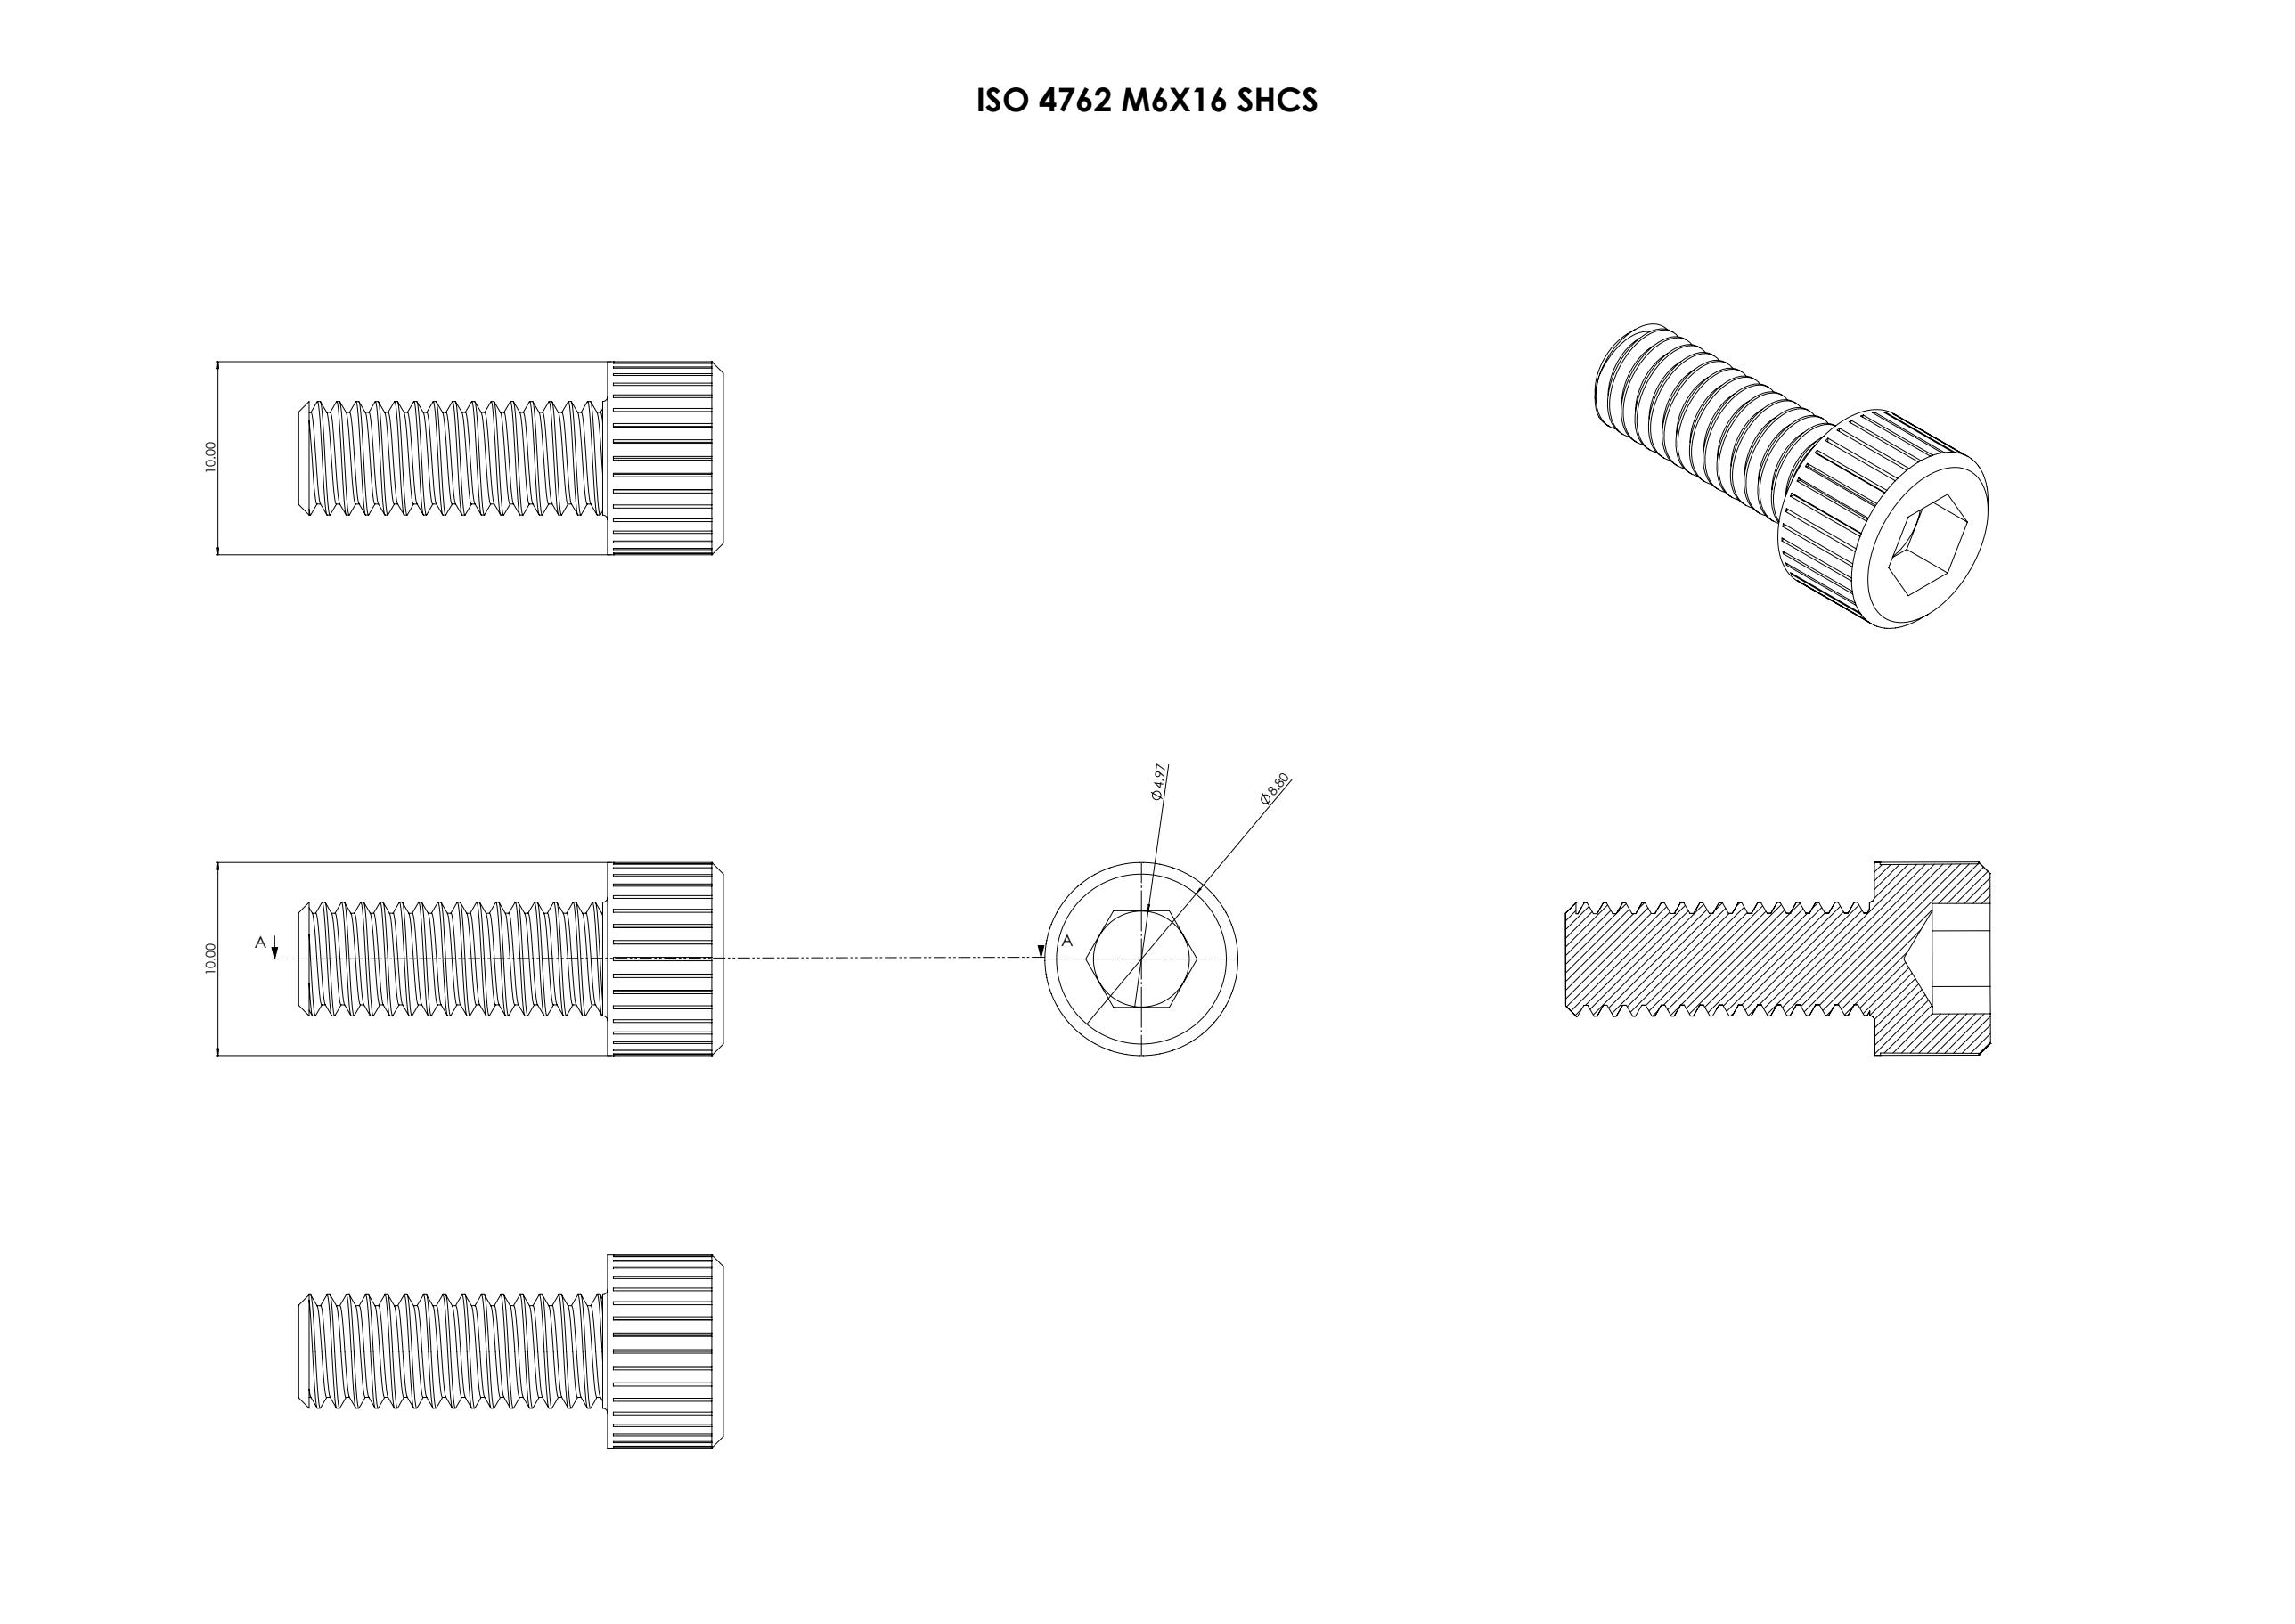
ISO-10303-21;
HEADER;
/* Generated by software containing ST-Developer
 * from STEP Tools, Inc. (www.steptools.com) 
 */

FILE_DESCRIPTION(
/* description */ (''),
/* implementation_level */ '2;1');

FILE_NAME(
/* name */ '09_ISO_4762_M6x16_SHCS.step',
/* time_stamp */ '2026-10-11T08:27:52-07:00',
/* author */ (''),
/* organization */ (''),
/* preprocessor_version */ 'ST-DEVELOPER v20.2',
/* originating_system */ 'Autodesk Translation Framework v15.15.0.0',
/* authorisation */ '');

FILE_SCHEMA (('AUTOMOTIVE_DESIGN { 1 0 10303 214 3 1 1 }'));
ENDSEC;

DATA;
#10=MECHANICAL_DESIGN_GEOMETRIC_PRESENTATION_REPRESENTATION('',(#927),#94301);
#550=B_SPLINE_CURVE_WITH_KNOTS('',3,(#87482,#87483,#87484,#87485,#87486,
#87487,#87488,#87489,#87490,#87491),.UNSPECIFIED.,.F.,.F.,(4,3,3,4),(-4.09293042013066,
-3.98462531944883,-2.98846898958662,-2.06863817490914),.UNSPECIFIED.);
#551=B_SPLINE_CURVE_WITH_KNOTS('',3,(#87494,#87495,#87496,#87497,#87498,
#87499,#87500),.UNSPECIFIED.,.F.,.F.,(4,3,4),(0.,0.996156329862199,1.11730040836818),
 .UNSPECIFIED.);
#552=B_SPLINE_CURVE_WITH_KNOTS('',3,(#87505,#87506,#87507,#87508,#87509,
#87510,#87511,#87512,#87513,#87514,#87515,#87516,#87517,#87518,#87519,#87520,
#87521,#87522,#87523,#87524,#87525,#87526),.UNSPECIFIED.,.F.,.F.,(4,3,3,
3,3,3,3,4),(-10.3761157273103,-9.96156329862207,-8.96540696875986,-7.96925063889766,
-6.97309430903545,-5.97693797917324,-4.98078164931104,-4.09293042013066),
 .UNSPECIFIED.);
#553=B_SPLINE_CURVE_WITH_KNOTS('',3,(#87527,#87528,#87529,#87530,#87531,
#87532,#87533,#87534,#87535,#87536,#87537,#87538,#87539,#87540,#87541,#87542,
#87543,#87544,#87545,#87546,#87547,#87548),.UNSPECIFIED.,.F.,.F.,(4,3,3,
3,3,3,3,4),(1.11730040836818,1.99231265972441,2.98846898958662,3.98462531944883,
4.98078164931103,5.97693797917324,6.97309430903544,7.40048571554775),
 .UNSPECIFIED.);
#554=B_SPLINE_CURVE_WITH_KNOTS('',3,(#87553,#87554,#87555,#87556,#87557,
#87558,#87559,#87560,#87561,#87562,#87563,#87564,#87565,#87566,#87567,#87568,
#87569,#87570,#87571,#87572,#87573,#87574),.UNSPECIFIED.,.F.,.F.,(4,3,3,
3,3,3,3,4),(-16.6593010344898,-15.9385012777953,-14.9423449479331,-13.9461886180709,
-12.9500322882087,-11.9538759583465,-10.9577196284843,-10.3761157273103),
 .UNSPECIFIED.);
#555=B_SPLINE_CURVE_WITH_KNOTS('',3,(#87575,#87576,#87577,#87578,#87579,
#87580,#87581,#87582,#87583,#87584,#87585,#87586,#87587,#87588,#87589,#87590,
#87591,#87592,#87593,#87594,#87595,#87596),.UNSPECIFIED.,.F.,.F.,(4,3,3,
3,3,3,3,4),(7.40048571554775,7.96925063889765,8.96540696875986,9.96156329862207,
10.9577196284843,11.9538759583465,12.9500322882087,13.6836710227273),
 .UNSPECIFIED.);
#556=B_SPLINE_CURVE_WITH_KNOTS('',3,(#87601,#87602,#87603,#87604,#87605,
#87606,#87607,#87608,#87609,#87610,#87611,#87612,#87613,#87614,#87615,#87616,
#87617,#87618,#87619,#87620,#87621,#87622,#87623,#87624,#87625),
 .UNSPECIFIED.,.F.,.F.,(4,3,3,3,3,3,3,3,4),(-22.9424863416694,-22.9115955868308,
-21.9154392569686,-20.9192829271063,-19.9231265972441,-18.9269702673819,
-17.9308139375197,-16.9346576076575,-16.6593010344898),.UNSPECIFIED.);
#557=B_SPLINE_CURVE_WITH_KNOTS('',3,(#87626,#87627,#87628,#87629,#87630,
#87631,#87632,#87633,#87634,#87635,#87636,#87637,#87638,#87639,#87640,#87641,
#87642,#87643,#87644,#87645,#87646,#87647,#87648,#87649,#87650),
 .UNSPECIFIED.,.F.,.F.,(4,3,3,3,3,3,3,3,4),(13.6836710227273,13.9461886180709,
14.9423449479331,15.9385012777953,16.9346576076575,17.9308139375197,18.9269702673819,
19.9231265972441,19.9668563299069),.UNSPECIFIED.);
#558=B_SPLINE_CURVE_WITH_KNOTS('',3,(#87655,#87656,#87657,#87658,#87659,
#87660,#87661,#87662,#87663,#87664,#87665,#87666,#87667,#87668,#87669,#87670,
#87671,#87672,#87673,#87674,#87675,#87676),.UNSPECIFIED.,.F.,.F.,(4,3,3,
3,3,3,3,4),(-29.225671648849,-28.888533566004,-27.8923772361418,-26.8962209062796,
-25.9000645764174,-24.9039082465552,-23.907751916693,-22.9424863416694),
 .UNSPECIFIED.);
#559=B_SPLINE_CURVE_WITH_KNOTS('',3,(#87677,#87678,#87679,#87680,#87681,
#87682,#87683,#87684,#87685,#87686,#87687,#87688,#87689,#87690,#87691,#87692,
#87693,#87694,#87695,#87696,#87697,#87698),.UNSPECIFIED.,.F.,.F.,(4,3,3,
3,3,3,3,4),(19.9668563299069,20.9192829271063,21.9154392569685,22.9115955868307,
23.907751916693,24.9039082465552,25.9000645764174,26.2500416370865),
 .UNSPECIFIED.);
#560=B_SPLINE_CURVE_WITH_KNOTS('',3,(#87703,#87704,#87705,#87706,#87707,
#87708,#87709,#87710,#87711,#87712,#87713,#87714,#87715,#87716,#87717,#87718,
#87719,#87720,#87721,#87722,#87723,#87724),.UNSPECIFIED.,.F.,.F.,(4,3,3,
3,3,3,3,4),(-35.5088569560286,-34.8654715451772,-33.869315215315,-32.8731588854528,
-31.8770025555906,-30.8808462257284,-29.8846898958662,-29.225671648849),
 .UNSPECIFIED.);
#561=B_SPLINE_CURVE_WITH_KNOTS('',3,(#87725,#87726,#87727,#87728,#87729,
#87730,#87731,#87732,#87733,#87734,#87735,#87736,#87737,#87738,#87739,#87740,
#87741,#87742,#87743,#87744,#87745,#87746),.UNSPECIFIED.,.F.,.F.,(4,3,3,
3,3,3,3,4),(26.2500416370865,26.8962209062796,27.8923772361418,28.888533566004,
29.8846898958662,30.8808462257284,31.8770025555906,32.5332269442661),
 .UNSPECIFIED.);
#562=B_SPLINE_CURVE_WITH_KNOTS('',3,(#87751,#87752,#87753,#87754,#87755,
#87756,#87757,#87758,#87759,#87760,#87761,#87762,#87763,#87764,#87765,#87766,
#87767,#87768,#87769,#87770,#87771,#87772),.UNSPECIFIED.,.F.,.F.,(4,3,3,
3,3,3,3,4),(-41.7920422632082,-40.8424095243505,-39.8462531944883,-38.8500968646261,
-37.8539405347639,-36.8577842049017,-35.8616278750394,-35.5088569560286),
 .UNSPECIFIED.);
#563=B_SPLINE_CURVE_WITH_KNOTS('',3,(#87773,#87774,#87775,#87776,#87777,
#87778,#87779,#87780,#87781,#87782,#87783,#87784,#87785,#87786,#87787,#87788,
#87789,#87790,#87791,#87792,#87793,#87794),.UNSPECIFIED.,.F.,.F.,(4,3,3,
3,3,3,3,4),(32.5332269442661,32.8731588854528,33.869315215315,34.8654715451772,
35.8616278750394,36.8577842049016,37.8539405347639,38.8164122514457),
 .UNSPECIFIED.);
#564=B_SPLINE_CURVE_WITH_KNOTS('',3,(#87799,#87800,#87801,#87802,#87803,
#87804,#87805,#87806,#87807,#87808,#87809,#87810,#87811,#87812,#87813,#87814,
#87815,#87816,#87817,#87818,#87819,#87820,#87821,#87822,#87823),
 .UNSPECIFIED.,.F.,.F.,(4,3,3,3,3,3,3,3,4),(-48.0752275703878,-47.8155038333859,
-46.8193475035237,-45.8231911736615,-44.8270348437993,-43.8308785139371,
-42.8347221840749,-41.8385658542127,-41.7920422632082),.UNSPECIFIED.);
#565=B_SPLINE_CURVE_WITH_KNOTS('',3,(#87824,#87825,#87826,#87827,#87828,
#87829,#87830,#87831,#87832,#87833,#87834,#87835,#87836,#87837,#87838,#87839,
#87840,#87841,#87842,#87843,#87844,#87845,#87846,#87847,#87848),
 .UNSPECIFIED.,.F.,.F.,(4,3,3,3,3,3,3,3,4),(38.8164122514457,38.8500968646261,
39.8462531944883,40.8424095243505,41.8385658542127,42.8347221840749,43.8308785139371,
44.8270348437993,45.0995975586253),.UNSPECIFIED.);
#566=B_SPLINE_CURVE_WITH_KNOTS('',3,(#87853,#87854,#87855,#87856,#87857,
#87858,#87859,#87860,#87861,#87862,#87863,#87864,#87865,#87866,#87867,#87868,
#87869,#87870,#87871,#87872,#87873,#87874),.UNSPECIFIED.,.F.,.F.,(4,3,3,
3,3,3,3,4),(-54.3584128775674,-53.7924418125592,-52.796285482697,-51.8001291528348,
-50.8039728229726,-49.8078164931104,-48.8116601632481,-48.0752275703878),
 .UNSPECIFIED.);
#567=B_SPLINE_CURVE_WITH_KNOTS('',3,(#87875,#87876,#87877,#87878,#87879,
#87880,#87881,#87882,#87883,#87884,#87885,#87886,#87887,#87888,#87889,#87890,
#87891,#87892,#87893,#87894,#87895,#87896),.UNSPECIFIED.,.F.,.F.,(4,3,3,
3,3,3,3,4),(45.0995975586253,45.8231911736615,46.8193475035237,47.8155038333859,
48.8116601632481,49.8078164931103,50.8039728229725,51.3827828658049),
 .UNSPECIFIED.);
#568=B_SPLINE_CURVE_WITH_KNOTS('',3,(#87901,#87902,#87903,#87904,#87905,
#87906,#87907,#87908,#87909,#87910,#87911,#87912,#87913,#87914,#87915,#87916,
#87917,#87918,#87919,#87920,#87921,#87922),.UNSPECIFIED.,.F.,.F.,(4,3,3,
3,3,3,3,4),(-60.641598184747,-59.7693797917324,-58.7732234618702,-57.777067132008,
-56.7809108021458,-55.7847544722836,-54.7885981424214,-54.3584128775674),
 .UNSPECIFIED.);
#569=B_SPLINE_CURVE_WITH_KNOTS('',3,(#87923,#87924,#87925,#87926,#87927,
#87928,#87929,#87930,#87931,#87932,#87933,#87934,#87935,#87936,#87937,#87938,
#87939,#87940,#87941,#87942,#87943,#87944),.UNSPECIFIED.,.F.,.F.,(4,3,3,
3,3,3,3,4),(51.3827828658049,51.8001291528347,52.796285482697,53.7924418125592,
54.7885981424214,55.7847544722836,56.7809108021458,57.6659681729845),
 .UNSPECIFIED.);
#570=B_SPLINE_CURVE_WITH_KNOTS('',3,(#87949,#87950,#87951,#87952,#87953,
#87954,#87955,#87956,#87957,#87958,#87959,#87960,#87961,#87962,#87963,#87964,
#87965,#87966,#87967,#87968,#87969,#87970,#87971,#87972,#87973),
 .UNSPECIFIED.,.F.,.F.,(4,3,3,3,3,3,3,3,4),(-66.9247834919266,-66.7424741007679,
-65.7463177709057,-64.7501614410435,-63.7540051111813,-62.757848781319,
-61.7616924514568,-60.7655361215946,-60.641598184747),.UNSPECIFIED.);
#571=B_SPLINE_CURVE_WITH_KNOTS('',3,(#87974,#87975,#87976,#87977,#87978,
#87979,#87980,#87981,#87982,#87983,#87984,#87985,#87986,#87987,#87988,#87989,
#87990,#87991,#87992,#87993,#87994,#87995,#87996,#87997,#87998),
 .UNSPECIFIED.,.F.,.F.,(4,3,3,3,3,3,3,3,4),(57.6659681729845,57.777067132008,
58.7732234618702,59.7693797917324,60.7655361215946,61.7616924514568,62.757848781319,
63.7540051111813,63.9491534801641),.UNSPECIFIED.);
#572=B_SPLINE_CURVE_WITH_KNOTS('',3,(#88003,#88004,#88005,#88006,#88007,
#88008,#88009,#88010,#88011,#88012,#88013,#88014,#88015,#88016,#88017,#88018,
#88019,#88020,#88021,#88022,#88023,#88024),.UNSPECIFIED.,.F.,.F.,(4,3,3,
3,3,3,3,4),(-73.2079687991062,-72.7194120799411,-71.7232557500789,-70.7270994202167,
-69.7309430903545,-68.7347867604923,-67.7386304306301,-66.9247834919266),
 .UNSPECIFIED.);
#573=B_SPLINE_CURVE_WITH_KNOTS('',3,(#88025,#88026,#88027,#88028,#88029,
#88030,#88031,#88032,#88033,#88034,#88035,#88036,#88037,#88038,#88039,#88040,
#88041,#88042,#88043,#88044,#88045,#88046),.UNSPECIFIED.,.F.,.F.,(4,3,3,
3,3,3,3,4),(63.9491534801641,64.7501614410435,65.7463177709057,66.7424741007679,
67.7386304306301,68.7347867604923,69.7309430903545,70.2323387873437),
 .UNSPECIFIED.);
#574=B_SPLINE_CURVE_WITH_KNOTS('',3,(#88051,#88052,#88053,#88054,#88055,
#88056,#88057,#88058,#88059,#88060,#88061,#88062,#88063,#88064,#88065,#88066,
#88067,#88068,#88069,#88070,#88071,#88072),.UNSPECIFIED.,.F.,.F.,(4,3,3,
3,3,3,3,4),(-79.4911541062857,-78.6963500591144,-77.7001937292521,-76.7040373993899,
-75.7078810695277,-74.7117247396655,-73.7155684098033,-73.2079687991062),
 .UNSPECIFIED.);
#575=B_SPLINE_CURVE_WITH_KNOTS('',3,(#88073,#88074,#88075,#88076,#88077,
#88078,#88079,#88080,#88081,#88082,#88083,#88084,#88085,#88086,#88087,#88088,
#88089,#88090,#88091,#88092,#88093,#88094),.UNSPECIFIED.,.F.,.F.,(4,3,3,
3,3,3,3,4),(70.2323387873437,70.7270994202167,71.7232557500789,72.7194120799411,
73.7155684098033,74.7117247396655,75.7078810695277,76.5155240945233),
 .UNSPECIFIED.);
#576=B_SPLINE_CURVE_WITH_KNOTS('',3,(#88099,#88100,#88101,#88102,#88103,
#88104,#88105,#88106,#88107,#88108,#88109,#88110,#88111,#88112,#88113,#88114,
#88115,#88116,#88117,#88118,#88119,#88120,#88121,#88122,#88123),
 .UNSPECIFIED.,.F.,.F.,(4,3,3,3,3,3,3,3,4),(-85.7743394134653,-85.6694443681498,
-84.6732880382876,-83.6771317084254,-82.6809753785632,-81.684819048701,
-80.6886627188388,-79.6925063889766,-79.4911541062857),.UNSPECIFIED.);
#577=B_SPLINE_CURVE_WITH_KNOTS('',3,(#88124,#88125,#88126,#88127,#88128,
#88129,#88130,#88131,#88132,#88133,#88134,#88135,#88136,#88137,#88138,#88139,
#88140,#88141,#88142,#88143,#88144,#88145,#88146,#88147,#88148),
 .UNSPECIFIED.,.F.,.F.,(4,3,3,3,3,3,3,3,4),(76.5155240945233,76.7040373993899,
77.7001937292521,78.6963500591143,79.6925063889765,80.6886627188388,81.684819048701,
82.6809753785631,82.7987094017029),.UNSPECIFIED.);
#578=B_SPLINE_CURVE_WITH_KNOTS('',3,(#88153,#88154,#88155,#88156,#88157,
#88158,#88159,#88160,#88161,#88162,#88163,#88164,#88165,#88166,#88167,#88168,
#88169,#88170,#88171,#88172,#88173,#88174),.UNSPECIFIED.,.F.,.F.,(4,3,3,
3,3,3,3,4),(-92.0575247206449,-91.646382347323,-90.6502260174608,-89.6540696875986,
-88.6579133577364,-87.6617570278742,-86.665600698012,-85.7743394134653),
 .UNSPECIFIED.);
#579=B_SPLINE_CURVE_WITH_KNOTS('',3,(#88175,#88176,#88177,#88178,#88179,
#88180,#88181,#88182,#88183,#88184,#88185,#88186,#88187,#88188,#88189,#88190,
#88191,#88192,#88193,#88194,#88195,#88196),.UNSPECIFIED.,.F.,.F.,(4,3,3,
3,3,3,3,4),(82.7987094017029,83.6771317084254,84.6732880382876,85.6694443681498,
86.665600698012,87.6617570278742,88.6579133577364,89.0818947088824),
 .UNSPECIFIED.);
#580=B_SPLINE_CURVE_WITH_KNOTS('',3,(#88203,#88204,#88205,#88206,#88207,
#88208,#88209,#88210,#88211,#88212,#88213,#88214,#88215,#88216,#88217,#88218,
#88219,#88220,#88221),.UNSPECIFIED.,.F.,.F.,(4,3,3,3,3,3,4),(-97.6233203264963,
-96.6271639966341,-95.6310076667719,-94.6348513369097,-93.6386950070474,
-92.6425386771852,-92.0575247206449),.UNSPECIFIED.);
#581=B_SPLINE_CURVE_WITH_KNOTS('',3,(#88222,#88223,#88224,#88225,#88226,
#88227,#88228,#88229,#88230,#88231,#88232,#88233,#88234,#88235,#88236,#88237,
#88238,#88239,#88240,#88241,#88242,#88243),.UNSPECIFIED.,.F.,.F.,(4,3,3,
3,3,3,3,4),(89.0818947088824,89.6540696875986,90.6502260174608,91.646382347323,
92.6425386771852,93.6386950070475,94.6348513369096,95.365080016062),
 .UNSPECIFIED.);
#582=B_SPLINE_CURVE_WITH_KNOTS('',3,(#88249,#88250,#88251,#88252,#88253,
#88254,#88255),.UNSPECIFIED.,.F.,.F.,(4,1,1,1,4),(103.672557568463,104.257571525003,
105.253727854866,106.249884184728,107.169714999405),.UNSPECIFIED.);
#583=B_SPLINE_CURVE_WITH_KNOTS('',3,(#88258,#88259,#88260,#88261,#88262,
#88263),.UNSPECIFIED.,.F.,.F.,(4,1,1,4),(103.672557568463,103.938485219173,
104.934641549035,105.930797878897),.UNSPECIFIED.);
#584=B_SPLINE_CURVE_WITH_KNOTS('',3,(#88268,#88269,#88270,#88271,#88272,
#88273,#88274,#88275,#88276,#88277),.UNSPECIFIED.,.F.,.F.,(4,1,1,1,1,1,
1,4),(97.3893722612836,98.2806335458302,99.2767898756924,100.272946205555,
101.269102535417,102.265258865279,103.261415195141,103.672557568463),
 .UNSPECIFIED.);
#585=B_SPLINE_CURVE_WITH_KNOTS('',3,(#88278,#88279,#88280,#88281,#88282,
#88283,#88284,#88285,#88286,#88287),.UNSPECIFIED.,.F.,.F.,(4,1,1,1,1,1,
1,4),(97.3893722612836,97.9615472399996,98.9577035698618,99.9538598997241,
100.950016229586,101.946172559448,102.942328889311,103.672557568463),
 .UNSPECIFIED.);
#586=B_SPLINE_CURVE_WITH_KNOTS('',3,(#88292,#88293,#88294,#88295,#88296,
#88297,#88298,#88299,#88300,#88301,#88302),.UNSPECIFIED.,.F.,.F.,(4,1,1,
1,1,1,1,1,4),(91.106186954104,91.3075392367948,92.303695566657,93.2998518965192,
94.2960082263814,95.2921645562436,96.2883208861058,97.284477215968,97.3893722612836),
 .UNSPECIFIED.);
#587=B_SPLINE_CURVE_WITH_KNOTS('',3,(#88303,#88304,#88305,#88306,#88307,
#88308,#88309,#88310,#88311,#88312),.UNSPECIFIED.,.F.,.F.,(4,1,1,1,1,1,
1,4),(91.106186954104,91.9846092608264,92.9807655906886,93.9769219205508,
94.973078250413,95.9692345802752,96.9653909101374,97.3893722612836),
 .UNSPECIFIED.);
#588=B_SPLINE_CURVE_WITH_KNOTS('',3,(#88317,#88318,#88319,#88320,#88321,
#88322,#88323,#88324,#88325,#88326),.UNSPECIFIED.,.F.,.F.,(4,1,1,1,1,1,
1,4),(84.8230016469244,85.3306012576215,86.3267575874837,87.322913917346,
88.3190702472082,89.3152265770704,90.3113829069326,91.106186954104),
 .UNSPECIFIED.);
#589=B_SPLINE_CURVE_WITH_KNOTS('',3,(#88327,#88328,#88329,#88330,#88331,
#88332,#88333,#88334,#88335,#88336,#88337),.UNSPECIFIED.,.F.,.F.,(4,1,1,
1,1,1,1,1,4),(84.8230016469244,85.0115149517909,86.0076712816532,87.0038276115154,
87.9999839413776,88.9961402712398,89.992296601102,90.9884529309642,91.106186954104),
 .UNSPECIFIED.);
#590=B_SPLINE_CURVE_WITH_KNOTS('',3,(#88342,#88343,#88344,#88345,#88346,
#88347,#88348,#88349,#88350,#88351),.UNSPECIFIED.,.F.,.F.,(4,1,1,1,1,1,
1,4),(78.5398163397448,79.3536632784483,80.3498196083105,81.3459759381727,
82.3421322680349,83.3382885978971,84.3344449277593,84.8230016469244),
 .UNSPECIFIED.);
#591=B_SPLINE_CURVE_WITH_KNOTS('',3,(#88352,#88353,#88354,#88355,#88356,
#88357,#88358,#88359,#88360,#88361),.UNSPECIFIED.,.F.,.F.,(4,1,1,1,1,1,
1,4),(78.5398163397448,79.0345769726177,80.0307333024799,81.0268896323421,
82.0230459622043,83.0192022920665,84.0153586219287,84.8230016469244),
 .UNSPECIFIED.);
#592=B_SPLINE_CURVE_WITH_KNOTS('',3,(#88366,#88367,#88368,#88369,#88370,
#88371,#88372,#88373,#88374,#88375,#88376),.UNSPECIFIED.,.F.,.F.,(4,1,1,
1,1,1,1,1,4),(72.2566310325652,72.3805689694128,73.3767252992751,74.3728816291373,
75.3690379589995,76.3651942888617,77.3613506187239,78.3575069485861,78.5398163397448),
 .UNSPECIFIED.);
#593=B_SPLINE_CURVE_WITH_KNOTS('',3,(#88377,#88378,#88379,#88380,#88381,
#88382,#88383,#88384,#88385,#88386),.UNSPECIFIED.,.F.,.F.,(4,1,1,1,1,1,
1,4),(72.2566310325652,73.0576389934445,74.0537953233067,75.0499516531689,
76.0461079830311,77.0422643128933,78.0384206427555,78.5398163397448),
 .UNSPECIFIED.);
#594=B_SPLINE_CURVE_WITH_KNOTS('',3,(#88391,#88392,#88393,#88394,#88395,
#88396,#88397,#88398,#88399,#88400),.UNSPECIFIED.,.F.,.F.,(4,1,1,1,1,1,
1,4),(65.9734457253856,66.4036309902396,67.3997873201018,68.395943649964,
69.3920999798262,70.3882563096884,71.3844126395506,72.2566310325652),
 .UNSPECIFIED.);
#595=B_SPLINE_CURVE_WITH_KNOTS('',3,(#88401,#88402,#88403,#88404,#88405,
#88406,#88407,#88408,#88409,#88410,#88411),.UNSPECIFIED.,.F.,.F.,(4,1,1,
1,1,1,1,1,4),(65.9734457253856,66.084544684409,67.0807010142712,68.0768573441334,
69.0730136739956,70.0691700038578,71.0653263337201,72.0614826635823,72.2566310325652),
 .UNSPECIFIED.);
#596=B_SPLINE_CURVE_WITH_KNOTS('',3,(#88416,#88417,#88418,#88419,#88420,
#88421,#88422,#88423,#88424,#88425),.UNSPECIFIED.,.F.,.F.,(4,1,1,1,1,1,
1,4),(59.690260418206,60.4266930110664,61.4228493409286,62.4190056707908,
63.415162000653,64.4113183305152,65.4074746603774,65.9734457253856),
 .UNSPECIFIED.);
#597=B_SPLINE_CURVE_WITH_KNOTS('',3,(#88426,#88427,#88428,#88429,#88430,
#88431,#88432,#88433,#88434,#88435),.UNSPECIFIED.,.F.,.F.,(4,1,1,1,1,1,
1,4),(59.690260418206,60.1076067052358,61.103763035098,62.0999193649602,
63.0960756948224,64.0922320246846,65.0883883545468,65.9734457253856),
 .UNSPECIFIED.);
#598=B_SPLINE_CURVE_WITH_KNOTS('',3,(#88440,#88441,#88442,#88443,#88444,
#88445,#88446,#88447,#88448,#88449,#88450),.UNSPECIFIED.,.F.,.F.,(4,1,1,
1,1,1,1,1,4),(53.4070751110264,53.4535987020309,54.4497550318931,55.4459113617553,
56.4420676916175,57.4382240214797,58.434380351342,59.4305366812042,59.690260418206),
 .UNSPECIFIED.);
#599=B_SPLINE_CURVE_WITH_KNOTS('',3,(#88451,#88452,#88453,#88454,#88455,
#88456,#88457,#88458,#88459,#88460),.UNSPECIFIED.,.F.,.F.,(4,1,1,1,1,1,
1,4),(53.4070751110264,54.1306687260625,55.1268250559247,56.122981385787,
57.1191377156492,58.1152940455114,59.1114503753736,59.690260418206),
 .UNSPECIFIED.);
#600=B_SPLINE_CURVE_WITH_KNOTS('',3,(#88465,#88466,#88467,#88468,#88469,
#88470,#88471,#88472,#88473,#88474),.UNSPECIFIED.,.F.,.F.,(4,1,1,1,1,1,
1,4),(47.1238898038468,47.4766607228577,48.4728170527199,49.4689733825821,
50.4651297124443,51.4612860423065,52.4574423721687,53.4070751110264),
 .UNSPECIFIED.);
#601=B_SPLINE_CURVE_WITH_KNOTS('',3,(#88475,#88476,#88477,#88478,#88479,
#88480,#88481,#88482,#88483,#88484,#88485),.UNSPECIFIED.,.F.,.F.,(4,1,1,
1,1,1,1,1,4),(47.1238898038468,47.1575744170271,48.1537307468893,49.1498870767515,
50.1460434066137,51.1421997364759,52.1383560663381,53.1345123962003,53.4070751110264),
 .UNSPECIFIED.);
#602=B_SPLINE_CURVE_WITH_KNOTS('',3,(#88490,#88491,#88492,#88493,#88494,
#88495,#88496,#88497,#88498,#88499),.UNSPECIFIED.,.F.,.F.,(4,1,1,1,1,1,
1,4),(40.8407044966673,41.4997227436844,42.4958790735466,43.4920354034088,
44.4881917332711,45.4843480631333,46.4805043929955,47.1238898038468),
 .UNSPECIFIED.);
#603=B_SPLINE_CURVE_WITH_KNOTS('',3,(#88500,#88501,#88502,#88503,#88504,
#88505,#88506,#88507,#88508,#88509),.UNSPECIFIED.,.F.,.F.,(4,1,1,1,1,1,
1,4),(40.8407044966672,41.1806364378538,42.1767927677161,43.1729490975783,
44.1691054274405,45.1652617573027,46.1614180871649,47.1238898038468),
 .UNSPECIFIED.);
#604=B_SPLINE_CURVE_WITH_KNOTS('',3,(#88514,#88515,#88516,#88517,#88518,
#88519,#88520,#88521,#88522,#88523),.UNSPECIFIED.,.F.,.F.,(4,1,1,1,1,1,
1,4),(34.5575191894877,35.5227847645112,36.5189410943734,37.5150974242356,
38.5112537540978,39.50741008396,40.5035664138222,40.8407044966673),
 .UNSPECIFIED.);
#605=B_SPLINE_CURVE_WITH_KNOTS('',3,(#88524,#88525,#88526,#88527,#88528,
#88529,#88530,#88531,#88532,#88533),.UNSPECIFIED.,.F.,.F.,(4,1,1,1,1,1,
1,4),(34.5575191894876,35.2036984586806,36.1998547885428,37.196011118405,
38.1921674482672,39.1883237781294,40.1844801079916,40.8407044966672),
 .UNSPECIFIED.);
#606=B_SPLINE_CURVE_WITH_KNOTS('',3,(#88538,#88539,#88540,#88541,#88542,
#88543,#88544,#88545,#88546,#88547,#88548),.UNSPECIFIED.,.F.,.F.,(4,1,1,
1,1,1,1,1,4),(28.2743338823081,28.5496904554757,29.545846785338,30.5420031152002,
31.5381594450624,32.5343157749246,33.5304721047868,34.526628434649,34.5575191894877),
 .UNSPECIFIED.);
#607=B_SPLINE_CURVE_WITH_KNOTS('',3,(#88549,#88550,#88551,#88552,#88553,
#88554,#88555,#88556,#88557,#88558),.UNSPECIFIED.,.F.,.F.,(4,1,1,1,1,1,
1,4),(28.2743338823081,29.2267604795074,30.2229168093696,31.2190731392318,
32.215229469094,33.2113857989562,34.2075421288184,34.5575191894876),
 .UNSPECIFIED.);
#608=B_SPLINE_CURVE_WITH_KNOTS('',3,(#88563,#88564,#88565,#88566,#88567,
#88568,#88569,#88570,#88571,#88572),.UNSPECIFIED.,.F.,.F.,(4,1,1,1,1,1,
1,4),(21.9911485751285,22.5727524763025,23.5689088061647,24.5650651360269,
25.5612214658891,26.5573777957513,27.5535341256135,28.2743338823081),
 .UNSPECIFIED.);
#609=B_SPLINE_CURVE_WITH_KNOTS('',3,(#88573,#88574,#88575,#88576,#88577,
#88578,#88579,#88580,#88581,#88582,#88583),.UNSPECIFIED.,.F.,.F.,(4,1,1,
1,1,1,1,1,4),(21.9911485751285,22.2536661704719,23.2498225003341,24.2459788301963,
25.2421351600585,26.2382914899207,27.234447819783,28.2306041496452,28.2743338823081),
 .UNSPECIFIED.);
#610=B_SPLINE_CURVE_WITH_KNOTS('',3,(#88588,#88589,#88590,#88591,#88592,
#88593,#88594,#88595,#88596,#88597),.UNSPECIFIED.,.F.,.F.,(4,1,1,1,1,1,
1,4),(15.7079632679489,16.5958144971293,17.5919708269915,18.5881271568537,
19.5842834867159,20.5804398165781,21.5765961464403,21.9911485751285),
 .UNSPECIFIED.);
#611=B_SPLINE_CURVE_WITH_KNOTS('',3,(#88598,#88599,#88600,#88601,#88602,
#88603,#88604,#88605,#88606,#88607),.UNSPECIFIED.,.F.,.F.,(4,1,1,1,1,1,
1,4),(15.7079632679489,16.2767281912987,17.2728845211609,18.2690408510231,
19.2651971808853,20.2613535107475,21.2575098406097,21.9911485751285),
 .UNSPECIFIED.);
#612=B_SPLINE_CURVE_WITH_KNOTS('',3,(#88609,#88610,#88611,#88612,#88613,
#88614,#88615,#88616,#88617,#88618,#88619,#88620,#88621,#88622,#88623,#88624,
#88625,#88626,#88627,#88628,#88629,#88630,#88631,#88632,#88633,#88634,#88635,
#88636,#88637,#88638,#88639,#88640,#88641,#88642,#88643,#88644,#88645,#88646,
#88647,#88648,#88649,#88650,#88651,#88652,#88653,#88654,#88655,#88656,#88657,
#88658,#88659,#88660,#88661,#88662,#88663,#88664,#88665,#88666,#88667,#88668,
#88669,#88670,#88671,#88672,#88673,#88674,#88675,#88676,#88677,#88678,#88679,
#88680,#88681,#88682,#88683,#88684,#88685,#88686,#88687,#88688,#88689,#88690,
#88691,#88692,#88693,#88694,#88695,#88696,#88697,#88698,#88699),
 .UNSPECIFIED.,.F.,.F.,(4,3,3,3,3,3,3,3,3,3,3,3,3,3,3,3,3,3,3,3,3,3,3,3,
3,3,3,3,3,3,4),(-0.555272788399387,-0.536878011109327,-0.51216130922638,
-0.497772596378623,-0.492151132384111,-0.487788613626176,-0.462008896459435,
-0.439500522359789,-0.428647464230627,-0.422031983310641,-0.395447331110844,
-0.367070974248699,-0.34578870660209,-0.329827005867133,-0.325388458044637,
-0.321109090061203,-0.293193723306362,-0.281941903662263,-0.254996262835833,
-0.227510620629366,-0.221955374106226,-0.217785459312042,-0.189854551496702,
-0.161379875371563,-0.132653453208679,-0.116071771557594,-0.111842840924105,
-0.082388957527505,-0.052837079875276,-0.0238339308196913,0.),
 .UNSPECIFIED.);
#613=B_SPLINE_CURVE_WITH_KNOTS('',3,(#88704,#88705,#88706,#88707,#88708,
#88709,#88710,#88711,#88712,#88713,#88714,#88715,#88716,#88717,#88718,#88719,
#88720,#88721,#88722,#88723,#88724,#88725,#88726,#88727,#88728,#88729,#88730,
#88731,#88732,#88733,#88734,#88735,#88736,#88737,#88738,#88739,#88740,#88741,
#88742,#88743,#88744,#88745,#88746,#88747,#88748,#88749,#88750,#88751,#88752,
#88753,#88754,#88755,#88756,#88757,#88758,#88759,#88760,#88761,#88762,#88763,
#88764,#88765,#88766,#88767,#88768,#88769,#88770,#88771,#88772,#88773,#88774,
#88775,#88776,#88777,#88778,#88779,#88780,#88781,#88782,#88783,#88784,#88785,
#88786,#88787,#88788,#88789,#88790,#88791,#88792,#88793,#88794,#88795,#88796,
#88797),.UNSPECIFIED.,.F.,.F.,(4,3,3,3,3,3,3,3,3,3,3,3,3,3,3,3,3,3,3,3,
3,3,3,3,3,3,3,3,3,3,3,4),(-0.552745378375053,-0.530338827917477,-0.500953818352793,
-0.485391213597782,-0.477022768561509,-0.471909598051007,-0.44285760577117,
-0.418994422833851,-0.408389712365122,-0.402041246675515,-0.397478427204802,
-0.369171225298371,-0.339866454541933,-0.31274605694021,-0.296909993024151,
-0.291443327397581,-0.264638986575274,-0.251952142272617,-0.224584144938619,
-0.196511126821292,-0.192477354107935,-0.188234651713186,-0.161595549194534,
-0.134996331746453,-0.108821820380775,-0.0998778564626278,-0.0942964343013907,
-0.0901979491855338,-0.0646528926729606,-0.0395090521317962,-0.0151488290738175,
0.),.UNSPECIFIED.);
#614=B_SPLINE_CURVE_WITH_KNOTS('',3,(#89202,#89203,#89204,#89205),
 .UNSPECIFIED.,.F.,.F.,(4,4),(95.365080016062,95.5546821515871),
 .UNSPECIFIED.);
#615=B_SPLINE_CURVE_WITH_KNOTS('',3,(#89207,#89208,#89209,#89210,#89211,
#89212,#89213,#89214,#89215,#89216,#89217,#89218,#89219,#89220,#89221,#89222,
#89223,#89224,#89225,#89226,#89227,#89228,#89229,#89230,#89231,#89232,#89233,
#89234,#89235,#89236,#89237,#89238,#89239,#89240,#89241,#89242,#89243,#89244,
#89245,#89246,#89247,#89248,#89249,#89250,#89251,#89252,#89253,#89254,#89255,
#89256,#89257,#89258,#89259,#89260,#89261,#89262,#89263,#89264,#89265,#89266,
#89267,#89268,#89269,#89270,#89271,#89272,#89273,#89274,#89275,#89276,#89277,
#89278,#89279,#89280,#89281,#89282,#89283,#89284,#89285,#89286,#89287,#89288,
#89289,#89290,#89291,#89292,#89293,#89294,#89295,#89296,#89297),
 .UNSPECIFIED.,.F.,.F.,(4,3,3,3,3,3,3,3,3,3,3,3,3,3,3,3,3,3,3,3,3,3,3,3,
3,3,3,3,3,3,4),(-0.555272788399382,-0.536878011109318,-0.512161326342915,
-0.497772612425373,-0.492151154968866,-0.487788650423359,-0.462008945431106,
-0.43950056521,-0.42864753175858,-0.422031972845274,-0.395447329416593,
-0.367070972978008,-0.34578870564907,-0.329827005152366,-0.325388447497642,
-0.3211090901766,-0.293193722617674,-0.281941903662254,-0.254996269333342,
-0.227510635185161,-0.221955302854236,-0.217785398797394,-0.189854497259803,
-0.161379828090615,-0.132653408275648,-0.116071732241192,-0.111842820088624,
-0.082388941995823,-0.0528370621263981,-0.0238338935438655,0.),
 .UNSPECIFIED.);
#616=B_SPLINE_CURVE_WITH_KNOTS('',3,(#89298,#89299,#89300,#89301,#89302,
#89303,#89304,#89305,#89306),.UNSPECIFIED.,.F.,.F.,(4,1,1,1,1,1,4),(10.3761157273101,
11.2959465419876,12.2921028718499,13.2882592017121,14.2844155315743,15.2805718614365,
15.7079632679489),.UNSPECIFIED.);
#617=B_SPLINE_CURVE_WITH_KNOTS('',3,(#89312,#89313,#89314,#89315,#89316,
#89317,#89318,#89319,#89320,#89321,#89322,#89323,#89324,#89325,#89326,#89327,
#89328,#89329,#89330,#89331,#89332,#89333,#89334,#89335,#89336,#89337,#89338,
#89339,#89340,#89341,#89342,#89343,#89344,#89345,#89346,#89347,#89348,#89349,
#89350,#89351,#89352,#89353,#89354,#89355,#89356,#89357,#89358,#89359,#89360,
#89361,#89362,#89363,#89364,#89365,#89366,#89367,#89368,#89369,#89370,#89371,
#89372,#89373,#89374,#89375,#89376,#89377,#89378,#89379,#89380,#89381,#89382,
#89383,#89384,#89385,#89386,#89387,#89388,#89389,#89390,#89391,#89392,#89393,
#89394,#89395,#89396,#89397,#89398,#89399,#89400,#89401,#89402,#89403,#89404,
#89405),.UNSPECIFIED.,.F.,.F.,(4,3,3,3,3,3,3,3,3,3,3,3,3,3,3,3,3,3,3,3,
3,3,3,3,3,3,3,3,3,3,3,4),(-0.552745378375037,-0.530338827917459,-0.500953817808515,
-0.485391213087521,-0.477022760402337,-0.471909587137758,-0.442857594671736,
-0.418994413121844,-0.408389707498453,-0.402041225045699,-0.397478412365188,
-0.36917120902983,-0.339866442340524,-0.312746024644426,-0.296909938382682,
-0.291443325001991,-0.264638969851884,-0.251952142272605,-0.224584135800549,
-0.19651111882548,-0.192477332906104,-0.188234649643676,-0.161595542748898,
-0.134996333495264,-0.108821841443691,-0.0998779134716403,-0.0942962236814242,
-0.0901979154241252,-0.0646528744752608,-0.0395090567028245,-0.0151488617676011,
0.),.UNSPECIFIED.);
#618=B_SPLINE_CURVE_WITH_KNOTS('',3,(#89408,#89409,#89410,#89411,#89412,
#89413,#89414,#89415),.UNSPECIFIED.,.F.,.F.,(4,1,1,1,1,4),(11.6150328478182,
12.6111891776804,13.6073455075426,14.6035018374048,15.5996581672671,15.7079632679489),
 .UNSPECIFIED.);
#887=B_SPLINE_SURFACE_WITH_KNOTS('',3,3,((#88798,#88799,#88800,#88801,#88802,
#88803,#88804,#88805,#88806,#88807,#88808,#88809,#88810,#88811,#88812,#88813,
#88814,#88815,#88816,#88817,#88818,#88819,#88820,#88821,#88822,#88823,#88824,
#88825,#88826,#88827,#88828,#88829,#88830,#88831,#88832,#88833,#88834,#88835,
#88836,#88837,#88838,#88839,#88840,#88841,#88842,#88843,#88844,#88845,#88846,
#88847,#88848,#88849,#88850,#88851,#88852,#88853,#88854,#88855,#88856,#88857,
#88858,#88859,#88860,#88861,#88862,#88863,#88864,#88865,#88866,#88867,#88868,
#88869,#88870,#88871,#88872,#88873,#88874,#88875,#88876,#88877,#88878,#88879,
#88880,#88881,#88882,#88883,#88884,#88885,#88886,#88887,#88888,#88889,#88890,
#88891,#88892,#88893,#88894,#88895,#88896,#88897,#88898),(#88899,#88900,
#88901,#88902,#88903,#88904,#88905,#88906,#88907,#88908,#88909,#88910,#88911,
#88912,#88913,#88914,#88915,#88916,#88917,#88918,#88919,#88920,#88921,#88922,
#88923,#88924,#88925,#88926,#88927,#88928,#88929,#88930,#88931,#88932,#88933,
#88934,#88935,#88936,#88937,#88938,#88939,#88940,#88941,#88942,#88943,#88944,
#88945,#88946,#88947,#88948,#88949,#88950,#88951,#88952,#88953,#88954,#88955,
#88956,#88957,#88958,#88959,#88960,#88961,#88962,#88963,#88964,#88965,#88966,
#88967,#88968,#88969,#88970,#88971,#88972,#88973,#88974,#88975,#88976,#88977,
#88978,#88979,#88980,#88981,#88982,#88983,#88984,#88985,#88986,#88987,#88988,
#88989,#88990,#88991,#88992,#88993,#88994,#88995,#88996,#88997,#88998,#88999),
(#89000,#89001,#89002,#89003,#89004,#89005,#89006,#89007,#89008,#89009,
#89010,#89011,#89012,#89013,#89014,#89015,#89016,#89017,#89018,#89019,#89020,
#89021,#89022,#89023,#89024,#89025,#89026,#89027,#89028,#89029,#89030,#89031,
#89032,#89033,#89034,#89035,#89036,#89037,#89038,#89039,#89040,#89041,#89042,
#89043,#89044,#89045,#89046,#89047,#89048,#89049,#89050,#89051,#89052,#89053,
#89054,#89055,#89056,#89057,#89058,#89059,#89060,#89061,#89062,#89063,#89064,
#89065,#89066,#89067,#89068,#89069,#89070,#89071,#89072,#89073,#89074,#89075,
#89076,#89077,#89078,#89079,#89080,#89081,#89082,#89083,#89084,#89085,#89086,
#89087,#89088,#89089,#89090,#89091,#89092,#89093,#89094,#89095,#89096,#89097,
#89098,#89099,#89100),(#89101,#89102,#89103,#89104,#89105,#89106,#89107,
#89108,#89109,#89110,#89111,#89112,#89113,#89114,#89115,#89116,#89117,#89118,
#89119,#89120,#89121,#89122,#89123,#89124,#89125,#89126,#89127,#89128,#89129,
#89130,#89131,#89132,#89133,#89134,#89135,#89136,#89137,#89138,#89139,#89140,
#89141,#89142,#89143,#89144,#89145,#89146,#89147,#89148,#89149,#89150,#89151,
#89152,#89153,#89154,#89155,#89156,#89157,#89158,#89159,#89160,#89161,#89162,
#89163,#89164,#89165,#89166,#89167,#89168,#89169,#89170,#89171,#89172,#89173,
#89174,#89175,#89176,#89177,#89178,#89179,#89180,#89181,#89182,#89183,#89184,
#89185,#89186,#89187,#89188,#89189,#89190,#89191,#89192,#89193,#89194,#89195,
#89196,#89197,#89198,#89199,#89200,#89201)),.UNSPECIFIED.,.F.,.F.,.F.,(4,
4),(4,1,1,1,1,1,1,1,1,1,1,1,1,1,1,1,1,1,1,1,1,1,1,1,1,1,1,1,1,1,1,1,1,1,
1,1,1,1,1,1,1,1,1,1,1,1,1,1,1,1,1,1,1,1,1,1,1,1,1,1,1,1,1,1,1,1,1,1,1,1,
1,1,1,1,1,1,1,1,1,1,1,1,1,1,1,1,1,1,1,1,1,1,1,1,1,1,1,1,4),(0.,0.0658467982010768),
(8.30747755240103,9.30363388226323,10.2997902121254,11.2959465419876,12.2921028718499,
13.2882592017121,14.2844155315743,15.2805718614365,16.2767281912987,17.2728845211609,
18.2690408510231,19.2651971808853,20.2613535107475,21.2575098406097,22.2536661704719,
23.2498225003341,24.2459788301963,25.2421351600585,26.2382914899207,27.234447819783,
28.2306041496452,29.2267604795074,30.2229168093696,31.2190731392318,32.215229469094,
33.2113857989562,34.2075421288184,35.2036984586806,36.1998547885428,37.196011118405,
38.1921674482672,39.1883237781294,40.1844801079916,41.1806364378538,42.1767927677161,
43.1729490975783,44.1691054274405,45.1652617573027,46.1614180871649,47.1575744170271,
48.1537307468893,49.1498870767515,50.1460434066137,51.1421997364759,52.1383560663381,
53.1345123962003,54.1306687260625,55.1268250559247,56.122981385787,57.1191377156492,
58.1152940455114,59.1114503753736,60.1076067052358,61.103763035098,62.0999193649602,
63.0960756948224,64.0922320246846,65.0883883545468,66.084544684409,67.0807010142712,
68.0768573441334,69.0730136739956,70.0691700038578,71.0653263337201,72.0614826635823,
73.0576389934445,74.0537953233067,75.0499516531689,76.0461079830311,77.0422643128933,
78.0384206427555,79.0345769726177,80.0307333024799,81.0268896323421,82.0230459622043,
83.0192022920665,84.0153586219287,85.0115149517909,86.0076712816532,87.0038276115154,
87.9999839413776,88.9961402712398,89.992296601102,90.9884529309642,91.9846092608264,
92.9807655906886,93.9769219205508,94.973078250413,95.9692345802752,96.9653909101374,
97.9615472399996,98.9577035698618,99.9538598997241,100.950016229586,101.946172559448,
102.942328889311,103.938485219173,104.934641549035,105.930797878897),
 .UNSPECIFIED.);
#888=B_SPLINE_SURFACE_WITH_KNOTS('',3,3,((#89416,#89417,#89418,#89419,#89420,
#89421,#89422,#89423,#89424,#89425,#89426,#89427,#89428,#89429,#89430,#89431,
#89432,#89433,#89434,#89435,#89436,#89437,#89438,#89439,#89440,#89441,#89442,
#89443,#89444,#89445,#89446,#89447,#89448,#89449,#89450,#89451,#89452,#89453,
#89454,#89455,#89456,#89457,#89458,#89459,#89460,#89461,#89462,#89463,#89464,
#89465,#89466,#89467,#89468,#89469,#89470,#89471,#89472,#89473,#89474,#89475,
#89476,#89477,#89478,#89479,#89480,#89481,#89482,#89483,#89484,#89485,#89486,
#89487,#89488,#89489,#89490,#89491,#89492,#89493,#89494,#89495,#89496,#89497,
#89498,#89499,#89500,#89501,#89502,#89503,#89504,#89505,#89506,#89507,#89508,
#89509,#89510,#89511,#89512,#89513,#89514,#89515,#89516),(#89517,#89518,
#89519,#89520,#89521,#89522,#89523,#89524,#89525,#89526,#89527,#89528,#89529,
#89530,#89531,#89532,#89533,#89534,#89535,#89536,#89537,#89538,#89539,#89540,
#89541,#89542,#89543,#89544,#89545,#89546,#89547,#89548,#89549,#89550,#89551,
#89552,#89553,#89554,#89555,#89556,#89557,#89558,#89559,#89560,#89561,#89562,
#89563,#89564,#89565,#89566,#89567,#89568,#89569,#89570,#89571,#89572,#89573,
#89574,#89575,#89576,#89577,#89578,#89579,#89580,#89581,#89582,#89583,#89584,
#89585,#89586,#89587,#89588,#89589,#89590,#89591,#89592,#89593,#89594,#89595,
#89596,#89597,#89598,#89599,#89600,#89601,#89602,#89603,#89604,#89605,#89606,
#89607,#89608,#89609,#89610,#89611,#89612,#89613,#89614,#89615,#89616,#89617),
(#89618,#89619,#89620,#89621,#89622,#89623,#89624,#89625,#89626,#89627,
#89628,#89629,#89630,#89631,#89632,#89633,#89634,#89635,#89636,#89637,#89638,
#89639,#89640,#89641,#89642,#89643,#89644,#89645,#89646,#89647,#89648,#89649,
#89650,#89651,#89652,#89653,#89654,#89655,#89656,#89657,#89658,#89659,#89660,
#89661,#89662,#89663,#89664,#89665,#89666,#89667,#89668,#89669,#89670,#89671,
#89672,#89673,#89674,#89675,#89676,#89677,#89678,#89679,#89680,#89681,#89682,
#89683,#89684,#89685,#89686,#89687,#89688,#89689,#89690,#89691,#89692,#89693,
#89694,#89695,#89696,#89697,#89698,#89699,#89700,#89701,#89702,#89703,#89704,
#89705,#89706,#89707,#89708,#89709,#89710,#89711,#89712,#89713,#89714,#89715,
#89716,#89717,#89718),(#89719,#89720,#89721,#89722,#89723,#89724,#89725,
#89726,#89727,#89728,#89729,#89730,#89731,#89732,#89733,#89734,#89735,#89736,
#89737,#89738,#89739,#89740,#89741,#89742,#89743,#89744,#89745,#89746,#89747,
#89748,#89749,#89750,#89751,#89752,#89753,#89754,#89755,#89756,#89757,#89758,
#89759,#89760,#89761,#89762,#89763,#89764,#89765,#89766,#89767,#89768,#89769,
#89770,#89771,#89772,#89773,#89774,#89775,#89776,#89777,#89778,#89779,#89780,
#89781,#89782,#89783,#89784,#89785,#89786,#89787,#89788,#89789,#89790,#89791,
#89792,#89793,#89794,#89795,#89796,#89797,#89798,#89799,#89800,#89801,#89802,
#89803,#89804,#89805,#89806,#89807,#89808,#89809,#89810,#89811,#89812,#89813,
#89814,#89815,#89816,#89817,#89818,#89819)),.UNSPECIFIED.,.F.,.F.,.F.,(4,
4),(4,1,1,1,1,1,1,1,1,1,1,1,1,1,1,1,1,1,1,1,1,1,1,1,1,1,1,1,1,1,1,1,1,1,
1,1,1,1,1,1,1,1,1,1,1,1,1,1,1,1,1,1,1,1,1,1,1,1,1,1,1,1,1,1,1,1,1,1,1,1,
1,1,1,1,1,1,1,1,1,1,1,1,1,1,1,1,1,1,1,1,1,1,1,1,1,1,1,1,4),(0.,0.0658467982010768),
(11.6150328478182,12.6111891776804,13.6073455075426,14.6035018374048,15.5996581672671,
16.5958144971293,17.5919708269915,18.5881271568537,19.5842834867159,20.5804398165781,
21.5765961464403,22.5727524763025,23.5689088061647,24.5650651360269,25.5612214658891,
26.5573777957513,27.5535341256135,28.5496904554757,29.545846785338,30.5420031152002,
31.5381594450624,32.5343157749246,33.5304721047868,34.526628434649,35.5227847645112,
36.5189410943734,37.5150974242356,38.5112537540978,39.50741008396,40.5035664138222,
41.4997227436844,42.4958790735466,43.4920354034088,44.4881917332711,45.4843480631333,
46.4805043929955,47.4766607228577,48.4728170527199,49.4689733825821,50.4651297124443,
51.4612860423065,52.4574423721687,53.4535987020309,54.4497550318931,55.4459113617553,
56.4420676916175,57.4382240214797,58.434380351342,59.4305366812042,60.4266930110664,
61.4228493409286,62.4190056707908,63.415162000653,64.4113183305152,65.4074746603774,
66.4036309902396,67.3997873201018,68.395943649964,69.3920999798262,70.3882563096884,
71.3844126395506,72.3805689694128,73.3767252992751,74.3728816291373,75.3690379589995,
76.3651942888617,77.3613506187239,78.3575069485861,79.3536632784483,80.3498196083105,
81.3459759381727,82.3421322680349,83.3382885978971,84.3344449277593,85.3306012576215,
86.3267575874837,87.322913917346,88.3190702472082,89.3152265770704,90.3113829069326,
91.3075392367948,92.303695566657,93.2998518965192,94.2960082263814,95.2921645562436,
96.2883208861058,97.284477215968,98.2806335458302,99.2767898756924,100.272946205555,
101.269102535417,102.265258865279,103.261415195141,104.257571525003,105.253727854866,
106.249884184728,107.24604051459,108.242196844452,109.238353174315),
 .UNSPECIFIED.);
#899=SHAPE_REPRESENTATION_RELATIONSHIP('SRR','None',#94379,#913);
#913=ADVANCED_BREP_SHAPE_REPRESENTATION('',(#941),#94295);
#927=STYLED_ITEM('',(#94588),#941);
#941=MANIFOLD_SOLID_BREP('Body1',#51026);
#956=TOROIDAL_SURFACE('',#54901,3.192,0.25);
#1035=FACE_BOUND('',#18428,.T.);
#1036=FACE_BOUND('',#18581,.T.);
#1037=FACE_BOUND('',#18587,.T.);
#1198=CYLINDRICAL_SURFACE('',#54859,2.942);
#1199=CYLINDRICAL_SURFACE('',#54861,2.942);
#1200=CYLINDRICAL_SURFACE('',#54862,2.942);
#1201=CYLINDRICAL_SURFACE('',#54863,2.942);
#1202=CYLINDRICAL_SURFACE('',#54864,2.942);
#1203=CYLINDRICAL_SURFACE('',#54865,2.942);
#1204=CYLINDRICAL_SURFACE('',#54866,2.942);
#1205=CYLINDRICAL_SURFACE('',#54867,2.942);
#1206=CYLINDRICAL_SURFACE('',#54868,2.942);
#1207=CYLINDRICAL_SURFACE('',#54869,2.942);
#1208=CYLINDRICAL_SURFACE('',#54870,2.942);
#1209=CYLINDRICAL_SURFACE('',#54871,2.942);
#1210=CYLINDRICAL_SURFACE('',#54872,2.942);
#1211=CYLINDRICAL_SURFACE('',#54873,2.942);
#1212=CYLINDRICAL_SURFACE('',#54874,2.942);
#1213=CYLINDRICAL_SURFACE('',#54875,2.942);
#1214=CYLINDRICAL_SURFACE('',#54877,2.37175);
#1215=CYLINDRICAL_SURFACE('',#54879,2.37175);
#1216=CYLINDRICAL_SURFACE('',#54880,2.37175);
#1217=CYLINDRICAL_SURFACE('',#54881,2.37175);
#1218=CYLINDRICAL_SURFACE('',#54882,2.37175);
#1219=CYLINDRICAL_SURFACE('',#54883,2.37175);
#1220=CYLINDRICAL_SURFACE('',#54884,2.37175);
#1221=CYLINDRICAL_SURFACE('',#54885,2.37175);
#1222=CYLINDRICAL_SURFACE('',#54886,2.37175);
#1223=CYLINDRICAL_SURFACE('',#54887,2.37175);
#1224=CYLINDRICAL_SURFACE('',#54888,2.37175);
#1225=CYLINDRICAL_SURFACE('',#54889,2.37175);
#1226=CYLINDRICAL_SURFACE('',#54890,2.37175);
#1227=CYLINDRICAL_SURFACE('',#54891,2.37175);
#1228=CYLINDRICAL_SURFACE('',#54892,2.37175);
#1229=CYLINDRICAL_SURFACE('',#54900,2.37175);
#1230=CYLINDRICAL_SURFACE('',#54905,2.942);
#1231=CYLINDRICAL_SURFACE('',#55138,5.);
#6297=LINE('',#87480,#10825);
#6298=LINE('',#87504,#10826);
#6299=LINE('',#87552,#10827);
#6300=LINE('',#87600,#10828);
#6301=LINE('',#87654,#10829);
#6302=LINE('',#87702,#10830);
#6303=LINE('',#87750,#10831);
#6304=LINE('',#87798,#10832);
#6305=LINE('',#87852,#10833);
#6306=LINE('',#87900,#10834);
#6307=LINE('',#87948,#10835);
#6308=LINE('',#88002,#10836);
#6309=LINE('',#88050,#10837);
#6310=LINE('',#88098,#10838);
#6311=LINE('',#88152,#10839);
#6312=LINE('',#88200,#10840);
#6313=LINE('',#88247,#10841);
#6314=LINE('',#88267,#10842);
#6315=LINE('',#88291,#10843);
#6316=LINE('',#88316,#10844);
#6317=LINE('',#88341,#10845);
#6318=LINE('',#88365,#10846);
#6319=LINE('',#88390,#10847);
#6320=LINE('',#88415,#10848);
#6321=LINE('',#88439,#10849);
#6322=LINE('',#88464,#10850);
#6323=LINE('',#88489,#10851);
#6324=LINE('',#88513,#10852);
#6325=LINE('',#88537,#10853);
#6326=LINE('',#88562,#10854);
#6327=LINE('',#88587,#10855);
#6328=LINE('',#89832,#10856);
#6329=LINE('',#89834,#10857);
#6330=LINE('',#89836,#10858);
#6331=LINE('',#89837,#10859);
#6332=LINE('',#89841,#10860);
#6333=LINE('',#89844,#10861);
#6334=LINE('',#89845,#10862);
#6335=LINE('',#89851,#10863);
#6336=LINE('',#89853,#10864);
#6337=LINE('',#89855,#10865);
#6338=LINE('',#89856,#10866);
#6339=LINE('',#89860,#10867);
#6340=LINE('',#89863,#10868);
#6341=LINE('',#89864,#10869);
#6342=LINE('',#89870,#10870);
#6343=LINE('',#89872,#10871);
#6344=LINE('',#89874,#10872);
#6345=LINE('',#89875,#10873);
#6346=LINE('',#89879,#10874);
#6347=LINE('',#89882,#10875);
#6348=LINE('',#89883,#10876);
#6349=LINE('',#89889,#10877);
#6350=LINE('',#89891,#10878);
#6351=LINE('',#89893,#10879);
#6352=LINE('',#89894,#10880);
#6353=LINE('',#89898,#10881);
#6354=LINE('',#89901,#10882);
#6355=LINE('',#89902,#10883);
#6356=LINE('',#89908,#10884);
#6357=LINE('',#89910,#10885);
#6358=LINE('',#89912,#10886);
#6359=LINE('',#89913,#10887);
#6360=LINE('',#89917,#10888);
#6361=LINE('',#89920,#10889);
#6362=LINE('',#89921,#10890);
#6363=LINE('',#89927,#10891);
#6364=LINE('',#89929,#10892);
#6365=LINE('',#89931,#10893);
#6366=LINE('',#89932,#10894);
#6367=LINE('',#89936,#10895);
#6368=LINE('',#89939,#10896);
#6369=LINE('',#89940,#10897);
#6370=LINE('',#89946,#10898);
#6371=LINE('',#89948,#10899);
#6372=LINE('',#89950,#10900);
#6373=LINE('',#89951,#10901);
#6374=LINE('',#89955,#10902);
#6375=LINE('',#89958,#10903);
#6376=LINE('',#89959,#10904);
#6377=LINE('',#89965,#10905);
#6378=LINE('',#89967,#10906);
#6379=LINE('',#89969,#10907);
#6380=LINE('',#89970,#10908);
#6381=LINE('',#89974,#10909);
#6382=LINE('',#89977,#10910);
#6383=LINE('',#89978,#10911);
#6384=LINE('',#89984,#10912);
#6385=LINE('',#89986,#10913);
#6386=LINE('',#89988,#10914);
#6387=LINE('',#89989,#10915);
#6388=LINE('',#89993,#10916);
#6389=LINE('',#89996,#10917);
#6390=LINE('',#89997,#10918);
#6391=LINE('',#90003,#10919);
#6392=LINE('',#90005,#10920);
#6393=LINE('',#90007,#10921);
#6394=LINE('',#90008,#10922);
#6395=LINE('',#90012,#10923);
#6396=LINE('',#90015,#10924);
#6397=LINE('',#90016,#10925);
#6398=LINE('',#90022,#10926);
#6399=LINE('',#90024,#10927);
#6400=LINE('',#90026,#10928);
#6401=LINE('',#90027,#10929);
#6402=LINE('',#90031,#10930);
#6403=LINE('',#90034,#10931);
#6404=LINE('',#90035,#10932);
#6405=LINE('',#90041,#10933);
#6406=LINE('',#90043,#10934);
#6407=LINE('',#90045,#10935);
#6408=LINE('',#90046,#10936);
#6409=LINE('',#90050,#10937);
#6410=LINE('',#90053,#10938);
#6411=LINE('',#90054,#10939);
#6412=LINE('',#90060,#10940);
#6413=LINE('',#90062,#10941);
#6414=LINE('',#90064,#10942);
#6415=LINE('',#90065,#10943);
#6416=LINE('',#90069,#10944);
#6417=LINE('',#90072,#10945);
#6418=LINE('',#90073,#10946);
#6419=LINE('',#90079,#10947);
#6420=LINE('',#90081,#10948);
#6421=LINE('',#90083,#10949);
#6422=LINE('',#90084,#10950);
#6423=LINE('',#90088,#10951);
#6424=LINE('',#90091,#10952);
#6425=LINE('',#90092,#10953);
#6426=LINE('',#90098,#10954);
#6427=LINE('',#90100,#10955);
#6428=LINE('',#90102,#10956);
#6429=LINE('',#90103,#10957);
#6430=LINE('',#90107,#10958);
#6431=LINE('',#90110,#10959);
#6432=LINE('',#90111,#10960);
#6433=LINE('',#90117,#10961);
#6434=LINE('',#90119,#10962);
#6435=LINE('',#90121,#10963);
#6436=LINE('',#90122,#10964);
#6437=LINE('',#90126,#10965);
#6438=LINE('',#90129,#10966);
#6439=LINE('',#90130,#10967);
#6440=LINE('',#90136,#10968);
#6441=LINE('',#90138,#10969);
#6442=LINE('',#90140,#10970);
#6443=LINE('',#90141,#10971);
#6444=LINE('',#90145,#10972);
#6445=LINE('',#90148,#10973);
#6446=LINE('',#90149,#10974);
#6447=LINE('',#90155,#10975);
#6448=LINE('',#90157,#10976);
#6449=LINE('',#90159,#10977);
#6450=LINE('',#90160,#10978);
#6451=LINE('',#90165,#10979);
#6452=LINE('',#90169,#10980);
#6453=LINE('',#90170,#10981);
#6454=LINE('',#90178,#10982);
#6455=LINE('',#90180,#10983);
#6456=LINE('',#90182,#10984);
#6457=LINE('',#90183,#10985);
#6458=LINE('',#90187,#10986);
#6459=LINE('',#90190,#10987);
#6460=LINE('',#90191,#10988);
#6461=LINE('',#90197,#10989);
#6462=LINE('',#90199,#10990);
#6463=LINE('',#90201,#10991);
#6464=LINE('',#90202,#10992);
#6465=LINE('',#90206,#10993);
#6466=LINE('',#90209,#10994);
#6467=LINE('',#90210,#10995);
#6468=LINE('',#90216,#10996);
#6469=LINE('',#90218,#10997);
#6470=LINE('',#90220,#10998);
#6471=LINE('',#90221,#10999);
#6472=LINE('',#90225,#11000);
#6473=LINE('',#90228,#11001);
#6474=LINE('',#90229,#11002);
#6475=LINE('',#90235,#11003);
#6476=LINE('',#90237,#11004);
#6477=LINE('',#90239,#11005);
#6478=LINE('',#90240,#11006);
#6479=LINE('',#90244,#11007);
#6480=LINE('',#90247,#11008);
#6481=LINE('',#90248,#11009);
#6482=LINE('',#90254,#11010);
#6483=LINE('',#90256,#11011);
#6484=LINE('',#90258,#11012);
#6485=LINE('',#90259,#11013);
#6486=LINE('',#90263,#11014);
#6487=LINE('',#90266,#11015);
#6488=LINE('',#90267,#11016);
#6489=LINE('',#90273,#11017);
#6490=LINE('',#90275,#11018);
#6491=LINE('',#90277,#11019);
#6492=LINE('',#90278,#11020);
#6493=LINE('',#90282,#11021);
#6494=LINE('',#90285,#11022);
#6495=LINE('',#90286,#11023);
#6496=LINE('',#90292,#11024);
#6497=LINE('',#90294,#11025);
#6498=LINE('',#90296,#11026);
#6499=LINE('',#90297,#11027);
#6500=LINE('',#90301,#11028);
#6501=LINE('',#90304,#11029);
#6502=LINE('',#90305,#11030);
#6503=LINE('',#90311,#11031);
#6504=LINE('',#90313,#11032);
#6505=LINE('',#90315,#11033);
#6506=LINE('',#90316,#11034);
#6507=LINE('',#90320,#11035);
#6508=LINE('',#90323,#11036);
#6509=LINE('',#90324,#11037);
#6510=LINE('',#90330,#11038);
#6511=LINE('',#90332,#11039);
#6512=LINE('',#90334,#11040);
#6513=LINE('',#90335,#11041);
#6514=LINE('',#90339,#11042);
#6515=LINE('',#90342,#11043);
#6516=LINE('',#90343,#11044);
#6517=LINE('',#90349,#11045);
#6518=LINE('',#90351,#11046);
#6519=LINE('',#90353,#11047);
#6520=LINE('',#90354,#11048);
#6521=LINE('',#90358,#11049);
#6522=LINE('',#90361,#11050);
#6523=LINE('',#90362,#11051);
#6524=LINE('',#90368,#11052);
#6525=LINE('',#90370,#11053);
#6526=LINE('',#90372,#11054);
#6527=LINE('',#90373,#11055);
#6528=LINE('',#90377,#11056);
#6529=LINE('',#90380,#11057);
#6530=LINE('',#90381,#11058);
#6531=LINE('',#90387,#11059);
#6532=LINE('',#90389,#11060);
#6533=LINE('',#90391,#11061);
#6534=LINE('',#90392,#11062);
#6535=LINE('',#90396,#11063);
#6536=LINE('',#90399,#11064);
#6537=LINE('',#90400,#11065);
#6538=LINE('',#90406,#11066);
#6539=LINE('',#90408,#11067);
#6540=LINE('',#90410,#11068);
#6541=LINE('',#90411,#11069);
#6542=LINE('',#90415,#11070);
#6543=LINE('',#90418,#11071);
#6544=LINE('',#90419,#11072);
#6545=LINE('',#90425,#11073);
#6546=LINE('',#90427,#11074);
#6547=LINE('',#90429,#11075);
#6548=LINE('',#90430,#11076);
#6549=LINE('',#90434,#11077);
#6550=LINE('',#90437,#11078);
#6551=LINE('',#90438,#11079);
#6552=LINE('',#90444,#11080);
#6553=LINE('',#90446,#11081);
#6554=LINE('',#90448,#11082);
#6555=LINE('',#90449,#11083);
#6556=LINE('',#90453,#11084);
#6557=LINE('',#90456,#11085);
#6558=LINE('',#90457,#11086);
#6559=LINE('',#90463,#11087);
#6560=LINE('',#90465,#11088);
#6561=LINE('',#90467,#11089);
#6562=LINE('',#90468,#11090);
#6563=LINE('',#90472,#11091);
#6564=LINE('',#90475,#11092);
#6565=LINE('',#90476,#11093);
#6566=LINE('',#90482,#11094);
#6567=LINE('',#90484,#11095);
#6568=LINE('',#90486,#11096);
#6569=LINE('',#90487,#11097);
#6570=LINE('',#90491,#11098);
#6571=LINE('',#90494,#11099);
#6572=LINE('',#90495,#11100);
#6573=LINE('',#90503,#11101);
#6574=LINE('',#90504,#11102);
#6575=LINE('',#90507,#11103);
#6576=LINE('',#90509,#11104);
#6577=LINE('',#90510,#11105);
#6578=LINE('',#90513,#11106);
#6579=LINE('',#90514,#11107);
#6580=LINE('',#90520,#11108);
#6581=LINE('',#90525,#11109);
#6582=LINE('',#90527,#11110);
#6583=LINE('',#90529,#11111);
#6584=LINE('',#90530,#11112);
#6585=LINE('',#90533,#11113);
#6586=LINE('',#90535,#11114);
#6587=LINE('',#90536,#11115);
#6588=LINE('',#90539,#11116);
#6589=LINE('',#90541,#11117);
#6590=LINE('',#90542,#11118);
#6591=LINE('',#90545,#11119);
#6592=LINE('',#90547,#11120);
#6593=LINE('',#90548,#11121);
#6594=LINE('',#90551,#11122);
#6595=LINE('',#90553,#11123);
#6596=LINE('',#90554,#11124);
#6597=LINE('',#90556,#11125);
#6598=LINE('',#90557,#11126);
#6599=LINE('',#90563,#11127);
#6600=LINE('',#90582,#11128);
#6601=LINE('',#90605,#11129);
#10825=VECTOR('',#66851,3.);
#10826=VECTOR('',#66856,3.);
#10827=VECTOR('',#66859,3.);
#10828=VECTOR('',#66862,3.);
#10829=VECTOR('',#66865,3.);
#10830=VECTOR('',#66868,3.);
#10831=VECTOR('',#66871,3.);
#10832=VECTOR('',#66874,3.);
#10833=VECTOR('',#66877,3.);
#10834=VECTOR('',#66880,3.);
#10835=VECTOR('',#66883,3.);
#10836=VECTOR('',#66886,3.);
#10837=VECTOR('',#66889,3.);
#10838=VECTOR('',#66892,3.);
#10839=VECTOR('',#66895,3.);
#10840=VECTOR('',#66898,3.);
#10841=VECTOR('',#66903,2.37175);
#10842=VECTOR('',#66908,2.37175);
#10843=VECTOR('',#66911,2.37175);
#10844=VECTOR('',#66914,2.37175);
#10845=VECTOR('',#66917,2.37175);
#10846=VECTOR('',#66920,2.37175);
#10847=VECTOR('',#66923,2.37175);
#10848=VECTOR('',#66926,2.37175);
#10849=VECTOR('',#66929,2.37175);
#10850=VECTOR('',#66932,2.37175);
#10851=VECTOR('',#66935,2.37175);
#10852=VECTOR('',#66938,2.37175);
#10853=VECTOR('',#66941,2.37175);
#10854=VECTOR('',#66944,2.37175);
#10855=VECTOR('',#66947,2.37175);
#10856=VECTOR('',#66980,10.);
#10857=VECTOR('',#66981,10.);
#10858=VECTOR('',#66982,10.);
#10859=VECTOR('',#66983,10.);
#10860=VECTOR('',#66988,10.);
#10861=VECTOR('',#66991,10.);
#10862=VECTOR('',#66992,10.);
#10863=VECTOR('',#66999,10.);
#10864=VECTOR('',#67000,10.);
#10865=VECTOR('',#67001,10.);
#10866=VECTOR('',#67002,10.);
#10867=VECTOR('',#67007,10.);
#10868=VECTOR('',#67010,10.);
#10869=VECTOR('',#67011,10.);
#10870=VECTOR('',#67018,10.);
#10871=VECTOR('',#67019,10.);
#10872=VECTOR('',#67020,10.);
#10873=VECTOR('',#67021,10.);
#10874=VECTOR('',#67026,10.);
#10875=VECTOR('',#67029,10.);
#10876=VECTOR('',#67030,10.);
#10877=VECTOR('',#67037,10.);
#10878=VECTOR('',#67038,10.);
#10879=VECTOR('',#67039,10.);
#10880=VECTOR('',#67040,10.);
#10881=VECTOR('',#67045,10.);
#10882=VECTOR('',#67048,10.);
#10883=VECTOR('',#67049,10.);
#10884=VECTOR('',#67056,10.);
#10885=VECTOR('',#67057,10.);
#10886=VECTOR('',#67058,10.);
#10887=VECTOR('',#67059,10.);
#10888=VECTOR('',#67064,10.);
#10889=VECTOR('',#67067,10.);
#10890=VECTOR('',#67068,10.);
#10891=VECTOR('',#67075,10.);
#10892=VECTOR('',#67076,10.);
#10893=VECTOR('',#67077,10.);
#10894=VECTOR('',#67078,10.);
#10895=VECTOR('',#67083,10.);
#10896=VECTOR('',#67086,10.);
#10897=VECTOR('',#67087,10.);
#10898=VECTOR('',#67094,10.);
#10899=VECTOR('',#67095,10.);
#10900=VECTOR('',#67096,10.);
#10901=VECTOR('',#67097,10.);
#10902=VECTOR('',#67102,10.);
#10903=VECTOR('',#67105,10.);
#10904=VECTOR('',#67106,10.);
#10905=VECTOR('',#67113,10.);
#10906=VECTOR('',#67114,10.);
#10907=VECTOR('',#67115,10.);
#10908=VECTOR('',#67116,10.);
#10909=VECTOR('',#67121,10.);
#10910=VECTOR('',#67124,10.);
#10911=VECTOR('',#67125,10.);
#10912=VECTOR('',#67132,10.);
#10913=VECTOR('',#67133,10.);
#10914=VECTOR('',#67134,10.);
#10915=VECTOR('',#67135,10.);
#10916=VECTOR('',#67140,10.);
#10917=VECTOR('',#67143,10.);
#10918=VECTOR('',#67144,10.);
#10919=VECTOR('',#67151,10.);
#10920=VECTOR('',#67152,10.);
#10921=VECTOR('',#67153,10.);
#10922=VECTOR('',#67154,10.);
#10923=VECTOR('',#67159,10.);
#10924=VECTOR('',#67162,10.);
#10925=VECTOR('',#67163,10.);
#10926=VECTOR('',#67170,10.);
#10927=VECTOR('',#67171,10.);
#10928=VECTOR('',#67172,10.);
#10929=VECTOR('',#67173,10.);
#10930=VECTOR('',#67178,10.);
#10931=VECTOR('',#67181,10.);
#10932=VECTOR('',#67182,10.);
#10933=VECTOR('',#67189,10.);
#10934=VECTOR('',#67190,10.);
#10935=VECTOR('',#67191,10.);
#10936=VECTOR('',#67192,10.);
#10937=VECTOR('',#67197,10.);
#10938=VECTOR('',#67200,10.);
#10939=VECTOR('',#67201,10.);
#10940=VECTOR('',#67208,10.);
#10941=VECTOR('',#67209,10.);
#10942=VECTOR('',#67210,10.);
#10943=VECTOR('',#67211,10.);
#10944=VECTOR('',#67216,10.);
#10945=VECTOR('',#67219,10.);
#10946=VECTOR('',#67220,10.);
#10947=VECTOR('',#67227,10.);
#10948=VECTOR('',#67228,10.);
#10949=VECTOR('',#67229,10.);
#10950=VECTOR('',#67230,10.);
#10951=VECTOR('',#67235,10.);
#10952=VECTOR('',#67238,10.);
#10953=VECTOR('',#67239,10.);
#10954=VECTOR('',#67246,10.);
#10955=VECTOR('',#67247,10.);
#10956=VECTOR('',#67248,10.);
#10957=VECTOR('',#67249,10.);
#10958=VECTOR('',#67254,10.);
#10959=VECTOR('',#67257,10.);
#10960=VECTOR('',#67258,10.);
#10961=VECTOR('',#67265,10.);
#10962=VECTOR('',#67266,10.);
#10963=VECTOR('',#67267,10.);
#10964=VECTOR('',#67268,10.);
#10965=VECTOR('',#67273,10.);
#10966=VECTOR('',#67276,10.);
#10967=VECTOR('',#67277,10.);
#10968=VECTOR('',#67284,10.);
#10969=VECTOR('',#67285,10.);
#10970=VECTOR('',#67286,10.);
#10971=VECTOR('',#67287,10.);
#10972=VECTOR('',#67292,10.);
#10973=VECTOR('',#67295,10.);
#10974=VECTOR('',#67296,10.);
#10975=VECTOR('',#67303,10.);
#10976=VECTOR('',#67304,10.);
#10977=VECTOR('',#67305,10.);
#10978=VECTOR('',#67306,10.);
#10979=VECTOR('',#67311,10.);
#10980=VECTOR('',#67316,10.);
#10981=VECTOR('',#67317,10.);
#10982=VECTOR('',#67326,10.);
#10983=VECTOR('',#67327,10.);
#10984=VECTOR('',#67328,10.);
#10985=VECTOR('',#67329,10.);
#10986=VECTOR('',#67334,10.);
#10987=VECTOR('',#67337,10.);
#10988=VECTOR('',#67338,10.);
#10989=VECTOR('',#67345,10.);
#10990=VECTOR('',#67346,10.);
#10991=VECTOR('',#67347,10.);
#10992=VECTOR('',#67348,10.);
#10993=VECTOR('',#67353,10.);
#10994=VECTOR('',#67356,10.);
#10995=VECTOR('',#67357,10.);
#10996=VECTOR('',#67364,10.);
#10997=VECTOR('',#67365,10.);
#10998=VECTOR('',#67366,10.);
#10999=VECTOR('',#67367,10.);
#11000=VECTOR('',#67372,10.);
#11001=VECTOR('',#67375,10.);
#11002=VECTOR('',#67376,10.);
#11003=VECTOR('',#67383,10.);
#11004=VECTOR('',#67384,10.);
#11005=VECTOR('',#67385,10.);
#11006=VECTOR('',#67386,10.);
#11007=VECTOR('',#67391,10.);
#11008=VECTOR('',#67394,10.);
#11009=VECTOR('',#67395,10.);
#11010=VECTOR('',#67402,10.);
#11011=VECTOR('',#67403,10.);
#11012=VECTOR('',#67404,10.);
#11013=VECTOR('',#67405,10.);
#11014=VECTOR('',#67410,10.);
#11015=VECTOR('',#67413,10.);
#11016=VECTOR('',#67414,10.);
#11017=VECTOR('',#67421,10.);
#11018=VECTOR('',#67422,10.);
#11019=VECTOR('',#67423,10.);
#11020=VECTOR('',#67424,10.);
#11021=VECTOR('',#67429,10.);
#11022=VECTOR('',#67432,10.);
#11023=VECTOR('',#67433,10.);
#11024=VECTOR('',#67440,10.);
#11025=VECTOR('',#67441,10.);
#11026=VECTOR('',#67442,10.);
#11027=VECTOR('',#67443,10.);
#11028=VECTOR('',#67448,10.);
#11029=VECTOR('',#67451,10.);
#11030=VECTOR('',#67452,10.);
#11031=VECTOR('',#67459,10.);
#11032=VECTOR('',#67460,10.);
#11033=VECTOR('',#67461,10.);
#11034=VECTOR('',#67462,10.);
#11035=VECTOR('',#67467,10.);
#11036=VECTOR('',#67470,10.);
#11037=VECTOR('',#67471,10.);
#11038=VECTOR('',#67478,10.);
#11039=VECTOR('',#67479,10.);
#11040=VECTOR('',#67480,10.);
#11041=VECTOR('',#67481,10.);
#11042=VECTOR('',#67486,10.);
#11043=VECTOR('',#67489,10.);
#11044=VECTOR('',#67490,10.);
#11045=VECTOR('',#67497,10.);
#11046=VECTOR('',#67498,10.);
#11047=VECTOR('',#67499,10.);
#11048=VECTOR('',#67500,10.);
#11049=VECTOR('',#67505,10.);
#11050=VECTOR('',#67508,10.);
#11051=VECTOR('',#67509,10.);
#11052=VECTOR('',#67516,10.);
#11053=VECTOR('',#67517,10.);
#11054=VECTOR('',#67518,10.);
#11055=VECTOR('',#67519,10.);
#11056=VECTOR('',#67524,10.);
#11057=VECTOR('',#67527,10.);
#11058=VECTOR('',#67528,10.);
#11059=VECTOR('',#67535,10.);
#11060=VECTOR('',#67536,10.);
#11061=VECTOR('',#67537,10.);
#11062=VECTOR('',#67538,10.);
#11063=VECTOR('',#67543,10.);
#11064=VECTOR('',#67546,10.);
#11065=VECTOR('',#67547,10.);
#11066=VECTOR('',#67554,10.);
#11067=VECTOR('',#67555,10.);
#11068=VECTOR('',#67556,10.);
#11069=VECTOR('',#67557,10.);
#11070=VECTOR('',#67562,10.);
#11071=VECTOR('',#67565,10.);
#11072=VECTOR('',#67566,10.);
#11073=VECTOR('',#67573,10.);
#11074=VECTOR('',#67574,10.);
#11075=VECTOR('',#67575,10.);
#11076=VECTOR('',#67576,10.);
#11077=VECTOR('',#67581,10.);
#11078=VECTOR('',#67584,10.);
#11079=VECTOR('',#67585,10.);
#11080=VECTOR('',#67592,10.);
#11081=VECTOR('',#67593,10.);
#11082=VECTOR('',#67594,10.);
#11083=VECTOR('',#67595,10.);
#11084=VECTOR('',#67600,10.);
#11085=VECTOR('',#67603,10.);
#11086=VECTOR('',#67604,10.);
#11087=VECTOR('',#67611,10.);
#11088=VECTOR('',#67612,10.);
#11089=VECTOR('',#67613,10.);
#11090=VECTOR('',#67614,10.);
#11091=VECTOR('',#67619,10.);
#11092=VECTOR('',#67622,10.);
#11093=VECTOR('',#67623,10.);
#11094=VECTOR('',#67630,10.);
#11095=VECTOR('',#67631,10.);
#11096=VECTOR('',#67632,10.);
#11097=VECTOR('',#67633,10.);
#11098=VECTOR('',#67638,10.);
#11099=VECTOR('',#67641,10.);
#11100=VECTOR('',#67642,10.);
#11101=VECTOR('',#67651,10.);
#11102=VECTOR('',#67652,10.);
#11103=VECTOR('',#67655,10.);
#11104=VECTOR('',#67656,10.);
#11105=VECTOR('',#67657,10.);
#11106=VECTOR('',#67660,10.);
#11107=VECTOR('',#67661,10.);
#11108=VECTOR('',#67668,1.25);
#11109=VECTOR('',#67673,10.);
#11110=VECTOR('',#67674,10.);
#11111=VECTOR('',#67675,10.);
#11112=VECTOR('',#67676,10.);
#11113=VECTOR('',#67679,10.);
#11114=VECTOR('',#67680,10.);
#11115=VECTOR('',#67681,10.);
#11116=VECTOR('',#67684,10.);
#11117=VECTOR('',#67685,10.);
#11118=VECTOR('',#67686,10.);
#11119=VECTOR('',#67689,10.);
#11120=VECTOR('',#67690,10.);
#11121=VECTOR('',#67691,10.);
#11122=VECTOR('',#67694,10.);
#11123=VECTOR('',#67695,10.);
#11124=VECTOR('',#67696,10.);
#11125=VECTOR('',#67699,10.);
#11126=VECTOR('',#67700,10.);
#11127=VECTOR('',#67709,2.7);
#11128=VECTOR('',#67746,5.);
#11129=VECTOR('',#67789,4.7);
#13065=PLANE('',#54893);
#13066=PLANE('',#54896);
#13067=PLANE('',#54906);
#13068=PLANE('',#54908);
#13069=PLANE('',#54909);
#13070=PLANE('',#54911);
#13071=PLANE('',#54912);
#13072=PLANE('',#54914);
#13073=PLANE('',#54915);
#13074=PLANE('',#54917);
#13075=PLANE('',#54918);
#13076=PLANE('',#54920);
#13077=PLANE('',#54921);
#13078=PLANE('',#54923);
#13079=PLANE('',#54924);
#13080=PLANE('',#54926);
#13081=PLANE('',#54927);
#13082=PLANE('',#54929);
#13083=PLANE('',#54930);
#13084=PLANE('',#54932);
#13085=PLANE('',#54933);
#13086=PLANE('',#54935);
#13087=PLANE('',#54936);
#13088=PLANE('',#54938);
#13089=PLANE('',#54939);
#13090=PLANE('',#54941);
#13091=PLANE('',#54942);
#13092=PLANE('',#54944);
#13093=PLANE('',#54945);
#13094=PLANE('',#54947);
#13095=PLANE('',#54948);
#13096=PLANE('',#54950);
#13097=PLANE('',#54951);
#13098=PLANE('',#54953);
#13099=PLANE('',#54954);
#13100=PLANE('',#54956);
#13101=PLANE('',#54957);
#13102=PLANE('',#54959);
#13103=PLANE('',#54960);
#13104=PLANE('',#54962);
#13105=PLANE('',#54963);
#13106=PLANE('',#54965);
#13107=PLANE('',#54966);
#13108=PLANE('',#54968);
#13109=PLANE('',#54969);
#13110=PLANE('',#54971);
#13111=PLANE('',#54972);
#13112=PLANE('',#54974);
#13113=PLANE('',#54975);
#13114=PLANE('',#54977);
#13115=PLANE('',#54978);
#13116=PLANE('',#54980);
#13117=PLANE('',#54981);
#13118=PLANE('',#54983);
#13119=PLANE('',#54984);
#13120=PLANE('',#54986);
#13121=PLANE('',#54987);
#13122=PLANE('',#54989);
#13123=PLANE('',#54990);
#13124=PLANE('',#54992);
#13125=PLANE('',#54993);
#13126=PLANE('',#54995);
#13127=PLANE('',#54996);
#13128=PLANE('',#54998);
#13129=PLANE('',#54999);
#13130=PLANE('',#55001);
#13131=PLANE('',#55002);
#13132=PLANE('',#55004);
#13133=PLANE('',#55005);
#13134=PLANE('',#55007);
#13135=PLANE('',#55008);
#13136=PLANE('',#55010);
#13137=PLANE('',#55011);
#13138=PLANE('',#55014);
#13139=PLANE('',#55015);
#13140=PLANE('',#55018);
#13141=PLANE('',#55019);
#13142=PLANE('',#55021);
#13143=PLANE('',#55022);
#13144=PLANE('',#55024);
#13145=PLANE('',#55025);
#13146=PLANE('',#55027);
#13147=PLANE('',#55028);
#13148=PLANE('',#55030);
#13149=PLANE('',#55031);
#13150=PLANE('',#55033);
#13151=PLANE('',#55034);
#13152=PLANE('',#55036);
#13153=PLANE('',#55037);
#13154=PLANE('',#55039);
#13155=PLANE('',#55040);
#13156=PLANE('',#55042);
#13157=PLANE('',#55043);
#13158=PLANE('',#55045);
#13159=PLANE('',#55046);
#13160=PLANE('',#55048);
#13161=PLANE('',#55049);
#13162=PLANE('',#55051);
#13163=PLANE('',#55052);
#13164=PLANE('',#55054);
#13165=PLANE('',#55055);
#13166=PLANE('',#55057);
#13167=PLANE('',#55058);
#13168=PLANE('',#55060);
#13169=PLANE('',#55061);
#13170=PLANE('',#55063);
#13171=PLANE('',#55064);
#13172=PLANE('',#55066);
#13173=PLANE('',#55067);
#13174=PLANE('',#55069);
#13175=PLANE('',#55070);
#13176=PLANE('',#55072);
#13177=PLANE('',#55073);
#13178=PLANE('',#55075);
#13179=PLANE('',#55076);
#13180=PLANE('',#55078);
#13181=PLANE('',#55079);
#13182=PLANE('',#55081);
#13183=PLANE('',#55082);
#13184=PLANE('',#55084);
#13185=PLANE('',#55085);
#13186=PLANE('',#55087);
#13187=PLANE('',#55088);
#13188=PLANE('',#55090);
#13189=PLANE('',#55091);
#13190=PLANE('',#55093);
#13191=PLANE('',#55094);
#13192=PLANE('',#55096);
#13193=PLANE('',#55097);
#13194=PLANE('',#55099);
#13195=PLANE('',#55100);
#13196=PLANE('',#55102);
#13197=PLANE('',#55103);
#13198=PLANE('',#55105);
#13199=PLANE('',#55106);
#13200=PLANE('',#55108);
#13201=PLANE('',#55109);
#13202=PLANE('',#55111);
#13203=PLANE('',#55112);
#13204=PLANE('',#55114);
#13205=PLANE('',#55115);
#13206=PLANE('',#55117);
#13207=PLANE('',#55118);
#13208=PLANE('',#55120);
#13209=PLANE('',#55122);
#13210=PLANE('',#55123);
#13211=PLANE('',#55124);
#13212=PLANE('',#55128);
#13213=PLANE('',#55129);
#13214=PLANE('',#55130);
#13215=PLANE('',#55131);
#13216=PLANE('',#55132);
#13217=PLANE('',#55133);
#13218=PLANE('',#55134);
#13219=PLANE('',#55135);
#13220=PLANE('',#55177);
#15631=FACE_OUTER_BOUND('',#18389,.T.);
#15632=FACE_OUTER_BOUND('',#18390,.T.);
#15633=FACE_OUTER_BOUND('',#18391,.T.);
#15634=FACE_OUTER_BOUND('',#18392,.T.);
#15635=FACE_OUTER_BOUND('',#18393,.T.);
#15636=FACE_OUTER_BOUND('',#18394,.T.);
#15637=FACE_OUTER_BOUND('',#18395,.T.);
#15638=FACE_OUTER_BOUND('',#18396,.T.);
#15639=FACE_OUTER_BOUND('',#18397,.T.);
#15640=FACE_OUTER_BOUND('',#18398,.T.);
#15641=FACE_OUTER_BOUND('',#18399,.T.);
#15642=FACE_OUTER_BOUND('',#18400,.T.);
#15643=FACE_OUTER_BOUND('',#18401,.T.);
#15644=FACE_OUTER_BOUND('',#18402,.T.);
#15645=FACE_OUTER_BOUND('',#18403,.T.);
#15646=FACE_OUTER_BOUND('',#18404,.T.);
#15647=FACE_OUTER_BOUND('',#18405,.T.);
#15648=FACE_OUTER_BOUND('',#18406,.T.);
#15649=FACE_OUTER_BOUND('',#18407,.T.);
#15650=FACE_OUTER_BOUND('',#18408,.T.);
#15651=FACE_OUTER_BOUND('',#18409,.T.);
#15652=FACE_OUTER_BOUND('',#18410,.T.);
#15653=FACE_OUTER_BOUND('',#18411,.T.);
#15654=FACE_OUTER_BOUND('',#18412,.T.);
#15655=FACE_OUTER_BOUND('',#18413,.T.);
#15656=FACE_OUTER_BOUND('',#18414,.T.);
#15657=FACE_OUTER_BOUND('',#18415,.T.);
#15658=FACE_OUTER_BOUND('',#18416,.T.);
#15659=FACE_OUTER_BOUND('',#18417,.T.);
#15660=FACE_OUTER_BOUND('',#18418,.T.);
#15661=FACE_OUTER_BOUND('',#18419,.T.);
#15662=FACE_OUTER_BOUND('',#18420,.T.);
#15663=FACE_OUTER_BOUND('',#18421,.T.);
#15664=FACE_OUTER_BOUND('',#18422,.T.);
#15665=FACE_OUTER_BOUND('',#18423,.T.);
#15666=FACE_OUTER_BOUND('',#18424,.T.);
#15667=FACE_OUTER_BOUND('',#18425,.T.);
#15668=FACE_OUTER_BOUND('',#18426,.T.);
#15669=FACE_OUTER_BOUND('',#18427,.T.);
#15670=FACE_OUTER_BOUND('',#18429,.T.);
#15671=FACE_OUTER_BOUND('',#18430,.T.);
#15672=FACE_OUTER_BOUND('',#18431,.T.);
#15673=FACE_OUTER_BOUND('',#18432,.T.);
#15674=FACE_OUTER_BOUND('',#18433,.T.);
#15675=FACE_OUTER_BOUND('',#18434,.T.);
#15676=FACE_OUTER_BOUND('',#18435,.T.);
#15677=FACE_OUTER_BOUND('',#18436,.T.);
#15678=FACE_OUTER_BOUND('',#18437,.T.);
#15679=FACE_OUTER_BOUND('',#18438,.T.);
#15680=FACE_OUTER_BOUND('',#18439,.T.);
#15681=FACE_OUTER_BOUND('',#18440,.T.);
#15682=FACE_OUTER_BOUND('',#18441,.T.);
#15683=FACE_OUTER_BOUND('',#18442,.T.);
#15684=FACE_OUTER_BOUND('',#18443,.T.);
#15685=FACE_OUTER_BOUND('',#18444,.T.);
#15686=FACE_OUTER_BOUND('',#18445,.T.);
#15687=FACE_OUTER_BOUND('',#18446,.T.);
#15688=FACE_OUTER_BOUND('',#18447,.T.);
#15689=FACE_OUTER_BOUND('',#18448,.T.);
#15690=FACE_OUTER_BOUND('',#18449,.T.);
#15691=FACE_OUTER_BOUND('',#18450,.T.);
#15692=FACE_OUTER_BOUND('',#18451,.T.);
#15693=FACE_OUTER_BOUND('',#18452,.T.);
#15694=FACE_OUTER_BOUND('',#18453,.T.);
#15695=FACE_OUTER_BOUND('',#18454,.T.);
#15696=FACE_OUTER_BOUND('',#18455,.T.);
#15697=FACE_OUTER_BOUND('',#18456,.T.);
#15698=FACE_OUTER_BOUND('',#18457,.T.);
#15699=FACE_OUTER_BOUND('',#18458,.T.);
#15700=FACE_OUTER_BOUND('',#18459,.T.);
#15701=FACE_OUTER_BOUND('',#18460,.T.);
#15702=FACE_OUTER_BOUND('',#18461,.T.);
#15703=FACE_OUTER_BOUND('',#18462,.T.);
#15704=FACE_OUTER_BOUND('',#18463,.T.);
#15705=FACE_OUTER_BOUND('',#18464,.T.);
#15706=FACE_OUTER_BOUND('',#18465,.T.);
#15707=FACE_OUTER_BOUND('',#18466,.T.);
#15708=FACE_OUTER_BOUND('',#18467,.T.);
#15709=FACE_OUTER_BOUND('',#18468,.T.);
#15710=FACE_OUTER_BOUND('',#18469,.T.);
#15711=FACE_OUTER_BOUND('',#18470,.T.);
#15712=FACE_OUTER_BOUND('',#18471,.T.);
#15713=FACE_OUTER_BOUND('',#18472,.T.);
#15714=FACE_OUTER_BOUND('',#18473,.T.);
#15715=FACE_OUTER_BOUND('',#18474,.T.);
#15716=FACE_OUTER_BOUND('',#18475,.T.);
#15717=FACE_OUTER_BOUND('',#18476,.T.);
#15718=FACE_OUTER_BOUND('',#18477,.T.);
#15719=FACE_OUTER_BOUND('',#18478,.T.);
#15720=FACE_OUTER_BOUND('',#18479,.T.);
#15721=FACE_OUTER_BOUND('',#18480,.T.);
#15722=FACE_OUTER_BOUND('',#18481,.T.);
#15723=FACE_OUTER_BOUND('',#18482,.T.);
#15724=FACE_OUTER_BOUND('',#18483,.T.);
#15725=FACE_OUTER_BOUND('',#18484,.T.);
#15726=FACE_OUTER_BOUND('',#18485,.T.);
#15727=FACE_OUTER_BOUND('',#18486,.T.);
#15728=FACE_OUTER_BOUND('',#18487,.T.);
#15729=FACE_OUTER_BOUND('',#18488,.T.);
#15730=FACE_OUTER_BOUND('',#18489,.T.);
#15731=FACE_OUTER_BOUND('',#18490,.T.);
#15732=FACE_OUTER_BOUND('',#18491,.T.);
#15733=FACE_OUTER_BOUND('',#18492,.T.);
#15734=FACE_OUTER_BOUND('',#18493,.T.);
#15735=FACE_OUTER_BOUND('',#18494,.T.);
#15736=FACE_OUTER_BOUND('',#18495,.T.);
#15737=FACE_OUTER_BOUND('',#18496,.T.);
#15738=FACE_OUTER_BOUND('',#18497,.T.);
#15739=FACE_OUTER_BOUND('',#18498,.T.);
#15740=FACE_OUTER_BOUND('',#18499,.T.);
#15741=FACE_OUTER_BOUND('',#18500,.T.);
#15742=FACE_OUTER_BOUND('',#18501,.T.);
#15743=FACE_OUTER_BOUND('',#18502,.T.);
#15744=FACE_OUTER_BOUND('',#18503,.T.);
#15745=FACE_OUTER_BOUND('',#18504,.T.);
#15746=FACE_OUTER_BOUND('',#18505,.T.);
#15747=FACE_OUTER_BOUND('',#18506,.T.);
#15748=FACE_OUTER_BOUND('',#18507,.T.);
#15749=FACE_OUTER_BOUND('',#18508,.T.);
#15750=FACE_OUTER_BOUND('',#18509,.T.);
#15751=FACE_OUTER_BOUND('',#18510,.T.);
#15752=FACE_OUTER_BOUND('',#18511,.T.);
#15753=FACE_OUTER_BOUND('',#18512,.T.);
#15754=FACE_OUTER_BOUND('',#18513,.T.);
#15755=FACE_OUTER_BOUND('',#18514,.T.);
#15756=FACE_OUTER_BOUND('',#18515,.T.);
#15757=FACE_OUTER_BOUND('',#18516,.T.);
#15758=FACE_OUTER_BOUND('',#18517,.T.);
#15759=FACE_OUTER_BOUND('',#18518,.T.);
#15760=FACE_OUTER_BOUND('',#18519,.T.);
#15761=FACE_OUTER_BOUND('',#18520,.T.);
#15762=FACE_OUTER_BOUND('',#18521,.T.);
#15763=FACE_OUTER_BOUND('',#18522,.T.);
#15764=FACE_OUTER_BOUND('',#18523,.T.);
#15765=FACE_OUTER_BOUND('',#18524,.T.);
#15766=FACE_OUTER_BOUND('',#18525,.T.);
#15767=FACE_OUTER_BOUND('',#18526,.T.);
#15768=FACE_OUTER_BOUND('',#18527,.T.);
#15769=FACE_OUTER_BOUND('',#18528,.T.);
#15770=FACE_OUTER_BOUND('',#18529,.T.);
#15771=FACE_OUTER_BOUND('',#18530,.T.);
#15772=FACE_OUTER_BOUND('',#18531,.T.);
#15773=FACE_OUTER_BOUND('',#18532,.T.);
#15774=FACE_OUTER_BOUND('',#18533,.T.);
#15775=FACE_OUTER_BOUND('',#18534,.T.);
#15776=FACE_OUTER_BOUND('',#18535,.T.);
#15777=FACE_OUTER_BOUND('',#18536,.T.);
#15778=FACE_OUTER_BOUND('',#18537,.T.);
#15779=FACE_OUTER_BOUND('',#18538,.T.);
#15780=FACE_OUTER_BOUND('',#18539,.T.);
#15781=FACE_OUTER_BOUND('',#18540,.T.);
#15782=FACE_OUTER_BOUND('',#18541,.T.);
#15783=FACE_OUTER_BOUND('',#18542,.T.);
#15784=FACE_OUTER_BOUND('',#18543,.T.);
#15785=FACE_OUTER_BOUND('',#18544,.T.);
#15786=FACE_OUTER_BOUND('',#18545,.T.);
#15787=FACE_OUTER_BOUND('',#18546,.T.);
#15788=FACE_OUTER_BOUND('',#18547,.T.);
#15789=FACE_OUTER_BOUND('',#18548,.T.);
#15790=FACE_OUTER_BOUND('',#18549,.T.);
#15791=FACE_OUTER_BOUND('',#18550,.T.);
#15792=FACE_OUTER_BOUND('',#18551,.T.);
#15793=FACE_OUTER_BOUND('',#18552,.T.);
#15794=FACE_OUTER_BOUND('',#18553,.T.);
#15795=FACE_OUTER_BOUND('',#18554,.T.);
#15796=FACE_OUTER_BOUND('',#18555,.T.);
#15797=FACE_OUTER_BOUND('',#18556,.T.);
#15798=FACE_OUTER_BOUND('',#18557,.T.);
#15799=FACE_OUTER_BOUND('',#18558,.T.);
#15800=FACE_OUTER_BOUND('',#18559,.T.);
#15801=FACE_OUTER_BOUND('',#18560,.T.);
#15802=FACE_OUTER_BOUND('',#18561,.T.);
#15803=FACE_OUTER_BOUND('',#18562,.T.);
#15804=FACE_OUTER_BOUND('',#18563,.T.);
#15805=FACE_OUTER_BOUND('',#18564,.T.);
#15806=FACE_OUTER_BOUND('',#18565,.T.);
#15807=FACE_OUTER_BOUND('',#18566,.T.);
#15808=FACE_OUTER_BOUND('',#18567,.T.);
#15809=FACE_OUTER_BOUND('',#18568,.T.);
#15810=FACE_OUTER_BOUND('',#18569,.T.);
#15811=FACE_OUTER_BOUND('',#18570,.T.);
#15812=FACE_OUTER_BOUND('',#18571,.T.);
#15813=FACE_OUTER_BOUND('',#18572,.T.);
#15814=FACE_OUTER_BOUND('',#18573,.T.);
#15815=FACE_OUTER_BOUND('',#18574,.T.);
#15816=FACE_OUTER_BOUND('',#18575,.T.);
#15817=FACE_OUTER_BOUND('',#18576,.T.);
#15818=FACE_OUTER_BOUND('',#18577,.T.);
#15819=FACE_OUTER_BOUND('',#18578,.T.);
#15820=FACE_OUTER_BOUND('',#18579,.T.);
#15821=FACE_OUTER_BOUND('',#18580,.T.);
#15822=FACE_OUTER_BOUND('',#18582,.T.);
#15823=FACE_OUTER_BOUND('',#18583,.T.);
#15824=FACE_OUTER_BOUND('',#18584,.T.);
#15825=FACE_OUTER_BOUND('',#18585,.T.);
#15826=FACE_OUTER_BOUND('',#18586,.T.);
#18389=EDGE_LOOP('',(#46595,#46596,#46597,#46598));
#18390=EDGE_LOOP('',(#46599,#46600,#46601,#46602));
#18391=EDGE_LOOP('',(#46603,#46604,#46605,#46606));
#18392=EDGE_LOOP('',(#46607,#46608,#46609,#46610));
#18393=EDGE_LOOP('',(#46611,#46612,#46613,#46614));
#18394=EDGE_LOOP('',(#46615,#46616,#46617,#46618));
#18395=EDGE_LOOP('',(#46619,#46620,#46621,#46622));
#18396=EDGE_LOOP('',(#46623,#46624,#46625,#46626));
#18397=EDGE_LOOP('',(#46627,#46628,#46629,#46630));
#18398=EDGE_LOOP('',(#46631,#46632,#46633,#46634));
#18399=EDGE_LOOP('',(#46635,#46636,#46637,#46638));
#18400=EDGE_LOOP('',(#46639,#46640,#46641,#46642));
#18401=EDGE_LOOP('',(#46643,#46644,#46645,#46646));
#18402=EDGE_LOOP('',(#46647,#46648,#46649,#46650));
#18403=EDGE_LOOP('',(#46651,#46652,#46653,#46654));
#18404=EDGE_LOOP('',(#46655,#46656,#46657,#46658,#46659));
#18405=EDGE_LOOP('',(#46660,#46661,#46662,#46663));
#18406=EDGE_LOOP('',(#46664,#46665,#46666,#46667));
#18407=EDGE_LOOP('',(#46668,#46669,#46670,#46671));
#18408=EDGE_LOOP('',(#46672,#46673,#46674,#46675));
#18409=EDGE_LOOP('',(#46676,#46677,#46678,#46679));
#18410=EDGE_LOOP('',(#46680,#46681,#46682,#46683));
#18411=EDGE_LOOP('',(#46684,#46685,#46686,#46687));
#18412=EDGE_LOOP('',(#46688,#46689,#46690,#46691));
#18413=EDGE_LOOP('',(#46692,#46693,#46694,#46695));
#18414=EDGE_LOOP('',(#46696,#46697,#46698,#46699));
#18415=EDGE_LOOP('',(#46700,#46701,#46702,#46703));
#18416=EDGE_LOOP('',(#46704,#46705,#46706,#46707));
#18417=EDGE_LOOP('',(#46708,#46709,#46710,#46711));
#18418=EDGE_LOOP('',(#46712,#46713,#46714,#46715));
#18419=EDGE_LOOP('',(#46716,#46717,#46718,#46719));
#18420=EDGE_LOOP('',(#46720,#46721,#46722,#46723,#46724));
#18421=EDGE_LOOP('',(#46725,#46726,#46727,#46728,#46729,#46730,#46731,#46732,
#46733,#46734,#46735,#46736,#46737,#46738,#46739,#46740,#46741,#46742,#46743,
#46744,#46745,#46746,#46747,#46748,#46749,#46750,#46751,#46752,#46753,#46754,
#46755,#46756,#46757,#46758,#46759));
#18422=EDGE_LOOP('',(#46760,#46761,#46762,#46763,#46764));
#18423=EDGE_LOOP('',(#46765,#46766,#46767,#46768));
#18424=EDGE_LOOP('',(#46769,#46770,#46771,#46772,#46773,#46774,#46775,#46776,
#46777,#46778,#46779,#46780,#46781,#46782,#46783,#46784,#46785,#46786,#46787,
#46788,#46789,#46790,#46791,#46792,#46793,#46794,#46795,#46796,#46797,#46798,
#46799,#46800,#46801,#46802));
#18425=EDGE_LOOP('',(#46803,#46804,#46805,#46806,#46807,#46808,#46809));
#18426=EDGE_LOOP('',(#46810,#46811,#46812));
#18427=EDGE_LOOP('',(#46813));
#18428=EDGE_LOOP('',(#46814));
#18429=EDGE_LOOP('',(#46815,#46816,#46817,#46818));
#18430=EDGE_LOOP('',(#46819,#46820,#46821));
#18431=EDGE_LOOP('',(#46822,#46823,#46824,#46825));
#18432=EDGE_LOOP('',(#46826,#46827,#46828));
#18433=EDGE_LOOP('',(#46829,#46830,#46831,#46832));
#18434=EDGE_LOOP('',(#46833,#46834,#46835));
#18435=EDGE_LOOP('',(#46836,#46837,#46838,#46839));
#18436=EDGE_LOOP('',(#46840,#46841,#46842));
#18437=EDGE_LOOP('',(#46843,#46844,#46845,#46846));
#18438=EDGE_LOOP('',(#46847,#46848,#46849));
#18439=EDGE_LOOP('',(#46850,#46851,#46852,#46853));
#18440=EDGE_LOOP('',(#46854,#46855,#46856));
#18441=EDGE_LOOP('',(#46857,#46858,#46859,#46860));
#18442=EDGE_LOOP('',(#46861,#46862,#46863));
#18443=EDGE_LOOP('',(#46864,#46865,#46866,#46867));
#18444=EDGE_LOOP('',(#46868,#46869,#46870));
#18445=EDGE_LOOP('',(#46871,#46872,#46873,#46874));
#18446=EDGE_LOOP('',(#46875,#46876,#46877));
#18447=EDGE_LOOP('',(#46878,#46879,#46880,#46881));
#18448=EDGE_LOOP('',(#46882,#46883,#46884));
#18449=EDGE_LOOP('',(#46885,#46886,#46887,#46888));
#18450=EDGE_LOOP('',(#46889,#46890,#46891));
#18451=EDGE_LOOP('',(#46892,#46893,#46894,#46895));
#18452=EDGE_LOOP('',(#46896,#46897,#46898));
#18453=EDGE_LOOP('',(#46899,#46900,#46901,#46902));
#18454=EDGE_LOOP('',(#46903,#46904,#46905));
#18455=EDGE_LOOP('',(#46906,#46907,#46908,#46909));
#18456=EDGE_LOOP('',(#46910,#46911,#46912));
#18457=EDGE_LOOP('',(#46913,#46914,#46915,#46916));
#18458=EDGE_LOOP('',(#46917,#46918,#46919));
#18459=EDGE_LOOP('',(#46920,#46921,#46922,#46923));
#18460=EDGE_LOOP('',(#46924,#46925,#46926));
#18461=EDGE_LOOP('',(#46927,#46928,#46929,#46930));
#18462=EDGE_LOOP('',(#46931,#46932,#46933));
#18463=EDGE_LOOP('',(#46934,#46935,#46936,#46937));
#18464=EDGE_LOOP('',(#46938,#46939,#46940));
#18465=EDGE_LOOP('',(#46941,#46942,#46943,#46944));
#18466=EDGE_LOOP('',(#46945,#46946,#46947));
#18467=EDGE_LOOP('',(#46948,#46949,#46950,#46951));
#18468=EDGE_LOOP('',(#46952,#46953,#46954));
#18469=EDGE_LOOP('',(#46955,#46956,#46957,#46958));
#18470=EDGE_LOOP('',(#46959,#46960,#46961));
#18471=EDGE_LOOP('',(#46962,#46963,#46964,#46965));
#18472=EDGE_LOOP('',(#46966,#46967,#46968));
#18473=EDGE_LOOP('',(#46969,#46970,#46971,#46972));
#18474=EDGE_LOOP('',(#46973,#46974,#46975));
#18475=EDGE_LOOP('',(#46976,#46977,#46978,#46979));
#18476=EDGE_LOOP('',(#46980,#46981,#46982));
#18477=EDGE_LOOP('',(#46983,#46984,#46985,#46986));
#18478=EDGE_LOOP('',(#46987,#46988,#46989));
#18479=EDGE_LOOP('',(#46990,#46991,#46992,#46993));
#18480=EDGE_LOOP('',(#46994,#46995,#46996));
#18481=EDGE_LOOP('',(#46997,#46998,#46999,#47000));
#18482=EDGE_LOOP('',(#47001,#47002,#47003));
#18483=EDGE_LOOP('',(#47004,#47005,#47006,#47007));
#18484=EDGE_LOOP('',(#47008,#47009,#47010));
#18485=EDGE_LOOP('',(#47011,#47012,#47013,#47014));
#18486=EDGE_LOOP('',(#47015,#47016,#47017));
#18487=EDGE_LOOP('',(#47018,#47019,#47020,#47021));
#18488=EDGE_LOOP('',(#47022,#47023,#47024));
#18489=EDGE_LOOP('',(#47025,#47026,#47027,#47028));
#18490=EDGE_LOOP('',(#47029,#47030,#47031));
#18491=EDGE_LOOP('',(#47032,#47033,#47034,#47035));
#18492=EDGE_LOOP('',(#47036,#47037,#47038));
#18493=EDGE_LOOP('',(#47039,#47040,#47041,#47042));
#18494=EDGE_LOOP('',(#47043,#47044,#47045));
#18495=EDGE_LOOP('',(#47046,#47047,#47048,#47049));
#18496=EDGE_LOOP('',(#47050,#47051,#47052));
#18497=EDGE_LOOP('',(#47053,#47054,#47055,#47056));
#18498=EDGE_LOOP('',(#47057,#47058,#47059,#47060));
#18499=EDGE_LOOP('',(#47061,#47062,#47063,#47064));
#18500=EDGE_LOOP('',(#47065,#47066,#47067,#47068));
#18501=EDGE_LOOP('',(#47069,#47070,#47071,#47072));
#18502=EDGE_LOOP('',(#47073,#47074,#47075));
#18503=EDGE_LOOP('',(#47076,#47077,#47078,#47079));
#18504=EDGE_LOOP('',(#47080,#47081,#47082));
#18505=EDGE_LOOP('',(#47083,#47084,#47085,#47086));
#18506=EDGE_LOOP('',(#47087,#47088,#47089));
#18507=EDGE_LOOP('',(#47090,#47091,#47092,#47093));
#18508=EDGE_LOOP('',(#47094,#47095,#47096));
#18509=EDGE_LOOP('',(#47097,#47098,#47099,#47100));
#18510=EDGE_LOOP('',(#47101,#47102,#47103));
#18511=EDGE_LOOP('',(#47104,#47105,#47106,#47107));
#18512=EDGE_LOOP('',(#47108,#47109,#47110));
#18513=EDGE_LOOP('',(#47111,#47112,#47113,#47114));
#18514=EDGE_LOOP('',(#47115,#47116,#47117));
#18515=EDGE_LOOP('',(#47118,#47119,#47120,#47121));
#18516=EDGE_LOOP('',(#47122,#47123,#47124));
#18517=EDGE_LOOP('',(#47125,#47126,#47127,#47128));
#18518=EDGE_LOOP('',(#47129,#47130,#47131));
#18519=EDGE_LOOP('',(#47132,#47133,#47134,#47135));
#18520=EDGE_LOOP('',(#47136,#47137,#47138));
#18521=EDGE_LOOP('',(#47139,#47140,#47141,#47142));
#18522=EDGE_LOOP('',(#47143,#47144,#47145));
#18523=EDGE_LOOP('',(#47146,#47147,#47148,#47149));
#18524=EDGE_LOOP('',(#47150,#47151,#47152));
#18525=EDGE_LOOP('',(#47153,#47154,#47155,#47156));
#18526=EDGE_LOOP('',(#47157,#47158,#47159));
#18527=EDGE_LOOP('',(#47160,#47161,#47162,#47163));
#18528=EDGE_LOOP('',(#47164,#47165,#47166));
#18529=EDGE_LOOP('',(#47167,#47168,#47169,#47170));
#18530=EDGE_LOOP('',(#47171,#47172,#47173));
#18531=EDGE_LOOP('',(#47174,#47175,#47176,#47177));
#18532=EDGE_LOOP('',(#47178,#47179,#47180));
#18533=EDGE_LOOP('',(#47181,#47182,#47183,#47184));
#18534=EDGE_LOOP('',(#47185,#47186,#47187));
#18535=EDGE_LOOP('',(#47188,#47189,#47190,#47191));
#18536=EDGE_LOOP('',(#47192,#47193,#47194));
#18537=EDGE_LOOP('',(#47195,#47196,#47197,#47198));
#18538=EDGE_LOOP('',(#47199,#47200,#47201));
#18539=EDGE_LOOP('',(#47202,#47203,#47204,#47205));
#18540=EDGE_LOOP('',(#47206,#47207,#47208));
#18541=EDGE_LOOP('',(#47209,#47210,#47211,#47212));
#18542=EDGE_LOOP('',(#47213,#47214,#47215));
#18543=EDGE_LOOP('',(#47216,#47217,#47218,#47219));
#18544=EDGE_LOOP('',(#47220,#47221,#47222));
#18545=EDGE_LOOP('',(#47223,#47224,#47225,#47226));
#18546=EDGE_LOOP('',(#47227,#47228,#47229));
#18547=EDGE_LOOP('',(#47230,#47231,#47232,#47233));
#18548=EDGE_LOOP('',(#47234,#47235,#47236));
#18549=EDGE_LOOP('',(#47237,#47238,#47239,#47240));
#18550=EDGE_LOOP('',(#47241,#47242,#47243));
#18551=EDGE_LOOP('',(#47244,#47245,#47246,#47247));
#18552=EDGE_LOOP('',(#47248,#47249,#47250));
#18553=EDGE_LOOP('',(#47251,#47252,#47253,#47254));
#18554=EDGE_LOOP('',(#47255,#47256,#47257));
#18555=EDGE_LOOP('',(#47258,#47259,#47260,#47261));
#18556=EDGE_LOOP('',(#47262,#47263,#47264));
#18557=EDGE_LOOP('',(#47265,#47266,#47267,#47268));
#18558=EDGE_LOOP('',(#47269,#47270,#47271));
#18559=EDGE_LOOP('',(#47272,#47273,#47274,#47275));
#18560=EDGE_LOOP('',(#47276,#47277,#47278));
#18561=EDGE_LOOP('',(#47279,#47280,#47281,#47282));
#18562=EDGE_LOOP('',(#47283,#47284,#47285));
#18563=EDGE_LOOP('',(#47286,#47287,#47288,#47289));
#18564=EDGE_LOOP('',(#47290,#47291,#47292));
#18565=EDGE_LOOP('',(#47293,#47294,#47295,#47296));
#18566=EDGE_LOOP('',(#47297,#47298,#47299));
#18567=EDGE_LOOP('',(#47300,#47301,#47302,#47303));
#18568=EDGE_LOOP('',(#47304,#47305,#47306));
#18569=EDGE_LOOP('',(#47307,#47308,#47309));
#18570=EDGE_LOOP('',(#47310,#47311,#47312,#47313));
#18571=EDGE_LOOP('',(#47314,#47315,#47316,#47317));
#18572=EDGE_LOOP('',(#47318,#47319,#47320));
#18573=EDGE_LOOP('',(#47321,#47322,#47323));
#18574=EDGE_LOOP('',(#47324,#47325,#47326,#47327));
#18575=EDGE_LOOP('',(#47328,#47329,#47330,#47331));
#18576=EDGE_LOOP('',(#47332,#47333,#47334,#47335));
#18577=EDGE_LOOP('',(#47336,#47337,#47338,#47339));
#18578=EDGE_LOOP('',(#47340,#47341,#47342,#47343));
#18579=EDGE_LOOP('',(#47344,#47345,#47346,#47347));
#18580=EDGE_LOOP('',(#47348,#47349,#47350,#47351,#47352,#47353));
#18581=EDGE_LOOP('',(#47354));
#18582=EDGE_LOOP('',(#47355));
#18583=EDGE_LOOP('',(#47356,#47357,#47358,#47359,#47360,#47361));
#18584=EDGE_LOOP('',(#47362,#47363,#47364,#47365,#47366,#47367,#47368,#47369,
#47370,#47371,#47372,#47373,#47374,#47375,#47376,#47377,#47378,#47379,#47380,
#47381,#47382,#47383,#47384,#47385,#47386,#47387,#47388,#47389,#47390,#47391,
#47392,#47393,#47394,#47395,#47396,#47397,#47398,#47399,#47400,#47401,#47402,
#47403,#47404,#47405,#47406,#47407,#47408,#47409,#47410,#47411,#47412,#47413,
#47414,#47415,#47416,#47417,#47418,#47419,#47420,#47421,#47422,#47423,#47424,
#47425,#47426,#47427,#47428,#47429,#47430,#47431,#47432,#47433,#47434,#47435,
#47436,#47437,#47438,#47439,#47440,#47441,#47442,#47443,#47444,#47445,#47446,
#47447,#47448,#47449,#47450,#47451,#47452,#47453,#47454,#47455,#47456,#47457,
#47458,#47459,#47460,#47461,#47462,#47463,#47464,#47465,#47466,#47467,#47468,
#47469,#47470,#47471,#47472,#47473,#47474,#47475,#47476,#47477,#47478,#47479,
#47480,#47481,#47482,#47483,#47484,#47485,#47486,#47487,#47488,#47489,#47490,
#47491,#47492,#47493,#47494,#47495,#47496,#47497,#47498,#47499,#47500,#47501,
#47502,#47503,#47504,#47505,#47506,#47507,#47508,#47509));
#18585=EDGE_LOOP('',(#47510,#47511,#47512,#47513,#47514,#47515,#47516,#47517,
#47518,#47519,#47520,#47521,#47522,#47523,#47524,#47525,#47526,#47527,#47528,
#47529,#47530,#47531,#47532,#47533,#47534,#47535,#47536,#47537,#47538,#47539,
#47540,#47541,#47542,#47543,#47544,#47545,#47546,#47547,#47548,#47549,#47550,
#47551,#47552,#47553,#47554,#47555,#47556,#47557,#47558,#47559,#47560,#47561,
#47562,#47563,#47564,#47565,#47566,#47567,#47568,#47569,#47570,#47571,#47572,
#47573,#47574,#47575,#47576,#47577,#47578,#47579,#47580,#47581,#47582,#47583,
#47584,#47585));
#18586=EDGE_LOOP('',(#47586));
#18587=EDGE_LOOP('',(#47587,#47588,#47589,#47590,#47591,#47592));
#20154=CIRCLE('',#54860,2.942);
#20155=CIRCLE('',#54876,2.942);
#20156=CIRCLE('',#54878,2.37175);
#20157=CIRCLE('',#54894,2.942);
#20158=CIRCLE('',#54895,2.942);
#20159=CIRCLE('',#54897,2.942);
#20160=CIRCLE('',#54898,2.942);
#20161=CIRCLE('',#54899,2.37175);
#20162=CIRCLE('',#54902,2.942);
#20163=CIRCLE('',#54903,0.25);
#20164=CIRCLE('',#54904,3.192);
#20165=CIRCLE('',#54907,5.);
#20166=CIRCLE('',#54910,5.);
#20167=CIRCLE('',#54913,5.);
#20168=CIRCLE('',#54916,5.);
#20169=CIRCLE('',#54919,5.);
#20170=CIRCLE('',#54922,5.);
#20171=CIRCLE('',#54925,5.);
#20172=CIRCLE('',#54928,5.);
#20173=CIRCLE('',#54931,5.);
#20174=CIRCLE('',#54934,5.);
#20175=CIRCLE('',#54937,5.);
#20176=CIRCLE('',#54940,5.);
#20177=CIRCLE('',#54943,5.);
#20178=CIRCLE('',#54946,5.);
#20179=CIRCLE('',#54949,5.);
#20180=CIRCLE('',#54952,5.);
#20181=CIRCLE('',#54955,5.);
#20182=CIRCLE('',#54958,5.);
#20183=CIRCLE('',#54961,5.);
#20184=CIRCLE('',#54964,5.);
#20185=CIRCLE('',#54967,5.);
#20186=CIRCLE('',#54970,5.);
#20187=CIRCLE('',#54973,5.);
#20188=CIRCLE('',#54976,5.);
#20189=CIRCLE('',#54979,5.);
#20190=CIRCLE('',#54982,5.);
#20191=CIRCLE('',#54985,5.);
#20192=CIRCLE('',#54988,5.);
#20193=CIRCLE('',#54991,5.);
#20194=CIRCLE('',#54994,5.);
#20195=CIRCLE('',#54997,5.);
#20196=CIRCLE('',#55000,5.);
#20197=CIRCLE('',#55003,5.);
#20198=CIRCLE('',#55006,5.);
#20199=CIRCLE('',#55009,5.);
#20200=CIRCLE('',#55012,5.);
#20201=CIRCLE('',#55013,5.);
#20202=CIRCLE('',#55016,5.);
#20203=CIRCLE('',#55017,5.);
#20204=CIRCLE('',#55020,5.);
#20205=CIRCLE('',#55023,5.);
#20206=CIRCLE('',#55026,5.);
#20207=CIRCLE('',#55029,5.);
#20208=CIRCLE('',#55032,5.);
#20209=CIRCLE('',#55035,5.);
#20210=CIRCLE('',#55038,5.);
#20211=CIRCLE('',#55041,5.);
#20212=CIRCLE('',#55044,5.);
#20213=CIRCLE('',#55047,5.);
#20214=CIRCLE('',#55050,5.);
#20215=CIRCLE('',#55053,5.);
#20216=CIRCLE('',#55056,5.);
#20217=CIRCLE('',#55059,5.);
#20218=CIRCLE('',#55062,5.);
#20219=CIRCLE('',#55065,5.);
#20220=CIRCLE('',#55068,5.);
#20221=CIRCLE('',#55071,5.);
#20222=CIRCLE('',#55074,5.);
#20223=CIRCLE('',#55077,5.);
#20224=CIRCLE('',#55080,5.);
#20225=CIRCLE('',#55083,5.);
#20226=CIRCLE('',#55086,5.);
#20227=CIRCLE('',#55089,5.);
#20228=CIRCLE('',#55092,5.);
#20229=CIRCLE('',#55095,5.);
#20230=CIRCLE('',#55098,5.);
#20231=CIRCLE('',#55101,5.);
#20232=CIRCLE('',#55104,5.);
#20233=CIRCLE('',#55107,5.);
#20234=CIRCLE('',#55110,5.);
#20235=CIRCLE('',#55113,5.);
#20236=CIRCLE('',#55116,5.);
#20237=CIRCLE('',#55119,5.);
#20238=CIRCLE('',#55121,5.);
#20239=CIRCLE('',#55125,5.);
#20240=CIRCLE('',#55127,2.48346726553949);
#20241=CIRCLE('',#55136,2.4);
#20242=CIRCLE('',#55139,5.);
#20243=CIRCLE('',#55140,5.);
#20244=CIRCLE('',#55141,5.);
#20245=CIRCLE('',#55142,5.);
#20246=CIRCLE('',#55143,5.);
#20247=CIRCLE('',#55144,5.);
#20248=CIRCLE('',#55145,5.);
#20249=CIRCLE('',#55146,5.);
#20250=CIRCLE('',#55147,5.);
#20251=CIRCLE('',#55148,5.);
#20252=CIRCLE('',#55149,5.);
#20253=CIRCLE('',#55150,5.);
#20254=CIRCLE('',#55151,5.);
#20255=CIRCLE('',#55152,5.);
#20256=CIRCLE('',#55153,5.);
#20257=CIRCLE('',#55154,5.);
#20258=CIRCLE('',#55155,5.);
#20259=CIRCLE('',#55156,5.);
#20260=CIRCLE('',#55157,5.);
#20261=CIRCLE('',#55158,5.);
#20262=CIRCLE('',#55159,5.);
#20263=CIRCLE('',#55160,5.);
#20264=CIRCLE('',#55161,5.);
#20265=CIRCLE('',#55162,5.);
#20266=CIRCLE('',#55163,5.);
#20267=CIRCLE('',#55164,5.);
#20268=CIRCLE('',#55165,5.);
#20269=CIRCLE('',#55166,5.);
#20270=CIRCLE('',#55167,5.);
#20271=CIRCLE('',#55168,5.);
#20272=CIRCLE('',#55169,5.);
#20273=CIRCLE('',#55170,5.);
#20274=CIRCLE('',#55171,5.);
#20275=CIRCLE('',#55172,5.);
#20276=CIRCLE('',#55173,5.);
#20277=CIRCLE('',#55174,5.);
#20278=CIRCLE('',#55176,4.4);
#24844=VERTEX_POINT('',#87478);
#24845=VERTEX_POINT('',#87479);
#24846=VERTEX_POINT('',#87481);
#24847=VERTEX_POINT('',#87492);
#24848=VERTEX_POINT('',#87502);
#24849=VERTEX_POINT('',#87503);
#24850=VERTEX_POINT('',#87550);
#24851=VERTEX_POINT('',#87551);
#24852=VERTEX_POINT('',#87598);
#24853=VERTEX_POINT('',#87599);
#24854=VERTEX_POINT('',#87652);
#24855=VERTEX_POINT('',#87653);
#24856=VERTEX_POINT('',#87700);
#24857=VERTEX_POINT('',#87701);
#24858=VERTEX_POINT('',#87748);
#24859=VERTEX_POINT('',#87749);
#24860=VERTEX_POINT('',#87796);
#24861=VERTEX_POINT('',#87797);
#24862=VERTEX_POINT('',#87850);
#24863=VERTEX_POINT('',#87851);
#24864=VERTEX_POINT('',#87898);
#24865=VERTEX_POINT('',#87899);
#24866=VERTEX_POINT('',#87946);
#24867=VERTEX_POINT('',#87947);
#24868=VERTEX_POINT('',#88000);
#24869=VERTEX_POINT('',#88001);
#24870=VERTEX_POINT('',#88048);
#24871=VERTEX_POINT('',#88049);
#24872=VERTEX_POINT('',#88096);
#24873=VERTEX_POINT('',#88097);
#24874=VERTEX_POINT('',#88150);
#24875=VERTEX_POINT('',#88151);
#24876=VERTEX_POINT('',#88198);
#24877=VERTEX_POINT('',#88199);
#24878=VERTEX_POINT('',#88201);
#24879=VERTEX_POINT('',#88245);
#24880=VERTEX_POINT('',#88246);
#24881=VERTEX_POINT('',#88248);
#24882=VERTEX_POINT('',#88256);
#24883=VERTEX_POINT('',#88265);
#24884=VERTEX_POINT('',#88266);
#24885=VERTEX_POINT('',#88289);
#24886=VERTEX_POINT('',#88290);
#24887=VERTEX_POINT('',#88314);
#24888=VERTEX_POINT('',#88315);
#24889=VERTEX_POINT('',#88339);
#24890=VERTEX_POINT('',#88340);
#24891=VERTEX_POINT('',#88363);
#24892=VERTEX_POINT('',#88364);
#24893=VERTEX_POINT('',#88388);
#24894=VERTEX_POINT('',#88389);
#24895=VERTEX_POINT('',#88413);
#24896=VERTEX_POINT('',#88414);
#24897=VERTEX_POINT('',#88437);
#24898=VERTEX_POINT('',#88438);
#24899=VERTEX_POINT('',#88462);
#24900=VERTEX_POINT('',#88463);
#24901=VERTEX_POINT('',#88487);
#24902=VERTEX_POINT('',#88488);
#24903=VERTEX_POINT('',#88511);
#24904=VERTEX_POINT('',#88512);
#24905=VERTEX_POINT('',#88535);
#24906=VERTEX_POINT('',#88536);
#24907=VERTEX_POINT('',#88560);
#24908=VERTEX_POINT('',#88561);
#24909=VERTEX_POINT('',#88585);
#24910=VERTEX_POINT('',#88586);
#24911=VERTEX_POINT('',#88700);
#24912=VERTEX_POINT('',#88702);
#24913=VERTEX_POINT('',#89206);
#24914=VERTEX_POINT('',#89308);
#24915=VERTEX_POINT('',#89311);
#24916=VERTEX_POINT('',#89822);
#24917=VERTEX_POINT('',#89827);
#24918=VERTEX_POINT('',#89830);
#24919=VERTEX_POINT('',#89831);
#24920=VERTEX_POINT('',#89833);
#24921=VERTEX_POINT('',#89835);
#24922=VERTEX_POINT('',#89839);
#24923=VERTEX_POINT('',#89843);
#24924=VERTEX_POINT('',#89849);
#24925=VERTEX_POINT('',#89850);
#24926=VERTEX_POINT('',#89852);
#24927=VERTEX_POINT('',#89854);
#24928=VERTEX_POINT('',#89858);
#24929=VERTEX_POINT('',#89862);
#24930=VERTEX_POINT('',#89868);
#24931=VERTEX_POINT('',#89869);
#24932=VERTEX_POINT('',#89871);
#24933=VERTEX_POINT('',#89873);
#24934=VERTEX_POINT('',#89877);
#24935=VERTEX_POINT('',#89881);
#24936=VERTEX_POINT('',#89887);
#24937=VERTEX_POINT('',#89888);
#24938=VERTEX_POINT('',#89890);
#24939=VERTEX_POINT('',#89892);
#24940=VERTEX_POINT('',#89896);
#24941=VERTEX_POINT('',#89900);
#24942=VERTEX_POINT('',#89906);
#24943=VERTEX_POINT('',#89907);
#24944=VERTEX_POINT('',#89909);
#24945=VERTEX_POINT('',#89911);
#24946=VERTEX_POINT('',#89915);
#24947=VERTEX_POINT('',#89919);
#24948=VERTEX_POINT('',#89925);
#24949=VERTEX_POINT('',#89926);
#24950=VERTEX_POINT('',#89928);
#24951=VERTEX_POINT('',#89930);
#24952=VERTEX_POINT('',#89934);
#24953=VERTEX_POINT('',#89938);
#24954=VERTEX_POINT('',#89944);
#24955=VERTEX_POINT('',#89945);
#24956=VERTEX_POINT('',#89947);
#24957=VERTEX_POINT('',#89949);
#24958=VERTEX_POINT('',#89953);
#24959=VERTEX_POINT('',#89957);
#24960=VERTEX_POINT('',#89963);
#24961=VERTEX_POINT('',#89964);
#24962=VERTEX_POINT('',#89966);
#24963=VERTEX_POINT('',#89968);
#24964=VERTEX_POINT('',#89972);
#24965=VERTEX_POINT('',#89976);
#24966=VERTEX_POINT('',#89982);
#24967=VERTEX_POINT('',#89983);
#24968=VERTEX_POINT('',#89985);
#24969=VERTEX_POINT('',#89987);
#24970=VERTEX_POINT('',#89991);
#24971=VERTEX_POINT('',#89995);
#24972=VERTEX_POINT('',#90001);
#24973=VERTEX_POINT('',#90002);
#24974=VERTEX_POINT('',#90004);
#24975=VERTEX_POINT('',#90006);
#24976=VERTEX_POINT('',#90010);
#24977=VERTEX_POINT('',#90014);
#24978=VERTEX_POINT('',#90020);
#24979=VERTEX_POINT('',#90021);
#24980=VERTEX_POINT('',#90023);
#24981=VERTEX_POINT('',#90025);
#24982=VERTEX_POINT('',#90029);
#24983=VERTEX_POINT('',#90033);
#24984=VERTEX_POINT('',#90039);
#24985=VERTEX_POINT('',#90040);
#24986=VERTEX_POINT('',#90042);
#24987=VERTEX_POINT('',#90044);
#24988=VERTEX_POINT('',#90048);
#24989=VERTEX_POINT('',#90052);
#24990=VERTEX_POINT('',#90058);
#24991=VERTEX_POINT('',#90059);
#24992=VERTEX_POINT('',#90061);
#24993=VERTEX_POINT('',#90063);
#24994=VERTEX_POINT('',#90067);
#24995=VERTEX_POINT('',#90071);
#24996=VERTEX_POINT('',#90077);
#24997=VERTEX_POINT('',#90078);
#24998=VERTEX_POINT('',#90080);
#24999=VERTEX_POINT('',#90082);
#25000=VERTEX_POINT('',#90086);
#25001=VERTEX_POINT('',#90090);
#25002=VERTEX_POINT('',#90096);
#25003=VERTEX_POINT('',#90097);
#25004=VERTEX_POINT('',#90099);
#25005=VERTEX_POINT('',#90101);
#25006=VERTEX_POINT('',#90105);
#25007=VERTEX_POINT('',#90109);
#25008=VERTEX_POINT('',#90115);
#25009=VERTEX_POINT('',#90116);
#25010=VERTEX_POINT('',#90118);
#25011=VERTEX_POINT('',#90120);
#25012=VERTEX_POINT('',#90124);
#25013=VERTEX_POINT('',#90128);
#25014=VERTEX_POINT('',#90134);
#25015=VERTEX_POINT('',#90135);
#25016=VERTEX_POINT('',#90137);
#25017=VERTEX_POINT('',#90139);
#25018=VERTEX_POINT('',#90143);
#25019=VERTEX_POINT('',#90147);
#25020=VERTEX_POINT('',#90153);
#25021=VERTEX_POINT('',#90154);
#25022=VERTEX_POINT('',#90156);
#25023=VERTEX_POINT('',#90158);
#25024=VERTEX_POINT('',#90162);
#25025=VERTEX_POINT('',#90164);
#25026=VERTEX_POINT('',#90168);
#25027=VERTEX_POINT('',#90172);
#25028=VERTEX_POINT('',#90176);
#25029=VERTEX_POINT('',#90177);
#25030=VERTEX_POINT('',#90179);
#25031=VERTEX_POINT('',#90181);
#25032=VERTEX_POINT('',#90185);
#25033=VERTEX_POINT('',#90189);
#25034=VERTEX_POINT('',#90195);
#25035=VERTEX_POINT('',#90196);
#25036=VERTEX_POINT('',#90198);
#25037=VERTEX_POINT('',#90200);
#25038=VERTEX_POINT('',#90204);
#25039=VERTEX_POINT('',#90208);
#25040=VERTEX_POINT('',#90214);
#25041=VERTEX_POINT('',#90215);
#25042=VERTEX_POINT('',#90217);
#25043=VERTEX_POINT('',#90219);
#25044=VERTEX_POINT('',#90223);
#25045=VERTEX_POINT('',#90227);
#25046=VERTEX_POINT('',#90233);
#25047=VERTEX_POINT('',#90234);
#25048=VERTEX_POINT('',#90236);
#25049=VERTEX_POINT('',#90238);
#25050=VERTEX_POINT('',#90242);
#25051=VERTEX_POINT('',#90246);
#25052=VERTEX_POINT('',#90252);
#25053=VERTEX_POINT('',#90253);
#25054=VERTEX_POINT('',#90255);
#25055=VERTEX_POINT('',#90257);
#25056=VERTEX_POINT('',#90261);
#25057=VERTEX_POINT('',#90265);
#25058=VERTEX_POINT('',#90271);
#25059=VERTEX_POINT('',#90272);
#25060=VERTEX_POINT('',#90274);
#25061=VERTEX_POINT('',#90276);
#25062=VERTEX_POINT('',#90280);
#25063=VERTEX_POINT('',#90284);
#25064=VERTEX_POINT('',#90290);
#25065=VERTEX_POINT('',#90291);
#25066=VERTEX_POINT('',#90293);
#25067=VERTEX_POINT('',#90295);
#25068=VERTEX_POINT('',#90299);
#25069=VERTEX_POINT('',#90303);
#25070=VERTEX_POINT('',#90309);
#25071=VERTEX_POINT('',#90310);
#25072=VERTEX_POINT('',#90312);
#25073=VERTEX_POINT('',#90314);
#25074=VERTEX_POINT('',#90318);
#25075=VERTEX_POINT('',#90322);
#25076=VERTEX_POINT('',#90328);
#25077=VERTEX_POINT('',#90329);
#25078=VERTEX_POINT('',#90331);
#25079=VERTEX_POINT('',#90333);
#25080=VERTEX_POINT('',#90337);
#25081=VERTEX_POINT('',#90341);
#25082=VERTEX_POINT('',#90347);
#25083=VERTEX_POINT('',#90348);
#25084=VERTEX_POINT('',#90350);
#25085=VERTEX_POINT('',#90352);
#25086=VERTEX_POINT('',#90356);
#25087=VERTEX_POINT('',#90360);
#25088=VERTEX_POINT('',#90366);
#25089=VERTEX_POINT('',#90367);
#25090=VERTEX_POINT('',#90369);
#25091=VERTEX_POINT('',#90371);
#25092=VERTEX_POINT('',#90375);
#25093=VERTEX_POINT('',#90379);
#25094=VERTEX_POINT('',#90385);
#25095=VERTEX_POINT('',#90386);
#25096=VERTEX_POINT('',#90388);
#25097=VERTEX_POINT('',#90390);
#25098=VERTEX_POINT('',#90394);
#25099=VERTEX_POINT('',#90398);
#25100=VERTEX_POINT('',#90404);
#25101=VERTEX_POINT('',#90405);
#25102=VERTEX_POINT('',#90407);
#25103=VERTEX_POINT('',#90409);
#25104=VERTEX_POINT('',#90413);
#25105=VERTEX_POINT('',#90417);
#25106=VERTEX_POINT('',#90423);
#25107=VERTEX_POINT('',#90424);
#25108=VERTEX_POINT('',#90426);
#25109=VERTEX_POINT('',#90428);
#25110=VERTEX_POINT('',#90432);
#25111=VERTEX_POINT('',#90436);
#25112=VERTEX_POINT('',#90442);
#25113=VERTEX_POINT('',#90443);
#25114=VERTEX_POINT('',#90445);
#25115=VERTEX_POINT('',#90447);
#25116=VERTEX_POINT('',#90451);
#25117=VERTEX_POINT('',#90455);
#25118=VERTEX_POINT('',#90461);
#25119=VERTEX_POINT('',#90462);
#25120=VERTEX_POINT('',#90464);
#25121=VERTEX_POINT('',#90466);
#25122=VERTEX_POINT('',#90470);
#25123=VERTEX_POINT('',#90474);
#25124=VERTEX_POINT('',#90480);
#25125=VERTEX_POINT('',#90481);
#25126=VERTEX_POINT('',#90483);
#25127=VERTEX_POINT('',#90485);
#25128=VERTEX_POINT('',#90489);
#25129=VERTEX_POINT('',#90493);
#25130=VERTEX_POINT('',#90499);
#25131=VERTEX_POINT('',#90500);
#25132=VERTEX_POINT('',#90502);
#25133=VERTEX_POINT('',#90506);
#25134=VERTEX_POINT('',#90508);
#25135=VERTEX_POINT('',#90512);
#25136=VERTEX_POINT('',#90518);
#25137=VERTEX_POINT('',#90519);
#25138=VERTEX_POINT('',#90523);
#25139=VERTEX_POINT('',#90524);
#25140=VERTEX_POINT('',#90526);
#25141=VERTEX_POINT('',#90528);
#25142=VERTEX_POINT('',#90532);
#25143=VERTEX_POINT('',#90534);
#25144=VERTEX_POINT('',#90538);
#25145=VERTEX_POINT('',#90540);
#25146=VERTEX_POINT('',#90544);
#25147=VERTEX_POINT('',#90546);
#25148=VERTEX_POINT('',#90550);
#25149=VERTEX_POINT('',#90552);
#25150=VERTEX_POINT('',#90560);
#25151=VERTEX_POINT('',#90603);
#32159=EDGE_CURVE('',#24844,#24845,#6297,.T.);
#32160=EDGE_CURVE('',#24844,#24846,#550,.T.);
#32161=EDGE_CURVE('',#24846,#24847,#20154,.T.);
#32162=EDGE_CURVE('',#24847,#24845,#551,.T.);
#32163=EDGE_CURVE('',#24848,#24849,#6298,.T.);
#32164=EDGE_CURVE('',#24848,#24844,#552,.T.);
#32165=EDGE_CURVE('',#24845,#24849,#553,.T.);
#32166=EDGE_CURVE('',#24850,#24851,#6299,.T.);
#32167=EDGE_CURVE('',#24850,#24848,#554,.T.);
#32168=EDGE_CURVE('',#24849,#24851,#555,.T.);
#32169=EDGE_CURVE('',#24852,#24853,#6300,.T.);
#32170=EDGE_CURVE('',#24852,#24850,#556,.T.);
#32171=EDGE_CURVE('',#24851,#24853,#557,.T.);
#32172=EDGE_CURVE('',#24854,#24855,#6301,.T.);
#32173=EDGE_CURVE('',#24854,#24852,#558,.T.);
#32174=EDGE_CURVE('',#24853,#24855,#559,.T.);
#32175=EDGE_CURVE('',#24856,#24857,#6302,.T.);
#32176=EDGE_CURVE('',#24856,#24854,#560,.T.);
#32177=EDGE_CURVE('',#24855,#24857,#561,.T.);
#32178=EDGE_CURVE('',#24858,#24859,#6303,.T.);
#32179=EDGE_CURVE('',#24858,#24856,#562,.T.);
#32180=EDGE_CURVE('',#24857,#24859,#563,.T.);
#32181=EDGE_CURVE('',#24860,#24861,#6304,.T.);
#32182=EDGE_CURVE('',#24860,#24858,#564,.T.);
#32183=EDGE_CURVE('',#24859,#24861,#565,.T.);
#32184=EDGE_CURVE('',#24862,#24863,#6305,.T.);
#32185=EDGE_CURVE('',#24862,#24860,#566,.T.);
#32186=EDGE_CURVE('',#24861,#24863,#567,.T.);
#32187=EDGE_CURVE('',#24864,#24865,#6306,.T.);
#32188=EDGE_CURVE('',#24864,#24862,#568,.T.);
#32189=EDGE_CURVE('',#24863,#24865,#569,.T.);
#32190=EDGE_CURVE('',#24866,#24867,#6307,.T.);
#32191=EDGE_CURVE('',#24866,#24864,#570,.T.);
#32192=EDGE_CURVE('',#24865,#24867,#571,.T.);
#32193=EDGE_CURVE('',#24868,#24869,#6308,.T.);
#32194=EDGE_CURVE('',#24868,#24866,#572,.T.);
#32195=EDGE_CURVE('',#24867,#24869,#573,.T.);
#32196=EDGE_CURVE('',#24870,#24871,#6309,.T.);
#32197=EDGE_CURVE('',#24870,#24868,#574,.T.);
#32198=EDGE_CURVE('',#24869,#24871,#575,.T.);
#32199=EDGE_CURVE('',#24872,#24873,#6310,.T.);
#32200=EDGE_CURVE('',#24872,#24870,#576,.T.);
#32201=EDGE_CURVE('',#24871,#24873,#577,.T.);
#32202=EDGE_CURVE('',#24874,#24875,#6311,.T.);
#32203=EDGE_CURVE('',#24874,#24872,#578,.T.);
#32204=EDGE_CURVE('',#24873,#24875,#579,.T.);
#32205=EDGE_CURVE('',#24876,#24877,#6312,.T.);
#32206=EDGE_CURVE('',#24878,#24876,#20155,.T.);
#32207=EDGE_CURVE('',#24878,#24874,#580,.T.);
#32208=EDGE_CURVE('',#24875,#24877,#581,.T.);
#32209=EDGE_CURVE('',#24879,#24880,#6313,.T.);
#32210=EDGE_CURVE('',#24879,#24881,#582,.T.);
#32211=EDGE_CURVE('',#24882,#24881,#20156,.T.);
#32212=EDGE_CURVE('',#24880,#24882,#583,.T.);
#32213=EDGE_CURVE('',#24883,#24884,#6314,.T.);
#32214=EDGE_CURVE('',#24883,#24879,#584,.T.);
#32215=EDGE_CURVE('',#24884,#24880,#585,.T.);
#32216=EDGE_CURVE('',#24885,#24886,#6315,.T.);
#32217=EDGE_CURVE('',#24885,#24883,#586,.T.);
#32218=EDGE_CURVE('',#24886,#24884,#587,.T.);
#32219=EDGE_CURVE('',#24887,#24888,#6316,.T.);
#32220=EDGE_CURVE('',#24887,#24885,#588,.T.);
#32221=EDGE_CURVE('',#24888,#24886,#589,.T.);
#32222=EDGE_CURVE('',#24889,#24890,#6317,.T.);
#32223=EDGE_CURVE('',#24889,#24887,#590,.T.);
#32224=EDGE_CURVE('',#24890,#24888,#591,.T.);
#32225=EDGE_CURVE('',#24891,#24892,#6318,.T.);
#32226=EDGE_CURVE('',#24891,#24889,#592,.T.);
#32227=EDGE_CURVE('',#24892,#24890,#593,.T.);
#32228=EDGE_CURVE('',#24893,#24894,#6319,.T.);
#32229=EDGE_CURVE('',#24893,#24891,#594,.T.);
#32230=EDGE_CURVE('',#24894,#24892,#595,.T.);
#32231=EDGE_CURVE('',#24895,#24896,#6320,.T.);
#32232=EDGE_CURVE('',#24895,#24893,#596,.T.);
#32233=EDGE_CURVE('',#24896,#24894,#597,.T.);
#32234=EDGE_CURVE('',#24897,#24898,#6321,.T.);
#32235=EDGE_CURVE('',#24897,#24895,#598,.T.);
#32236=EDGE_CURVE('',#24898,#24896,#599,.T.);
#32237=EDGE_CURVE('',#24899,#24900,#6322,.T.);
#32238=EDGE_CURVE('',#24899,#24897,#600,.T.);
#32239=EDGE_CURVE('',#24900,#24898,#601,.T.);
#32240=EDGE_CURVE('',#24901,#24902,#6323,.T.);
#32241=EDGE_CURVE('',#24901,#24899,#602,.T.);
#32242=EDGE_CURVE('',#24902,#24900,#603,.T.);
#32243=EDGE_CURVE('',#24903,#24904,#6324,.T.);
#32244=EDGE_CURVE('',#24903,#24901,#604,.T.);
#32245=EDGE_CURVE('',#24904,#24902,#605,.T.);
#32246=EDGE_CURVE('',#24905,#24906,#6325,.T.);
#32247=EDGE_CURVE('',#24905,#24903,#606,.T.);
#32248=EDGE_CURVE('',#24906,#24904,#607,.T.);
#32249=EDGE_CURVE('',#24907,#24908,#6326,.T.);
#32250=EDGE_CURVE('',#24907,#24905,#608,.T.);
#32251=EDGE_CURVE('',#24908,#24906,#609,.T.);
#32252=EDGE_CURVE('',#24909,#24910,#6327,.T.);
#32253=EDGE_CURVE('',#24909,#24907,#610,.T.);
#32254=EDGE_CURVE('',#24910,#24908,#611,.T.);
#32255=EDGE_CURVE('',#24881,#24878,#612,.T.);
#32256=EDGE_CURVE('',#24911,#24878,#20157,.T.);
#32257=EDGE_CURVE('',#24912,#24911,#20158,.T.);
#32258=EDGE_CURVE('',#24912,#24882,#613,.T.);
#32259=EDGE_CURVE('',#24877,#24912,#614,.T.);
#32260=EDGE_CURVE('',#24913,#24847,#615,.T.);
#32261=EDGE_CURVE('',#24913,#24910,#616,.T.);
#32262=EDGE_CURVE('',#24847,#24914,#20159,.T.);
#32263=EDGE_CURVE('',#24914,#24846,#20160,.T.);
#32264=EDGE_CURVE('',#24846,#24915,#617,.T.);
#32265=EDGE_CURVE('',#24915,#24913,#20161,.T.);
#32266=EDGE_CURVE('',#24915,#24909,#618,.T.);
#32267=EDGE_CURVE('',#24876,#24912,#20162,.T.);
#32268=EDGE_CURVE('',#24911,#24916,#20163,.T.);
#32269=EDGE_CURVE('',#24916,#24916,#20164,.T.);
#32270=EDGE_CURVE('',#24917,#24917,#20165,.T.);
#32271=EDGE_CURVE('',#24918,#24919,#6328,.T.);
#32272=EDGE_CURVE('',#24918,#24920,#6329,.T.);
#32273=EDGE_CURVE('',#24920,#24921,#6330,.T.);
#32274=EDGE_CURVE('',#24921,#24919,#6331,.T.);
#32275=EDGE_CURVE('',#24919,#24922,#20166,.T.);
#32276=EDGE_CURVE('',#24922,#24921,#6332,.T.);
#32277=EDGE_CURVE('',#24922,#24923,#6333,.T.);
#32278=EDGE_CURVE('',#24920,#24923,#6334,.T.);
#32279=EDGE_CURVE('',#24923,#24918,#20167,.T.);
#32280=EDGE_CURVE('',#24924,#24925,#6335,.T.);
#32281=EDGE_CURVE('',#24924,#24926,#6336,.T.);
#32282=EDGE_CURVE('',#24926,#24927,#6337,.T.);
#32283=EDGE_CURVE('',#24927,#24925,#6338,.T.);
#32284=EDGE_CURVE('',#24925,#24928,#20168,.T.);
#32285=EDGE_CURVE('',#24928,#24927,#6339,.T.);
#32286=EDGE_CURVE('',#24928,#24929,#6340,.T.);
#32287=EDGE_CURVE('',#24926,#24929,#6341,.T.);
#32288=EDGE_CURVE('',#24929,#24924,#20169,.T.);
#32289=EDGE_CURVE('',#24930,#24931,#6342,.T.);
#32290=EDGE_CURVE('',#24930,#24932,#6343,.T.);
#32291=EDGE_CURVE('',#24932,#24933,#6344,.T.);
#32292=EDGE_CURVE('',#24933,#24931,#6345,.T.);
#32293=EDGE_CURVE('',#24931,#24934,#20170,.T.);
#32294=EDGE_CURVE('',#24934,#24933,#6346,.T.);
#32295=EDGE_CURVE('',#24934,#24935,#6347,.T.);
#32296=EDGE_CURVE('',#24932,#24935,#6348,.T.);
#32297=EDGE_CURVE('',#24935,#24930,#20171,.T.);
#32298=EDGE_CURVE('',#24936,#24937,#6349,.T.);
#32299=EDGE_CURVE('',#24936,#24938,#6350,.T.);
#32300=EDGE_CURVE('',#24938,#24939,#6351,.T.);
#32301=EDGE_CURVE('',#24939,#24937,#6352,.T.);
#32302=EDGE_CURVE('',#24937,#24940,#20172,.T.);
#32303=EDGE_CURVE('',#24940,#24939,#6353,.T.);
#32304=EDGE_CURVE('',#24940,#24941,#6354,.T.);
#32305=EDGE_CURVE('',#24938,#24941,#6355,.T.);
#32306=EDGE_CURVE('',#24941,#24936,#20173,.T.);
#32307=EDGE_CURVE('',#24942,#24943,#6356,.T.);
#32308=EDGE_CURVE('',#24942,#24944,#6357,.T.);
#32309=EDGE_CURVE('',#24944,#24945,#6358,.T.);
#32310=EDGE_CURVE('',#24945,#24943,#6359,.T.);
#32311=EDGE_CURVE('',#24943,#24946,#20174,.T.);
#32312=EDGE_CURVE('',#24946,#24945,#6360,.T.);
#32313=EDGE_CURVE('',#24946,#24947,#6361,.T.);
#32314=EDGE_CURVE('',#24944,#24947,#6362,.T.);
#32315=EDGE_CURVE('',#24947,#24942,#20175,.T.);
#32316=EDGE_CURVE('',#24948,#24949,#6363,.T.);
#32317=EDGE_CURVE('',#24948,#24950,#6364,.T.);
#32318=EDGE_CURVE('',#24950,#24951,#6365,.T.);
#32319=EDGE_CURVE('',#24951,#24949,#6366,.T.);
#32320=EDGE_CURVE('',#24949,#24952,#20176,.T.);
#32321=EDGE_CURVE('',#24952,#24951,#6367,.T.);
#32322=EDGE_CURVE('',#24952,#24953,#6368,.T.);
#32323=EDGE_CURVE('',#24950,#24953,#6369,.T.);
#32324=EDGE_CURVE('',#24953,#24948,#20177,.T.);
#32325=EDGE_CURVE('',#24954,#24955,#6370,.T.);
#32326=EDGE_CURVE('',#24954,#24956,#6371,.T.);
#32327=EDGE_CURVE('',#24956,#24957,#6372,.T.);
#32328=EDGE_CURVE('',#24957,#24955,#6373,.T.);
#32329=EDGE_CURVE('',#24955,#24958,#20178,.T.);
#32330=EDGE_CURVE('',#24958,#24957,#6374,.T.);
#32331=EDGE_CURVE('',#24958,#24959,#6375,.T.);
#32332=EDGE_CURVE('',#24956,#24959,#6376,.T.);
#32333=EDGE_CURVE('',#24959,#24954,#20179,.T.);
#32334=EDGE_CURVE('',#24960,#24961,#6377,.T.);
#32335=EDGE_CURVE('',#24960,#24962,#6378,.T.);
#32336=EDGE_CURVE('',#24962,#24963,#6379,.T.);
#32337=EDGE_CURVE('',#24963,#24961,#6380,.T.);
#32338=EDGE_CURVE('',#24961,#24964,#20180,.T.);
#32339=EDGE_CURVE('',#24964,#24963,#6381,.T.);
#32340=EDGE_CURVE('',#24964,#24965,#6382,.T.);
#32341=EDGE_CURVE('',#24962,#24965,#6383,.T.);
#32342=EDGE_CURVE('',#24965,#24960,#20181,.T.);
#32343=EDGE_CURVE('',#24966,#24967,#6384,.T.);
#32344=EDGE_CURVE('',#24966,#24968,#6385,.T.);
#32345=EDGE_CURVE('',#24968,#24969,#6386,.T.);
#32346=EDGE_CURVE('',#24969,#24967,#6387,.T.);
#32347=EDGE_CURVE('',#24967,#24970,#20182,.T.);
#32348=EDGE_CURVE('',#24970,#24969,#6388,.T.);
#32349=EDGE_CURVE('',#24970,#24971,#6389,.T.);
#32350=EDGE_CURVE('',#24968,#24971,#6390,.T.);
#32351=EDGE_CURVE('',#24971,#24966,#20183,.T.);
#32352=EDGE_CURVE('',#24972,#24973,#6391,.T.);
#32353=EDGE_CURVE('',#24972,#24974,#6392,.T.);
#32354=EDGE_CURVE('',#24974,#24975,#6393,.T.);
#32355=EDGE_CURVE('',#24975,#24973,#6394,.T.);
#32356=EDGE_CURVE('',#24973,#24976,#20184,.T.);
#32357=EDGE_CURVE('',#24976,#24975,#6395,.T.);
#32358=EDGE_CURVE('',#24976,#24977,#6396,.T.);
#32359=EDGE_CURVE('',#24974,#24977,#6397,.T.);
#32360=EDGE_CURVE('',#24977,#24972,#20185,.T.);
#32361=EDGE_CURVE('',#24978,#24979,#6398,.T.);
#32362=EDGE_CURVE('',#24978,#24980,#6399,.T.);
#32363=EDGE_CURVE('',#24980,#24981,#6400,.T.);
#32364=EDGE_CURVE('',#24981,#24979,#6401,.T.);
#32365=EDGE_CURVE('',#24979,#24982,#20186,.T.);
#32366=EDGE_CURVE('',#24982,#24981,#6402,.T.);
#32367=EDGE_CURVE('',#24982,#24983,#6403,.T.);
#32368=EDGE_CURVE('',#24980,#24983,#6404,.T.);
#32369=EDGE_CURVE('',#24983,#24978,#20187,.T.);
#32370=EDGE_CURVE('',#24984,#24985,#6405,.T.);
#32371=EDGE_CURVE('',#24984,#24986,#6406,.T.);
#32372=EDGE_CURVE('',#24986,#24987,#6407,.T.);
#32373=EDGE_CURVE('',#24987,#24985,#6408,.T.);
#32374=EDGE_CURVE('',#24985,#24988,#20188,.T.);
#32375=EDGE_CURVE('',#24988,#24987,#6409,.T.);
#32376=EDGE_CURVE('',#24988,#24989,#6410,.T.);
#32377=EDGE_CURVE('',#24986,#24989,#6411,.T.);
#32378=EDGE_CURVE('',#24989,#24984,#20189,.T.);
#32379=EDGE_CURVE('',#24990,#24991,#6412,.T.);
#32380=EDGE_CURVE('',#24990,#24992,#6413,.T.);
#32381=EDGE_CURVE('',#24992,#24993,#6414,.T.);
#32382=EDGE_CURVE('',#24993,#24991,#6415,.T.);
#32383=EDGE_CURVE('',#24991,#24994,#20190,.T.);
#32384=EDGE_CURVE('',#24994,#24993,#6416,.T.);
#32385=EDGE_CURVE('',#24994,#24995,#6417,.T.);
#32386=EDGE_CURVE('',#24992,#24995,#6418,.T.);
#32387=EDGE_CURVE('',#24995,#24990,#20191,.T.);
#32388=EDGE_CURVE('',#24996,#24997,#6419,.T.);
#32389=EDGE_CURVE('',#24996,#24998,#6420,.T.);
#32390=EDGE_CURVE('',#24998,#24999,#6421,.T.);
#32391=EDGE_CURVE('',#24999,#24997,#6422,.T.);
#32392=EDGE_CURVE('',#24997,#25000,#20192,.T.);
#32393=EDGE_CURVE('',#25000,#24999,#6423,.T.);
#32394=EDGE_CURVE('',#25000,#25001,#6424,.T.);
#32395=EDGE_CURVE('',#24998,#25001,#6425,.T.);
#32396=EDGE_CURVE('',#25001,#24996,#20193,.T.);
#32397=EDGE_CURVE('',#25002,#25003,#6426,.T.);
#32398=EDGE_CURVE('',#25002,#25004,#6427,.T.);
#32399=EDGE_CURVE('',#25004,#25005,#6428,.T.);
#32400=EDGE_CURVE('',#25005,#25003,#6429,.T.);
#32401=EDGE_CURVE('',#25003,#25006,#20194,.T.);
#32402=EDGE_CURVE('',#25006,#25005,#6430,.T.);
#32403=EDGE_CURVE('',#25006,#25007,#6431,.T.);
#32404=EDGE_CURVE('',#25004,#25007,#6432,.T.);
#32405=EDGE_CURVE('',#25007,#25002,#20195,.T.);
#32406=EDGE_CURVE('',#25008,#25009,#6433,.T.);
#32407=EDGE_CURVE('',#25008,#25010,#6434,.T.);
#32408=EDGE_CURVE('',#25010,#25011,#6435,.T.);
#32409=EDGE_CURVE('',#25011,#25009,#6436,.T.);
#32410=EDGE_CURVE('',#25009,#25012,#20196,.T.);
#32411=EDGE_CURVE('',#25012,#25011,#6437,.T.);
#32412=EDGE_CURVE('',#25012,#25013,#6438,.T.);
#32413=EDGE_CURVE('',#25010,#25013,#6439,.T.);
#32414=EDGE_CURVE('',#25013,#25008,#20197,.T.);
#32415=EDGE_CURVE('',#25014,#25015,#6440,.T.);
#32416=EDGE_CURVE('',#25014,#25016,#6441,.T.);
#32417=EDGE_CURVE('',#25016,#25017,#6442,.T.);
#32418=EDGE_CURVE('',#25017,#25015,#6443,.T.);
#32419=EDGE_CURVE('',#25015,#25018,#20198,.T.);
#32420=EDGE_CURVE('',#25018,#25017,#6444,.T.);
#32421=EDGE_CURVE('',#25018,#25019,#6445,.T.);
#32422=EDGE_CURVE('',#25016,#25019,#6446,.T.);
#32423=EDGE_CURVE('',#25019,#25014,#20199,.T.);
#32424=EDGE_CURVE('',#25020,#25021,#6447,.T.);
#32425=EDGE_CURVE('',#25020,#25022,#6448,.T.);
#32426=EDGE_CURVE('',#25022,#25023,#6449,.T.);
#32427=EDGE_CURVE('',#25023,#25021,#6450,.T.);
#32428=EDGE_CURVE('',#25021,#25024,#20200,.T.);
#32429=EDGE_CURVE('',#25025,#25023,#6451,.T.);
#32430=EDGE_CURVE('',#25024,#25025,#20201,.T.);
#32431=EDGE_CURVE('',#25025,#25026,#6452,.T.);
#32432=EDGE_CURVE('',#25022,#25026,#6453,.T.);
#32433=EDGE_CURVE('',#25026,#25027,#20202,.T.);
#32434=EDGE_CURVE('',#25027,#25020,#20203,.T.);
#32435=EDGE_CURVE('',#25028,#25029,#6454,.T.);
#32436=EDGE_CURVE('',#25028,#25030,#6455,.T.);
#32437=EDGE_CURVE('',#25030,#25031,#6456,.T.);
#32438=EDGE_CURVE('',#25031,#25029,#6457,.T.);
#32439=EDGE_CURVE('',#25029,#25032,#20204,.T.);
#32440=EDGE_CURVE('',#25032,#25031,#6458,.T.);
#32441=EDGE_CURVE('',#25032,#25033,#6459,.T.);
#32442=EDGE_CURVE('',#25030,#25033,#6460,.T.);
#32443=EDGE_CURVE('',#25033,#25028,#20205,.T.);
#32444=EDGE_CURVE('',#25034,#25035,#6461,.T.);
#32445=EDGE_CURVE('',#25034,#25036,#6462,.T.);
#32446=EDGE_CURVE('',#25036,#25037,#6463,.T.);
#32447=EDGE_CURVE('',#25037,#25035,#6464,.T.);
#32448=EDGE_CURVE('',#25035,#25038,#20206,.T.);
#32449=EDGE_CURVE('',#25038,#25037,#6465,.T.);
#32450=EDGE_CURVE('',#25038,#25039,#6466,.T.);
#32451=EDGE_CURVE('',#25036,#25039,#6467,.T.);
#32452=EDGE_CURVE('',#25039,#25034,#20207,.T.);
#32453=EDGE_CURVE('',#25040,#25041,#6468,.T.);
#32454=EDGE_CURVE('',#25040,#25042,#6469,.T.);
#32455=EDGE_CURVE('',#25042,#25043,#6470,.T.);
#32456=EDGE_CURVE('',#25043,#25041,#6471,.T.);
#32457=EDGE_CURVE('',#25041,#25044,#20208,.T.);
#32458=EDGE_CURVE('',#25044,#25043,#6472,.T.);
#32459=EDGE_CURVE('',#25044,#25045,#6473,.T.);
#32460=EDGE_CURVE('',#25042,#25045,#6474,.T.);
#32461=EDGE_CURVE('',#25045,#25040,#20209,.T.);
#32462=EDGE_CURVE('',#25046,#25047,#6475,.T.);
#32463=EDGE_CURVE('',#25046,#25048,#6476,.T.);
#32464=EDGE_CURVE('',#25048,#25049,#6477,.T.);
#32465=EDGE_CURVE('',#25049,#25047,#6478,.T.);
#32466=EDGE_CURVE('',#25047,#25050,#20210,.T.);
#32467=EDGE_CURVE('',#25050,#25049,#6479,.T.);
#32468=EDGE_CURVE('',#25050,#25051,#6480,.T.);
#32469=EDGE_CURVE('',#25048,#25051,#6481,.T.);
#32470=EDGE_CURVE('',#25051,#25046,#20211,.T.);
#32471=EDGE_CURVE('',#25052,#25053,#6482,.T.);
#32472=EDGE_CURVE('',#25052,#25054,#6483,.T.);
#32473=EDGE_CURVE('',#25054,#25055,#6484,.T.);
#32474=EDGE_CURVE('',#25055,#25053,#6485,.T.);
#32475=EDGE_CURVE('',#25053,#25056,#20212,.T.);
#32476=EDGE_CURVE('',#25056,#25055,#6486,.T.);
#32477=EDGE_CURVE('',#25056,#25057,#6487,.T.);
#32478=EDGE_CURVE('',#25054,#25057,#6488,.T.);
#32479=EDGE_CURVE('',#25057,#25052,#20213,.T.);
#32480=EDGE_CURVE('',#25058,#25059,#6489,.T.);
#32481=EDGE_CURVE('',#25058,#25060,#6490,.T.);
#32482=EDGE_CURVE('',#25060,#25061,#6491,.T.);
#32483=EDGE_CURVE('',#25061,#25059,#6492,.T.);
#32484=EDGE_CURVE('',#25059,#25062,#20214,.T.);
#32485=EDGE_CURVE('',#25062,#25061,#6493,.T.);
#32486=EDGE_CURVE('',#25062,#25063,#6494,.T.);
#32487=EDGE_CURVE('',#25060,#25063,#6495,.T.);
#32488=EDGE_CURVE('',#25063,#25058,#20215,.T.);
#32489=EDGE_CURVE('',#25064,#25065,#6496,.T.);
#32490=EDGE_CURVE('',#25064,#25066,#6497,.T.);
#32491=EDGE_CURVE('',#25066,#25067,#6498,.T.);
#32492=EDGE_CURVE('',#25067,#25065,#6499,.T.);
#32493=EDGE_CURVE('',#25065,#25068,#20216,.T.);
#32494=EDGE_CURVE('',#25068,#25067,#6500,.T.);
#32495=EDGE_CURVE('',#25068,#25069,#6501,.T.);
#32496=EDGE_CURVE('',#25066,#25069,#6502,.T.);
#32497=EDGE_CURVE('',#25069,#25064,#20217,.T.);
#32498=EDGE_CURVE('',#25070,#25071,#6503,.T.);
#32499=EDGE_CURVE('',#25070,#25072,#6504,.T.);
#32500=EDGE_CURVE('',#25072,#25073,#6505,.T.);
#32501=EDGE_CURVE('',#25073,#25071,#6506,.T.);
#32502=EDGE_CURVE('',#25071,#25074,#20218,.T.);
#32503=EDGE_CURVE('',#25074,#25073,#6507,.T.);
#32504=EDGE_CURVE('',#25074,#25075,#6508,.T.);
#32505=EDGE_CURVE('',#25072,#25075,#6509,.T.);
#32506=EDGE_CURVE('',#25075,#25070,#20219,.T.);
#32507=EDGE_CURVE('',#25076,#25077,#6510,.T.);
#32508=EDGE_CURVE('',#25076,#25078,#6511,.T.);
#32509=EDGE_CURVE('',#25078,#25079,#6512,.T.);
#32510=EDGE_CURVE('',#25079,#25077,#6513,.T.);
#32511=EDGE_CURVE('',#25077,#25080,#20220,.T.);
#32512=EDGE_CURVE('',#25080,#25079,#6514,.T.);
#32513=EDGE_CURVE('',#25080,#25081,#6515,.T.);
#32514=EDGE_CURVE('',#25078,#25081,#6516,.T.);
#32515=EDGE_CURVE('',#25081,#25076,#20221,.T.);
#32516=EDGE_CURVE('',#25082,#25083,#6517,.T.);
#32517=EDGE_CURVE('',#25082,#25084,#6518,.T.);
#32518=EDGE_CURVE('',#25084,#25085,#6519,.T.);
#32519=EDGE_CURVE('',#25085,#25083,#6520,.T.);
#32520=EDGE_CURVE('',#25083,#25086,#20222,.T.);
#32521=EDGE_CURVE('',#25086,#25085,#6521,.T.);
#32522=EDGE_CURVE('',#25086,#25087,#6522,.T.);
#32523=EDGE_CURVE('',#25084,#25087,#6523,.T.);
#32524=EDGE_CURVE('',#25087,#25082,#20223,.T.);
#32525=EDGE_CURVE('',#25088,#25089,#6524,.T.);
#32526=EDGE_CURVE('',#25088,#25090,#6525,.T.);
#32527=EDGE_CURVE('',#25090,#25091,#6526,.T.);
#32528=EDGE_CURVE('',#25091,#25089,#6527,.T.);
#32529=EDGE_CURVE('',#25089,#25092,#20224,.T.);
#32530=EDGE_CURVE('',#25092,#25091,#6528,.T.);
#32531=EDGE_CURVE('',#25092,#25093,#6529,.T.);
#32532=EDGE_CURVE('',#25090,#25093,#6530,.T.);
#32533=EDGE_CURVE('',#25093,#25088,#20225,.T.);
#32534=EDGE_CURVE('',#25094,#25095,#6531,.T.);
#32535=EDGE_CURVE('',#25094,#25096,#6532,.T.);
#32536=EDGE_CURVE('',#25096,#25097,#6533,.T.);
#32537=EDGE_CURVE('',#25097,#25095,#6534,.T.);
#32538=EDGE_CURVE('',#25095,#25098,#20226,.T.);
#32539=EDGE_CURVE('',#25098,#25097,#6535,.T.);
#32540=EDGE_CURVE('',#25098,#25099,#6536,.T.);
#32541=EDGE_CURVE('',#25096,#25099,#6537,.T.);
#32542=EDGE_CURVE('',#25099,#25094,#20227,.T.);
#32543=EDGE_CURVE('',#25100,#25101,#6538,.T.);
#32544=EDGE_CURVE('',#25100,#25102,#6539,.T.);
#32545=EDGE_CURVE('',#25102,#25103,#6540,.T.);
#32546=EDGE_CURVE('',#25103,#25101,#6541,.T.);
#32547=EDGE_CURVE('',#25101,#25104,#20228,.T.);
#32548=EDGE_CURVE('',#25104,#25103,#6542,.T.);
#32549=EDGE_CURVE('',#25104,#25105,#6543,.T.);
#32550=EDGE_CURVE('',#25102,#25105,#6544,.T.);
#32551=EDGE_CURVE('',#25105,#25100,#20229,.T.);
#32552=EDGE_CURVE('',#25106,#25107,#6545,.T.);
#32553=EDGE_CURVE('',#25106,#25108,#6546,.T.);
#32554=EDGE_CURVE('',#25108,#25109,#6547,.T.);
#32555=EDGE_CURVE('',#25109,#25107,#6548,.T.);
#32556=EDGE_CURVE('',#25107,#25110,#20230,.T.);
#32557=EDGE_CURVE('',#25110,#25109,#6549,.T.);
#32558=EDGE_CURVE('',#25110,#25111,#6550,.T.);
#32559=EDGE_CURVE('',#25108,#25111,#6551,.T.);
#32560=EDGE_CURVE('',#25111,#25106,#20231,.T.);
#32561=EDGE_CURVE('',#25112,#25113,#6552,.T.);
#32562=EDGE_CURVE('',#25112,#25114,#6553,.T.);
#32563=EDGE_CURVE('',#25114,#25115,#6554,.T.);
#32564=EDGE_CURVE('',#25115,#25113,#6555,.T.);
#32565=EDGE_CURVE('',#25113,#25116,#20232,.T.);
#32566=EDGE_CURVE('',#25116,#25115,#6556,.T.);
#32567=EDGE_CURVE('',#25116,#25117,#6557,.T.);
#32568=EDGE_CURVE('',#25114,#25117,#6558,.T.);
#32569=EDGE_CURVE('',#25117,#25112,#20233,.T.);
#32570=EDGE_CURVE('',#25118,#25119,#6559,.T.);
#32571=EDGE_CURVE('',#25118,#25120,#6560,.T.);
#32572=EDGE_CURVE('',#25120,#25121,#6561,.T.);
#32573=EDGE_CURVE('',#25121,#25119,#6562,.T.);
#32574=EDGE_CURVE('',#25119,#25122,#20234,.T.);
#32575=EDGE_CURVE('',#25122,#25121,#6563,.T.);
#32576=EDGE_CURVE('',#25122,#25123,#6564,.T.);
#32577=EDGE_CURVE('',#25120,#25123,#6565,.T.);
#32578=EDGE_CURVE('',#25123,#25118,#20235,.T.);
#32579=EDGE_CURVE('',#25124,#25125,#6566,.T.);
#32580=EDGE_CURVE('',#25124,#25126,#6567,.T.);
#32581=EDGE_CURVE('',#25126,#25127,#6568,.T.);
#32582=EDGE_CURVE('',#25127,#25125,#6569,.T.);
#32583=EDGE_CURVE('',#25125,#25128,#20236,.T.);
#32584=EDGE_CURVE('',#25128,#25127,#6570,.T.);
#32585=EDGE_CURVE('',#25128,#25129,#6571,.T.);
#32586=EDGE_CURVE('',#25126,#25129,#6572,.T.);
#32587=EDGE_CURVE('',#25129,#25124,#20237,.T.);
#32588=EDGE_CURVE('',#25130,#25131,#20238,.T.);
#32589=EDGE_CURVE('',#25132,#25130,#6573,.T.);
#32590=EDGE_CURVE('',#25131,#25132,#6574,.T.);
#32591=EDGE_CURVE('',#25133,#25130,#6575,.T.);
#32592=EDGE_CURVE('',#25133,#25134,#6576,.T.);
#32593=EDGE_CURVE('',#25134,#25132,#6577,.T.);
#32594=EDGE_CURVE('',#25131,#25135,#6578,.T.);
#32595=EDGE_CURVE('',#25134,#25135,#6579,.T.);
#32596=EDGE_CURVE('',#25135,#25133,#20239,.T.);
#32597=EDGE_CURVE('',#25136,#25137,#6580,.T.);
#32598=EDGE_CURVE('',#25137,#25137,#20240,.T.);
#32599=EDGE_CURVE('',#25138,#25139,#6581,.T.);
#32600=EDGE_CURVE('',#25140,#25138,#6582,.T.);
#32601=EDGE_CURVE('',#25141,#25140,#6583,.T.);
#32602=EDGE_CURVE('',#25141,#25139,#6584,.T.);
#32603=EDGE_CURVE('',#25139,#25142,#6585,.T.);
#32604=EDGE_CURVE('',#25143,#25141,#6586,.T.);
#32605=EDGE_CURVE('',#25143,#25142,#6587,.T.);
#32606=EDGE_CURVE('',#25142,#25144,#6588,.T.);
#32607=EDGE_CURVE('',#25145,#25143,#6589,.T.);
#32608=EDGE_CURVE('',#25145,#25144,#6590,.T.);
#32609=EDGE_CURVE('',#25144,#25146,#6591,.T.);
#32610=EDGE_CURVE('',#25147,#25145,#6592,.T.);
#32611=EDGE_CURVE('',#25147,#25146,#6593,.T.);
#32612=EDGE_CURVE('',#25146,#25148,#6594,.T.);
#32613=EDGE_CURVE('',#25149,#25147,#6595,.T.);
#32614=EDGE_CURVE('',#25149,#25148,#6596,.T.);
#32615=EDGE_CURVE('',#25148,#25138,#6597,.T.);
#32616=EDGE_CURVE('',#25140,#25149,#6598,.T.);
#32617=EDGE_CURVE('',#25150,#25150,#20241,.T.);
#32618=EDGE_CURVE('',#24914,#25150,#6599,.T.);
#32619=EDGE_CURVE('',#24928,#24919,#20242,.T.);
#32620=EDGE_CURVE('',#24934,#24925,#20243,.T.);
#32621=EDGE_CURVE('',#24940,#24931,#20244,.T.);
#32622=EDGE_CURVE('',#24946,#24937,#20245,.T.);
#32623=EDGE_CURVE('',#24952,#24943,#20246,.T.);
#32624=EDGE_CURVE('',#24958,#24949,#20247,.T.);
#32625=EDGE_CURVE('',#24964,#24955,#20248,.T.);
#32626=EDGE_CURVE('',#24970,#24961,#20249,.T.);
#32627=EDGE_CURVE('',#24976,#24967,#20250,.T.);
#32628=EDGE_CURVE('',#24982,#24973,#20251,.T.);
#32629=EDGE_CURVE('',#24988,#24979,#20252,.T.);
#32630=EDGE_CURVE('',#24994,#24985,#20253,.T.);
#32631=EDGE_CURVE('',#25000,#24991,#20254,.T.);
#32632=EDGE_CURVE('',#25006,#24997,#20255,.T.);
#32633=EDGE_CURVE('',#25012,#25003,#20256,.T.);
#32634=EDGE_CURVE('',#25018,#25009,#20257,.T.);
#32635=EDGE_CURVE('',#25025,#25015,#20258,.T.);
#32636=EDGE_CURVE('',#25027,#24917,#6600,.T.);
#32637=EDGE_CURVE('',#25032,#25021,#20259,.T.);
#32638=EDGE_CURVE('',#25038,#25029,#20260,.T.);
#32639=EDGE_CURVE('',#25044,#25035,#20261,.T.);
#32640=EDGE_CURVE('',#25050,#25041,#20262,.T.);
#32641=EDGE_CURVE('',#25056,#25047,#20263,.T.);
#32642=EDGE_CURVE('',#25062,#25053,#20264,.T.);
#32643=EDGE_CURVE('',#25068,#25059,#20265,.T.);
#32644=EDGE_CURVE('',#25074,#25065,#20266,.T.);
#32645=EDGE_CURVE('',#25080,#25071,#20267,.T.);
#32646=EDGE_CURVE('',#25086,#25077,#20268,.T.);
#32647=EDGE_CURVE('',#25092,#25083,#20269,.T.);
#32648=EDGE_CURVE('',#25098,#25089,#20270,.T.);
#32649=EDGE_CURVE('',#25104,#25095,#20271,.T.);
#32650=EDGE_CURVE('',#25110,#25101,#20272,.T.);
#32651=EDGE_CURVE('',#25116,#25107,#20273,.T.);
#32652=EDGE_CURVE('',#25122,#25113,#20274,.T.);
#32653=EDGE_CURVE('',#25128,#25119,#20275,.T.);
#32654=EDGE_CURVE('',#25131,#25125,#20276,.T.);
#32655=EDGE_CURVE('',#24922,#25130,#20277,.T.);
#32656=EDGE_CURVE('',#25151,#25151,#20278,.T.);
#32657=EDGE_CURVE('',#25151,#25024,#6601,.T.);
#46595=ORIENTED_EDGE('',*,*,#32159,.F.);
#46596=ORIENTED_EDGE('',*,*,#32160,.T.);
#46597=ORIENTED_EDGE('',*,*,#32161,.T.);
#46598=ORIENTED_EDGE('',*,*,#32162,.T.);
#46599=ORIENTED_EDGE('',*,*,#32163,.F.);
#46600=ORIENTED_EDGE('',*,*,#32164,.T.);
#46601=ORIENTED_EDGE('',*,*,#32159,.T.);
#46602=ORIENTED_EDGE('',*,*,#32165,.T.);
#46603=ORIENTED_EDGE('',*,*,#32166,.F.);
#46604=ORIENTED_EDGE('',*,*,#32167,.T.);
#46605=ORIENTED_EDGE('',*,*,#32163,.T.);
#46606=ORIENTED_EDGE('',*,*,#32168,.T.);
#46607=ORIENTED_EDGE('',*,*,#32169,.F.);
#46608=ORIENTED_EDGE('',*,*,#32170,.T.);
#46609=ORIENTED_EDGE('',*,*,#32166,.T.);
#46610=ORIENTED_EDGE('',*,*,#32171,.T.);
#46611=ORIENTED_EDGE('',*,*,#32172,.F.);
#46612=ORIENTED_EDGE('',*,*,#32173,.T.);
#46613=ORIENTED_EDGE('',*,*,#32169,.T.);
#46614=ORIENTED_EDGE('',*,*,#32174,.T.);
#46615=ORIENTED_EDGE('',*,*,#32175,.F.);
#46616=ORIENTED_EDGE('',*,*,#32176,.T.);
#46617=ORIENTED_EDGE('',*,*,#32172,.T.);
#46618=ORIENTED_EDGE('',*,*,#32177,.T.);
#46619=ORIENTED_EDGE('',*,*,#32178,.F.);
#46620=ORIENTED_EDGE('',*,*,#32179,.T.);
#46621=ORIENTED_EDGE('',*,*,#32175,.T.);
#46622=ORIENTED_EDGE('',*,*,#32180,.T.);
#46623=ORIENTED_EDGE('',*,*,#32181,.F.);
#46624=ORIENTED_EDGE('',*,*,#32182,.T.);
#46625=ORIENTED_EDGE('',*,*,#32178,.T.);
#46626=ORIENTED_EDGE('',*,*,#32183,.T.);
#46627=ORIENTED_EDGE('',*,*,#32184,.F.);
#46628=ORIENTED_EDGE('',*,*,#32185,.T.);
#46629=ORIENTED_EDGE('',*,*,#32181,.T.);
#46630=ORIENTED_EDGE('',*,*,#32186,.T.);
#46631=ORIENTED_EDGE('',*,*,#32187,.F.);
#46632=ORIENTED_EDGE('',*,*,#32188,.T.);
#46633=ORIENTED_EDGE('',*,*,#32184,.T.);
#46634=ORIENTED_EDGE('',*,*,#32189,.T.);
#46635=ORIENTED_EDGE('',*,*,#32190,.F.);
#46636=ORIENTED_EDGE('',*,*,#32191,.T.);
#46637=ORIENTED_EDGE('',*,*,#32187,.T.);
#46638=ORIENTED_EDGE('',*,*,#32192,.T.);
#46639=ORIENTED_EDGE('',*,*,#32193,.F.);
#46640=ORIENTED_EDGE('',*,*,#32194,.T.);
#46641=ORIENTED_EDGE('',*,*,#32190,.T.);
#46642=ORIENTED_EDGE('',*,*,#32195,.T.);
#46643=ORIENTED_EDGE('',*,*,#32196,.F.);
#46644=ORIENTED_EDGE('',*,*,#32197,.T.);
#46645=ORIENTED_EDGE('',*,*,#32193,.T.);
#46646=ORIENTED_EDGE('',*,*,#32198,.T.);
#46647=ORIENTED_EDGE('',*,*,#32199,.F.);
#46648=ORIENTED_EDGE('',*,*,#32200,.T.);
#46649=ORIENTED_EDGE('',*,*,#32196,.T.);
#46650=ORIENTED_EDGE('',*,*,#32201,.T.);
#46651=ORIENTED_EDGE('',*,*,#32202,.F.);
#46652=ORIENTED_EDGE('',*,*,#32203,.T.);
#46653=ORIENTED_EDGE('',*,*,#32199,.T.);
#46654=ORIENTED_EDGE('',*,*,#32204,.T.);
#46655=ORIENTED_EDGE('',*,*,#32205,.F.);
#46656=ORIENTED_EDGE('',*,*,#32206,.F.);
#46657=ORIENTED_EDGE('',*,*,#32207,.T.);
#46658=ORIENTED_EDGE('',*,*,#32202,.T.);
#46659=ORIENTED_EDGE('',*,*,#32208,.T.);
#46660=ORIENTED_EDGE('',*,*,#32209,.F.);
#46661=ORIENTED_EDGE('',*,*,#32210,.T.);
#46662=ORIENTED_EDGE('',*,*,#32211,.F.);
#46663=ORIENTED_EDGE('',*,*,#32212,.F.);
#46664=ORIENTED_EDGE('',*,*,#32213,.F.);
#46665=ORIENTED_EDGE('',*,*,#32214,.T.);
#46666=ORIENTED_EDGE('',*,*,#32209,.T.);
#46667=ORIENTED_EDGE('',*,*,#32215,.F.);
#46668=ORIENTED_EDGE('',*,*,#32216,.F.);
#46669=ORIENTED_EDGE('',*,*,#32217,.T.);
#46670=ORIENTED_EDGE('',*,*,#32213,.T.);
#46671=ORIENTED_EDGE('',*,*,#32218,.F.);
#46672=ORIENTED_EDGE('',*,*,#32219,.F.);
#46673=ORIENTED_EDGE('',*,*,#32220,.T.);
#46674=ORIENTED_EDGE('',*,*,#32216,.T.);
#46675=ORIENTED_EDGE('',*,*,#32221,.F.);
#46676=ORIENTED_EDGE('',*,*,#32222,.F.);
#46677=ORIENTED_EDGE('',*,*,#32223,.T.);
#46678=ORIENTED_EDGE('',*,*,#32219,.T.);
#46679=ORIENTED_EDGE('',*,*,#32224,.F.);
#46680=ORIENTED_EDGE('',*,*,#32225,.F.);
#46681=ORIENTED_EDGE('',*,*,#32226,.T.);
#46682=ORIENTED_EDGE('',*,*,#32222,.T.);
#46683=ORIENTED_EDGE('',*,*,#32227,.F.);
#46684=ORIENTED_EDGE('',*,*,#32228,.F.);
#46685=ORIENTED_EDGE('',*,*,#32229,.T.);
#46686=ORIENTED_EDGE('',*,*,#32225,.T.);
#46687=ORIENTED_EDGE('',*,*,#32230,.F.);
#46688=ORIENTED_EDGE('',*,*,#32231,.F.);
#46689=ORIENTED_EDGE('',*,*,#32232,.T.);
#46690=ORIENTED_EDGE('',*,*,#32228,.T.);
#46691=ORIENTED_EDGE('',*,*,#32233,.F.);
#46692=ORIENTED_EDGE('',*,*,#32234,.F.);
#46693=ORIENTED_EDGE('',*,*,#32235,.T.);
#46694=ORIENTED_EDGE('',*,*,#32231,.T.);
#46695=ORIENTED_EDGE('',*,*,#32236,.F.);
#46696=ORIENTED_EDGE('',*,*,#32237,.F.);
#46697=ORIENTED_EDGE('',*,*,#32238,.T.);
#46698=ORIENTED_EDGE('',*,*,#32234,.T.);
#46699=ORIENTED_EDGE('',*,*,#32239,.F.);
#46700=ORIENTED_EDGE('',*,*,#32240,.F.);
#46701=ORIENTED_EDGE('',*,*,#32241,.T.);
#46702=ORIENTED_EDGE('',*,*,#32237,.T.);
#46703=ORIENTED_EDGE('',*,*,#32242,.F.);
#46704=ORIENTED_EDGE('',*,*,#32243,.F.);
#46705=ORIENTED_EDGE('',*,*,#32244,.T.);
#46706=ORIENTED_EDGE('',*,*,#32240,.T.);
#46707=ORIENTED_EDGE('',*,*,#32245,.F.);
#46708=ORIENTED_EDGE('',*,*,#32246,.F.);
#46709=ORIENTED_EDGE('',*,*,#32247,.T.);
#46710=ORIENTED_EDGE('',*,*,#32243,.T.);
#46711=ORIENTED_EDGE('',*,*,#32248,.F.);
#46712=ORIENTED_EDGE('',*,*,#32249,.F.);
#46713=ORIENTED_EDGE('',*,*,#32250,.T.);
#46714=ORIENTED_EDGE('',*,*,#32246,.T.);
#46715=ORIENTED_EDGE('',*,*,#32251,.F.);
#46716=ORIENTED_EDGE('',*,*,#32252,.F.);
#46717=ORIENTED_EDGE('',*,*,#32253,.T.);
#46718=ORIENTED_EDGE('',*,*,#32249,.T.);
#46719=ORIENTED_EDGE('',*,*,#32254,.F.);
#46720=ORIENTED_EDGE('',*,*,#32211,.T.);
#46721=ORIENTED_EDGE('',*,*,#32255,.T.);
#46722=ORIENTED_EDGE('',*,*,#32256,.F.);
#46723=ORIENTED_EDGE('',*,*,#32257,.F.);
#46724=ORIENTED_EDGE('',*,*,#32258,.T.);
#46725=ORIENTED_EDGE('',*,*,#32258,.F.);
#46726=ORIENTED_EDGE('',*,*,#32259,.F.);
#46727=ORIENTED_EDGE('',*,*,#32208,.F.);
#46728=ORIENTED_EDGE('',*,*,#32204,.F.);
#46729=ORIENTED_EDGE('',*,*,#32201,.F.);
#46730=ORIENTED_EDGE('',*,*,#32198,.F.);
#46731=ORIENTED_EDGE('',*,*,#32195,.F.);
#46732=ORIENTED_EDGE('',*,*,#32192,.F.);
#46733=ORIENTED_EDGE('',*,*,#32189,.F.);
#46734=ORIENTED_EDGE('',*,*,#32186,.F.);
#46735=ORIENTED_EDGE('',*,*,#32183,.F.);
#46736=ORIENTED_EDGE('',*,*,#32180,.F.);
#46737=ORIENTED_EDGE('',*,*,#32177,.F.);
#46738=ORIENTED_EDGE('',*,*,#32174,.F.);
#46739=ORIENTED_EDGE('',*,*,#32171,.F.);
#46740=ORIENTED_EDGE('',*,*,#32168,.F.);
#46741=ORIENTED_EDGE('',*,*,#32165,.F.);
#46742=ORIENTED_EDGE('',*,*,#32162,.F.);
#46743=ORIENTED_EDGE('',*,*,#32260,.F.);
#46744=ORIENTED_EDGE('',*,*,#32261,.T.);
#46745=ORIENTED_EDGE('',*,*,#32254,.T.);
#46746=ORIENTED_EDGE('',*,*,#32251,.T.);
#46747=ORIENTED_EDGE('',*,*,#32248,.T.);
#46748=ORIENTED_EDGE('',*,*,#32245,.T.);
#46749=ORIENTED_EDGE('',*,*,#32242,.T.);
#46750=ORIENTED_EDGE('',*,*,#32239,.T.);
#46751=ORIENTED_EDGE('',*,*,#32236,.T.);
#46752=ORIENTED_EDGE('',*,*,#32233,.T.);
#46753=ORIENTED_EDGE('',*,*,#32230,.T.);
#46754=ORIENTED_EDGE('',*,*,#32227,.T.);
#46755=ORIENTED_EDGE('',*,*,#32224,.T.);
#46756=ORIENTED_EDGE('',*,*,#32221,.T.);
#46757=ORIENTED_EDGE('',*,*,#32218,.T.);
#46758=ORIENTED_EDGE('',*,*,#32215,.T.);
#46759=ORIENTED_EDGE('',*,*,#32212,.T.);
#46760=ORIENTED_EDGE('',*,*,#32262,.T.);
#46761=ORIENTED_EDGE('',*,*,#32263,.T.);
#46762=ORIENTED_EDGE('',*,*,#32264,.T.);
#46763=ORIENTED_EDGE('',*,*,#32265,.T.);
#46764=ORIENTED_EDGE('',*,*,#32260,.T.);
#46765=ORIENTED_EDGE('',*,*,#32252,.T.);
#46766=ORIENTED_EDGE('',*,*,#32261,.F.);
#46767=ORIENTED_EDGE('',*,*,#32265,.F.);
#46768=ORIENTED_EDGE('',*,*,#32266,.T.);
#46769=ORIENTED_EDGE('',*,*,#32255,.F.);
#46770=ORIENTED_EDGE('',*,*,#32210,.F.);
#46771=ORIENTED_EDGE('',*,*,#32214,.F.);
#46772=ORIENTED_EDGE('',*,*,#32217,.F.);
#46773=ORIENTED_EDGE('',*,*,#32220,.F.);
#46774=ORIENTED_EDGE('',*,*,#32223,.F.);
#46775=ORIENTED_EDGE('',*,*,#32226,.F.);
#46776=ORIENTED_EDGE('',*,*,#32229,.F.);
#46777=ORIENTED_EDGE('',*,*,#32232,.F.);
#46778=ORIENTED_EDGE('',*,*,#32235,.F.);
#46779=ORIENTED_EDGE('',*,*,#32238,.F.);
#46780=ORIENTED_EDGE('',*,*,#32241,.F.);
#46781=ORIENTED_EDGE('',*,*,#32244,.F.);
#46782=ORIENTED_EDGE('',*,*,#32247,.F.);
#46783=ORIENTED_EDGE('',*,*,#32250,.F.);
#46784=ORIENTED_EDGE('',*,*,#32253,.F.);
#46785=ORIENTED_EDGE('',*,*,#32266,.F.);
#46786=ORIENTED_EDGE('',*,*,#32264,.F.);
#46787=ORIENTED_EDGE('',*,*,#32160,.F.);
#46788=ORIENTED_EDGE('',*,*,#32164,.F.);
#46789=ORIENTED_EDGE('',*,*,#32167,.F.);
#46790=ORIENTED_EDGE('',*,*,#32170,.F.);
#46791=ORIENTED_EDGE('',*,*,#32173,.F.);
#46792=ORIENTED_EDGE('',*,*,#32176,.F.);
#46793=ORIENTED_EDGE('',*,*,#32179,.F.);
#46794=ORIENTED_EDGE('',*,*,#32182,.F.);
#46795=ORIENTED_EDGE('',*,*,#32185,.F.);
#46796=ORIENTED_EDGE('',*,*,#32188,.F.);
#46797=ORIENTED_EDGE('',*,*,#32191,.F.);
#46798=ORIENTED_EDGE('',*,*,#32194,.F.);
#46799=ORIENTED_EDGE('',*,*,#32197,.F.);
#46800=ORIENTED_EDGE('',*,*,#32200,.F.);
#46801=ORIENTED_EDGE('',*,*,#32203,.F.);
#46802=ORIENTED_EDGE('',*,*,#32207,.F.);
#46803=ORIENTED_EDGE('',*,*,#32206,.T.);
#46804=ORIENTED_EDGE('',*,*,#32267,.T.);
#46805=ORIENTED_EDGE('',*,*,#32257,.T.);
#46806=ORIENTED_EDGE('',*,*,#32268,.T.);
#46807=ORIENTED_EDGE('',*,*,#32269,.T.);
#46808=ORIENTED_EDGE('',*,*,#32268,.F.);
#46809=ORIENTED_EDGE('',*,*,#32256,.T.);
#46810=ORIENTED_EDGE('',*,*,#32205,.T.);
#46811=ORIENTED_EDGE('',*,*,#32259,.T.);
#46812=ORIENTED_EDGE('',*,*,#32267,.F.);
#46813=ORIENTED_EDGE('',*,*,#32270,.F.);
#46814=ORIENTED_EDGE('',*,*,#32269,.F.);
#46815=ORIENTED_EDGE('',*,*,#32271,.F.);
#46816=ORIENTED_EDGE('',*,*,#32272,.T.);
#46817=ORIENTED_EDGE('',*,*,#32273,.T.);
#46818=ORIENTED_EDGE('',*,*,#32274,.T.);
#46819=ORIENTED_EDGE('',*,*,#32275,.F.);
#46820=ORIENTED_EDGE('',*,*,#32274,.F.);
#46821=ORIENTED_EDGE('',*,*,#32276,.F.);
#46822=ORIENTED_EDGE('',*,*,#32277,.F.);
#46823=ORIENTED_EDGE('',*,*,#32276,.T.);
#46824=ORIENTED_EDGE('',*,*,#32273,.F.);
#46825=ORIENTED_EDGE('',*,*,#32278,.T.);
#46826=ORIENTED_EDGE('',*,*,#32279,.F.);
#46827=ORIENTED_EDGE('',*,*,#32278,.F.);
#46828=ORIENTED_EDGE('',*,*,#32272,.F.);
#46829=ORIENTED_EDGE('',*,*,#32280,.F.);
#46830=ORIENTED_EDGE('',*,*,#32281,.T.);
#46831=ORIENTED_EDGE('',*,*,#32282,.T.);
#46832=ORIENTED_EDGE('',*,*,#32283,.T.);
#46833=ORIENTED_EDGE('',*,*,#32284,.F.);
#46834=ORIENTED_EDGE('',*,*,#32283,.F.);
#46835=ORIENTED_EDGE('',*,*,#32285,.F.);
#46836=ORIENTED_EDGE('',*,*,#32286,.F.);
#46837=ORIENTED_EDGE('',*,*,#32285,.T.);
#46838=ORIENTED_EDGE('',*,*,#32282,.F.);
#46839=ORIENTED_EDGE('',*,*,#32287,.T.);
#46840=ORIENTED_EDGE('',*,*,#32288,.F.);
#46841=ORIENTED_EDGE('',*,*,#32287,.F.);
#46842=ORIENTED_EDGE('',*,*,#32281,.F.);
#46843=ORIENTED_EDGE('',*,*,#32289,.F.);
#46844=ORIENTED_EDGE('',*,*,#32290,.T.);
#46845=ORIENTED_EDGE('',*,*,#32291,.T.);
#46846=ORIENTED_EDGE('',*,*,#32292,.T.);
#46847=ORIENTED_EDGE('',*,*,#32293,.F.);
#46848=ORIENTED_EDGE('',*,*,#32292,.F.);
#46849=ORIENTED_EDGE('',*,*,#32294,.F.);
#46850=ORIENTED_EDGE('',*,*,#32295,.F.);
#46851=ORIENTED_EDGE('',*,*,#32294,.T.);
#46852=ORIENTED_EDGE('',*,*,#32291,.F.);
#46853=ORIENTED_EDGE('',*,*,#32296,.T.);
#46854=ORIENTED_EDGE('',*,*,#32297,.F.);
#46855=ORIENTED_EDGE('',*,*,#32296,.F.);
#46856=ORIENTED_EDGE('',*,*,#32290,.F.);
#46857=ORIENTED_EDGE('',*,*,#32298,.F.);
#46858=ORIENTED_EDGE('',*,*,#32299,.T.);
#46859=ORIENTED_EDGE('',*,*,#32300,.T.);
#46860=ORIENTED_EDGE('',*,*,#32301,.T.);
#46861=ORIENTED_EDGE('',*,*,#32302,.F.);
#46862=ORIENTED_EDGE('',*,*,#32301,.F.);
#46863=ORIENTED_EDGE('',*,*,#32303,.F.);
#46864=ORIENTED_EDGE('',*,*,#32304,.F.);
#46865=ORIENTED_EDGE('',*,*,#32303,.T.);
#46866=ORIENTED_EDGE('',*,*,#32300,.F.);
#46867=ORIENTED_EDGE('',*,*,#32305,.T.);
#46868=ORIENTED_EDGE('',*,*,#32306,.F.);
#46869=ORIENTED_EDGE('',*,*,#32305,.F.);
#46870=ORIENTED_EDGE('',*,*,#32299,.F.);
#46871=ORIENTED_EDGE('',*,*,#32307,.F.);
#46872=ORIENTED_EDGE('',*,*,#32308,.T.);
#46873=ORIENTED_EDGE('',*,*,#32309,.T.);
#46874=ORIENTED_EDGE('',*,*,#32310,.T.);
#46875=ORIENTED_EDGE('',*,*,#32311,.F.);
#46876=ORIENTED_EDGE('',*,*,#32310,.F.);
#46877=ORIENTED_EDGE('',*,*,#32312,.F.);
#46878=ORIENTED_EDGE('',*,*,#32313,.F.);
#46879=ORIENTED_EDGE('',*,*,#32312,.T.);
#46880=ORIENTED_EDGE('',*,*,#32309,.F.);
#46881=ORIENTED_EDGE('',*,*,#32314,.T.);
#46882=ORIENTED_EDGE('',*,*,#32315,.F.);
#46883=ORIENTED_EDGE('',*,*,#32314,.F.);
#46884=ORIENTED_EDGE('',*,*,#32308,.F.);
#46885=ORIENTED_EDGE('',*,*,#32316,.F.);
#46886=ORIENTED_EDGE('',*,*,#32317,.T.);
#46887=ORIENTED_EDGE('',*,*,#32318,.T.);
#46888=ORIENTED_EDGE('',*,*,#32319,.T.);
#46889=ORIENTED_EDGE('',*,*,#32320,.F.);
#46890=ORIENTED_EDGE('',*,*,#32319,.F.);
#46891=ORIENTED_EDGE('',*,*,#32321,.F.);
#46892=ORIENTED_EDGE('',*,*,#32322,.F.);
#46893=ORIENTED_EDGE('',*,*,#32321,.T.);
#46894=ORIENTED_EDGE('',*,*,#32318,.F.);
#46895=ORIENTED_EDGE('',*,*,#32323,.T.);
#46896=ORIENTED_EDGE('',*,*,#32324,.F.);
#46897=ORIENTED_EDGE('',*,*,#32323,.F.);
#46898=ORIENTED_EDGE('',*,*,#32317,.F.);
#46899=ORIENTED_EDGE('',*,*,#32325,.F.);
#46900=ORIENTED_EDGE('',*,*,#32326,.T.);
#46901=ORIENTED_EDGE('',*,*,#32327,.T.);
#46902=ORIENTED_EDGE('',*,*,#32328,.T.);
#46903=ORIENTED_EDGE('',*,*,#32329,.F.);
#46904=ORIENTED_EDGE('',*,*,#32328,.F.);
#46905=ORIENTED_EDGE('',*,*,#32330,.F.);
#46906=ORIENTED_EDGE('',*,*,#32331,.F.);
#46907=ORIENTED_EDGE('',*,*,#32330,.T.);
#46908=ORIENTED_EDGE('',*,*,#32327,.F.);
#46909=ORIENTED_EDGE('',*,*,#32332,.T.);
#46910=ORIENTED_EDGE('',*,*,#32333,.F.);
#46911=ORIENTED_EDGE('',*,*,#32332,.F.);
#46912=ORIENTED_EDGE('',*,*,#32326,.F.);
#46913=ORIENTED_EDGE('',*,*,#32334,.F.);
#46914=ORIENTED_EDGE('',*,*,#32335,.T.);
#46915=ORIENTED_EDGE('',*,*,#32336,.T.);
#46916=ORIENTED_EDGE('',*,*,#32337,.T.);
#46917=ORIENTED_EDGE('',*,*,#32338,.F.);
#46918=ORIENTED_EDGE('',*,*,#32337,.F.);
#46919=ORIENTED_EDGE('',*,*,#32339,.F.);
#46920=ORIENTED_EDGE('',*,*,#32340,.F.);
#46921=ORIENTED_EDGE('',*,*,#32339,.T.);
#46922=ORIENTED_EDGE('',*,*,#32336,.F.);
#46923=ORIENTED_EDGE('',*,*,#32341,.T.);
#46924=ORIENTED_EDGE('',*,*,#32342,.F.);
#46925=ORIENTED_EDGE('',*,*,#32341,.F.);
#46926=ORIENTED_EDGE('',*,*,#32335,.F.);
#46927=ORIENTED_EDGE('',*,*,#32343,.F.);
#46928=ORIENTED_EDGE('',*,*,#32344,.T.);
#46929=ORIENTED_EDGE('',*,*,#32345,.T.);
#46930=ORIENTED_EDGE('',*,*,#32346,.T.);
#46931=ORIENTED_EDGE('',*,*,#32347,.F.);
#46932=ORIENTED_EDGE('',*,*,#32346,.F.);
#46933=ORIENTED_EDGE('',*,*,#32348,.F.);
#46934=ORIENTED_EDGE('',*,*,#32349,.F.);
#46935=ORIENTED_EDGE('',*,*,#32348,.T.);
#46936=ORIENTED_EDGE('',*,*,#32345,.F.);
#46937=ORIENTED_EDGE('',*,*,#32350,.T.);
#46938=ORIENTED_EDGE('',*,*,#32351,.F.);
#46939=ORIENTED_EDGE('',*,*,#32350,.F.);
#46940=ORIENTED_EDGE('',*,*,#32344,.F.);
#46941=ORIENTED_EDGE('',*,*,#32352,.F.);
#46942=ORIENTED_EDGE('',*,*,#32353,.T.);
#46943=ORIENTED_EDGE('',*,*,#32354,.T.);
#46944=ORIENTED_EDGE('',*,*,#32355,.T.);
#46945=ORIENTED_EDGE('',*,*,#32356,.F.);
#46946=ORIENTED_EDGE('',*,*,#32355,.F.);
#46947=ORIENTED_EDGE('',*,*,#32357,.F.);
#46948=ORIENTED_EDGE('',*,*,#32358,.F.);
#46949=ORIENTED_EDGE('',*,*,#32357,.T.);
#46950=ORIENTED_EDGE('',*,*,#32354,.F.);
#46951=ORIENTED_EDGE('',*,*,#32359,.T.);
#46952=ORIENTED_EDGE('',*,*,#32360,.F.);
#46953=ORIENTED_EDGE('',*,*,#32359,.F.);
#46954=ORIENTED_EDGE('',*,*,#32353,.F.);
#46955=ORIENTED_EDGE('',*,*,#32361,.F.);
#46956=ORIENTED_EDGE('',*,*,#32362,.T.);
#46957=ORIENTED_EDGE('',*,*,#32363,.T.);
#46958=ORIENTED_EDGE('',*,*,#32364,.T.);
#46959=ORIENTED_EDGE('',*,*,#32365,.F.);
#46960=ORIENTED_EDGE('',*,*,#32364,.F.);
#46961=ORIENTED_EDGE('',*,*,#32366,.F.);
#46962=ORIENTED_EDGE('',*,*,#32367,.F.);
#46963=ORIENTED_EDGE('',*,*,#32366,.T.);
#46964=ORIENTED_EDGE('',*,*,#32363,.F.);
#46965=ORIENTED_EDGE('',*,*,#32368,.T.);
#46966=ORIENTED_EDGE('',*,*,#32369,.F.);
#46967=ORIENTED_EDGE('',*,*,#32368,.F.);
#46968=ORIENTED_EDGE('',*,*,#32362,.F.);
#46969=ORIENTED_EDGE('',*,*,#32370,.F.);
#46970=ORIENTED_EDGE('',*,*,#32371,.T.);
#46971=ORIENTED_EDGE('',*,*,#32372,.T.);
#46972=ORIENTED_EDGE('',*,*,#32373,.T.);
#46973=ORIENTED_EDGE('',*,*,#32374,.F.);
#46974=ORIENTED_EDGE('',*,*,#32373,.F.);
#46975=ORIENTED_EDGE('',*,*,#32375,.F.);
#46976=ORIENTED_EDGE('',*,*,#32376,.F.);
#46977=ORIENTED_EDGE('',*,*,#32375,.T.);
#46978=ORIENTED_EDGE('',*,*,#32372,.F.);
#46979=ORIENTED_EDGE('',*,*,#32377,.T.);
#46980=ORIENTED_EDGE('',*,*,#32378,.F.);
#46981=ORIENTED_EDGE('',*,*,#32377,.F.);
#46982=ORIENTED_EDGE('',*,*,#32371,.F.);
#46983=ORIENTED_EDGE('',*,*,#32379,.F.);
#46984=ORIENTED_EDGE('',*,*,#32380,.T.);
#46985=ORIENTED_EDGE('',*,*,#32381,.T.);
#46986=ORIENTED_EDGE('',*,*,#32382,.T.);
#46987=ORIENTED_EDGE('',*,*,#32383,.F.);
#46988=ORIENTED_EDGE('',*,*,#32382,.F.);
#46989=ORIENTED_EDGE('',*,*,#32384,.F.);
#46990=ORIENTED_EDGE('',*,*,#32385,.F.);
#46991=ORIENTED_EDGE('',*,*,#32384,.T.);
#46992=ORIENTED_EDGE('',*,*,#32381,.F.);
#46993=ORIENTED_EDGE('',*,*,#32386,.T.);
#46994=ORIENTED_EDGE('',*,*,#32387,.F.);
#46995=ORIENTED_EDGE('',*,*,#32386,.F.);
#46996=ORIENTED_EDGE('',*,*,#32380,.F.);
#46997=ORIENTED_EDGE('',*,*,#32388,.F.);
#46998=ORIENTED_EDGE('',*,*,#32389,.T.);
#46999=ORIENTED_EDGE('',*,*,#32390,.T.);
#47000=ORIENTED_EDGE('',*,*,#32391,.T.);
#47001=ORIENTED_EDGE('',*,*,#32392,.F.);
#47002=ORIENTED_EDGE('',*,*,#32391,.F.);
#47003=ORIENTED_EDGE('',*,*,#32393,.F.);
#47004=ORIENTED_EDGE('',*,*,#32394,.F.);
#47005=ORIENTED_EDGE('',*,*,#32393,.T.);
#47006=ORIENTED_EDGE('',*,*,#32390,.F.);
#47007=ORIENTED_EDGE('',*,*,#32395,.T.);
#47008=ORIENTED_EDGE('',*,*,#32396,.F.);
#47009=ORIENTED_EDGE('',*,*,#32395,.F.);
#47010=ORIENTED_EDGE('',*,*,#32389,.F.);
#47011=ORIENTED_EDGE('',*,*,#32397,.F.);
#47012=ORIENTED_EDGE('',*,*,#32398,.T.);
#47013=ORIENTED_EDGE('',*,*,#32399,.T.);
#47014=ORIENTED_EDGE('',*,*,#32400,.T.);
#47015=ORIENTED_EDGE('',*,*,#32401,.F.);
#47016=ORIENTED_EDGE('',*,*,#32400,.F.);
#47017=ORIENTED_EDGE('',*,*,#32402,.F.);
#47018=ORIENTED_EDGE('',*,*,#32403,.F.);
#47019=ORIENTED_EDGE('',*,*,#32402,.T.);
#47020=ORIENTED_EDGE('',*,*,#32399,.F.);
#47021=ORIENTED_EDGE('',*,*,#32404,.T.);
#47022=ORIENTED_EDGE('',*,*,#32405,.F.);
#47023=ORIENTED_EDGE('',*,*,#32404,.F.);
#47024=ORIENTED_EDGE('',*,*,#32398,.F.);
#47025=ORIENTED_EDGE('',*,*,#32406,.F.);
#47026=ORIENTED_EDGE('',*,*,#32407,.T.);
#47027=ORIENTED_EDGE('',*,*,#32408,.T.);
#47028=ORIENTED_EDGE('',*,*,#32409,.T.);
#47029=ORIENTED_EDGE('',*,*,#32410,.F.);
#47030=ORIENTED_EDGE('',*,*,#32409,.F.);
#47031=ORIENTED_EDGE('',*,*,#32411,.F.);
#47032=ORIENTED_EDGE('',*,*,#32412,.F.);
#47033=ORIENTED_EDGE('',*,*,#32411,.T.);
#47034=ORIENTED_EDGE('',*,*,#32408,.F.);
#47035=ORIENTED_EDGE('',*,*,#32413,.T.);
#47036=ORIENTED_EDGE('',*,*,#32414,.F.);
#47037=ORIENTED_EDGE('',*,*,#32413,.F.);
#47038=ORIENTED_EDGE('',*,*,#32407,.F.);
#47039=ORIENTED_EDGE('',*,*,#32415,.F.);
#47040=ORIENTED_EDGE('',*,*,#32416,.T.);
#47041=ORIENTED_EDGE('',*,*,#32417,.T.);
#47042=ORIENTED_EDGE('',*,*,#32418,.T.);
#47043=ORIENTED_EDGE('',*,*,#32419,.F.);
#47044=ORIENTED_EDGE('',*,*,#32418,.F.);
#47045=ORIENTED_EDGE('',*,*,#32420,.F.);
#47046=ORIENTED_EDGE('',*,*,#32421,.F.);
#47047=ORIENTED_EDGE('',*,*,#32420,.T.);
#47048=ORIENTED_EDGE('',*,*,#32417,.F.);
#47049=ORIENTED_EDGE('',*,*,#32422,.T.);
#47050=ORIENTED_EDGE('',*,*,#32423,.F.);
#47051=ORIENTED_EDGE('',*,*,#32422,.F.);
#47052=ORIENTED_EDGE('',*,*,#32416,.F.);
#47053=ORIENTED_EDGE('',*,*,#32424,.F.);
#47054=ORIENTED_EDGE('',*,*,#32425,.T.);
#47055=ORIENTED_EDGE('',*,*,#32426,.T.);
#47056=ORIENTED_EDGE('',*,*,#32427,.T.);
#47057=ORIENTED_EDGE('',*,*,#32428,.F.);
#47058=ORIENTED_EDGE('',*,*,#32427,.F.);
#47059=ORIENTED_EDGE('',*,*,#32429,.F.);
#47060=ORIENTED_EDGE('',*,*,#32430,.F.);
#47061=ORIENTED_EDGE('',*,*,#32431,.F.);
#47062=ORIENTED_EDGE('',*,*,#32429,.T.);
#47063=ORIENTED_EDGE('',*,*,#32426,.F.);
#47064=ORIENTED_EDGE('',*,*,#32432,.T.);
#47065=ORIENTED_EDGE('',*,*,#32433,.F.);
#47066=ORIENTED_EDGE('',*,*,#32432,.F.);
#47067=ORIENTED_EDGE('',*,*,#32425,.F.);
#47068=ORIENTED_EDGE('',*,*,#32434,.F.);
#47069=ORIENTED_EDGE('',*,*,#32435,.F.);
#47070=ORIENTED_EDGE('',*,*,#32436,.T.);
#47071=ORIENTED_EDGE('',*,*,#32437,.T.);
#47072=ORIENTED_EDGE('',*,*,#32438,.T.);
#47073=ORIENTED_EDGE('',*,*,#32439,.F.);
#47074=ORIENTED_EDGE('',*,*,#32438,.F.);
#47075=ORIENTED_EDGE('',*,*,#32440,.F.);
#47076=ORIENTED_EDGE('',*,*,#32441,.F.);
#47077=ORIENTED_EDGE('',*,*,#32440,.T.);
#47078=ORIENTED_EDGE('',*,*,#32437,.F.);
#47079=ORIENTED_EDGE('',*,*,#32442,.T.);
#47080=ORIENTED_EDGE('',*,*,#32443,.F.);
#47081=ORIENTED_EDGE('',*,*,#32442,.F.);
#47082=ORIENTED_EDGE('',*,*,#32436,.F.);
#47083=ORIENTED_EDGE('',*,*,#32444,.F.);
#47084=ORIENTED_EDGE('',*,*,#32445,.T.);
#47085=ORIENTED_EDGE('',*,*,#32446,.T.);
#47086=ORIENTED_EDGE('',*,*,#32447,.T.);
#47087=ORIENTED_EDGE('',*,*,#32448,.F.);
#47088=ORIENTED_EDGE('',*,*,#32447,.F.);
#47089=ORIENTED_EDGE('',*,*,#32449,.F.);
#47090=ORIENTED_EDGE('',*,*,#32450,.F.);
#47091=ORIENTED_EDGE('',*,*,#32449,.T.);
#47092=ORIENTED_EDGE('',*,*,#32446,.F.);
#47093=ORIENTED_EDGE('',*,*,#32451,.T.);
#47094=ORIENTED_EDGE('',*,*,#32452,.F.);
#47095=ORIENTED_EDGE('',*,*,#32451,.F.);
#47096=ORIENTED_EDGE('',*,*,#32445,.F.);
#47097=ORIENTED_EDGE('',*,*,#32453,.F.);
#47098=ORIENTED_EDGE('',*,*,#32454,.T.);
#47099=ORIENTED_EDGE('',*,*,#32455,.T.);
#47100=ORIENTED_EDGE('',*,*,#32456,.T.);
#47101=ORIENTED_EDGE('',*,*,#32457,.F.);
#47102=ORIENTED_EDGE('',*,*,#32456,.F.);
#47103=ORIENTED_EDGE('',*,*,#32458,.F.);
#47104=ORIENTED_EDGE('',*,*,#32459,.F.);
#47105=ORIENTED_EDGE('',*,*,#32458,.T.);
#47106=ORIENTED_EDGE('',*,*,#32455,.F.);
#47107=ORIENTED_EDGE('',*,*,#32460,.T.);
#47108=ORIENTED_EDGE('',*,*,#32461,.F.);
#47109=ORIENTED_EDGE('',*,*,#32460,.F.);
#47110=ORIENTED_EDGE('',*,*,#32454,.F.);
#47111=ORIENTED_EDGE('',*,*,#32462,.F.);
#47112=ORIENTED_EDGE('',*,*,#32463,.T.);
#47113=ORIENTED_EDGE('',*,*,#32464,.T.);
#47114=ORIENTED_EDGE('',*,*,#32465,.T.);
#47115=ORIENTED_EDGE('',*,*,#32466,.F.);
#47116=ORIENTED_EDGE('',*,*,#32465,.F.);
#47117=ORIENTED_EDGE('',*,*,#32467,.F.);
#47118=ORIENTED_EDGE('',*,*,#32468,.F.);
#47119=ORIENTED_EDGE('',*,*,#32467,.T.);
#47120=ORIENTED_EDGE('',*,*,#32464,.F.);
#47121=ORIENTED_EDGE('',*,*,#32469,.T.);
#47122=ORIENTED_EDGE('',*,*,#32470,.F.);
#47123=ORIENTED_EDGE('',*,*,#32469,.F.);
#47124=ORIENTED_EDGE('',*,*,#32463,.F.);
#47125=ORIENTED_EDGE('',*,*,#32471,.F.);
#47126=ORIENTED_EDGE('',*,*,#32472,.T.);
#47127=ORIENTED_EDGE('',*,*,#32473,.T.);
#47128=ORIENTED_EDGE('',*,*,#32474,.T.);
#47129=ORIENTED_EDGE('',*,*,#32475,.F.);
#47130=ORIENTED_EDGE('',*,*,#32474,.F.);
#47131=ORIENTED_EDGE('',*,*,#32476,.F.);
#47132=ORIENTED_EDGE('',*,*,#32477,.F.);
#47133=ORIENTED_EDGE('',*,*,#32476,.T.);
#47134=ORIENTED_EDGE('',*,*,#32473,.F.);
#47135=ORIENTED_EDGE('',*,*,#32478,.T.);
#47136=ORIENTED_EDGE('',*,*,#32479,.F.);
#47137=ORIENTED_EDGE('',*,*,#32478,.F.);
#47138=ORIENTED_EDGE('',*,*,#32472,.F.);
#47139=ORIENTED_EDGE('',*,*,#32480,.F.);
#47140=ORIENTED_EDGE('',*,*,#32481,.T.);
#47141=ORIENTED_EDGE('',*,*,#32482,.T.);
#47142=ORIENTED_EDGE('',*,*,#32483,.T.);
#47143=ORIENTED_EDGE('',*,*,#32484,.F.);
#47144=ORIENTED_EDGE('',*,*,#32483,.F.);
#47145=ORIENTED_EDGE('',*,*,#32485,.F.);
#47146=ORIENTED_EDGE('',*,*,#32486,.F.);
#47147=ORIENTED_EDGE('',*,*,#32485,.T.);
#47148=ORIENTED_EDGE('',*,*,#32482,.F.);
#47149=ORIENTED_EDGE('',*,*,#32487,.T.);
#47150=ORIENTED_EDGE('',*,*,#32488,.F.);
#47151=ORIENTED_EDGE('',*,*,#32487,.F.);
#47152=ORIENTED_EDGE('',*,*,#32481,.F.);
#47153=ORIENTED_EDGE('',*,*,#32489,.F.);
#47154=ORIENTED_EDGE('',*,*,#32490,.T.);
#47155=ORIENTED_EDGE('',*,*,#32491,.T.);
#47156=ORIENTED_EDGE('',*,*,#32492,.T.);
#47157=ORIENTED_EDGE('',*,*,#32493,.F.);
#47158=ORIENTED_EDGE('',*,*,#32492,.F.);
#47159=ORIENTED_EDGE('',*,*,#32494,.F.);
#47160=ORIENTED_EDGE('',*,*,#32495,.F.);
#47161=ORIENTED_EDGE('',*,*,#32494,.T.);
#47162=ORIENTED_EDGE('',*,*,#32491,.F.);
#47163=ORIENTED_EDGE('',*,*,#32496,.T.);
#47164=ORIENTED_EDGE('',*,*,#32497,.F.);
#47165=ORIENTED_EDGE('',*,*,#32496,.F.);
#47166=ORIENTED_EDGE('',*,*,#32490,.F.);
#47167=ORIENTED_EDGE('',*,*,#32498,.F.);
#47168=ORIENTED_EDGE('',*,*,#32499,.T.);
#47169=ORIENTED_EDGE('',*,*,#32500,.T.);
#47170=ORIENTED_EDGE('',*,*,#32501,.T.);
#47171=ORIENTED_EDGE('',*,*,#32502,.F.);
#47172=ORIENTED_EDGE('',*,*,#32501,.F.);
#47173=ORIENTED_EDGE('',*,*,#32503,.F.);
#47174=ORIENTED_EDGE('',*,*,#32504,.F.);
#47175=ORIENTED_EDGE('',*,*,#32503,.T.);
#47176=ORIENTED_EDGE('',*,*,#32500,.F.);
#47177=ORIENTED_EDGE('',*,*,#32505,.T.);
#47178=ORIENTED_EDGE('',*,*,#32506,.F.);
#47179=ORIENTED_EDGE('',*,*,#32505,.F.);
#47180=ORIENTED_EDGE('',*,*,#32499,.F.);
#47181=ORIENTED_EDGE('',*,*,#32507,.F.);
#47182=ORIENTED_EDGE('',*,*,#32508,.T.);
#47183=ORIENTED_EDGE('',*,*,#32509,.T.);
#47184=ORIENTED_EDGE('',*,*,#32510,.T.);
#47185=ORIENTED_EDGE('',*,*,#32511,.F.);
#47186=ORIENTED_EDGE('',*,*,#32510,.F.);
#47187=ORIENTED_EDGE('',*,*,#32512,.F.);
#47188=ORIENTED_EDGE('',*,*,#32513,.F.);
#47189=ORIENTED_EDGE('',*,*,#32512,.T.);
#47190=ORIENTED_EDGE('',*,*,#32509,.F.);
#47191=ORIENTED_EDGE('',*,*,#32514,.T.);
#47192=ORIENTED_EDGE('',*,*,#32515,.F.);
#47193=ORIENTED_EDGE('',*,*,#32514,.F.);
#47194=ORIENTED_EDGE('',*,*,#32508,.F.);
#47195=ORIENTED_EDGE('',*,*,#32516,.F.);
#47196=ORIENTED_EDGE('',*,*,#32517,.T.);
#47197=ORIENTED_EDGE('',*,*,#32518,.T.);
#47198=ORIENTED_EDGE('',*,*,#32519,.T.);
#47199=ORIENTED_EDGE('',*,*,#32520,.F.);
#47200=ORIENTED_EDGE('',*,*,#32519,.F.);
#47201=ORIENTED_EDGE('',*,*,#32521,.F.);
#47202=ORIENTED_EDGE('',*,*,#32522,.F.);
#47203=ORIENTED_EDGE('',*,*,#32521,.T.);
#47204=ORIENTED_EDGE('',*,*,#32518,.F.);
#47205=ORIENTED_EDGE('',*,*,#32523,.T.);
#47206=ORIENTED_EDGE('',*,*,#32524,.F.);
#47207=ORIENTED_EDGE('',*,*,#32523,.F.);
#47208=ORIENTED_EDGE('',*,*,#32517,.F.);
#47209=ORIENTED_EDGE('',*,*,#32525,.F.);
#47210=ORIENTED_EDGE('',*,*,#32526,.T.);
#47211=ORIENTED_EDGE('',*,*,#32527,.T.);
#47212=ORIENTED_EDGE('',*,*,#32528,.T.);
#47213=ORIENTED_EDGE('',*,*,#32529,.F.);
#47214=ORIENTED_EDGE('',*,*,#32528,.F.);
#47215=ORIENTED_EDGE('',*,*,#32530,.F.);
#47216=ORIENTED_EDGE('',*,*,#32531,.F.);
#47217=ORIENTED_EDGE('',*,*,#32530,.T.);
#47218=ORIENTED_EDGE('',*,*,#32527,.F.);
#47219=ORIENTED_EDGE('',*,*,#32532,.T.);
#47220=ORIENTED_EDGE('',*,*,#32533,.F.);
#47221=ORIENTED_EDGE('',*,*,#32532,.F.);
#47222=ORIENTED_EDGE('',*,*,#32526,.F.);
#47223=ORIENTED_EDGE('',*,*,#32534,.F.);
#47224=ORIENTED_EDGE('',*,*,#32535,.T.);
#47225=ORIENTED_EDGE('',*,*,#32536,.T.);
#47226=ORIENTED_EDGE('',*,*,#32537,.T.);
#47227=ORIENTED_EDGE('',*,*,#32538,.F.);
#47228=ORIENTED_EDGE('',*,*,#32537,.F.);
#47229=ORIENTED_EDGE('',*,*,#32539,.F.);
#47230=ORIENTED_EDGE('',*,*,#32540,.F.);
#47231=ORIENTED_EDGE('',*,*,#32539,.T.);
#47232=ORIENTED_EDGE('',*,*,#32536,.F.);
#47233=ORIENTED_EDGE('',*,*,#32541,.T.);
#47234=ORIENTED_EDGE('',*,*,#32542,.F.);
#47235=ORIENTED_EDGE('',*,*,#32541,.F.);
#47236=ORIENTED_EDGE('',*,*,#32535,.F.);
#47237=ORIENTED_EDGE('',*,*,#32543,.F.);
#47238=ORIENTED_EDGE('',*,*,#32544,.T.);
#47239=ORIENTED_EDGE('',*,*,#32545,.T.);
#47240=ORIENTED_EDGE('',*,*,#32546,.T.);
#47241=ORIENTED_EDGE('',*,*,#32547,.F.);
#47242=ORIENTED_EDGE('',*,*,#32546,.F.);
#47243=ORIENTED_EDGE('',*,*,#32548,.F.);
#47244=ORIENTED_EDGE('',*,*,#32549,.F.);
#47245=ORIENTED_EDGE('',*,*,#32548,.T.);
#47246=ORIENTED_EDGE('',*,*,#32545,.F.);
#47247=ORIENTED_EDGE('',*,*,#32550,.T.);
#47248=ORIENTED_EDGE('',*,*,#32551,.F.);
#47249=ORIENTED_EDGE('',*,*,#32550,.F.);
#47250=ORIENTED_EDGE('',*,*,#32544,.F.);
#47251=ORIENTED_EDGE('',*,*,#32552,.F.);
#47252=ORIENTED_EDGE('',*,*,#32553,.T.);
#47253=ORIENTED_EDGE('',*,*,#32554,.T.);
#47254=ORIENTED_EDGE('',*,*,#32555,.T.);
#47255=ORIENTED_EDGE('',*,*,#32556,.F.);
#47256=ORIENTED_EDGE('',*,*,#32555,.F.);
#47257=ORIENTED_EDGE('',*,*,#32557,.F.);
#47258=ORIENTED_EDGE('',*,*,#32558,.F.);
#47259=ORIENTED_EDGE('',*,*,#32557,.T.);
#47260=ORIENTED_EDGE('',*,*,#32554,.F.);
#47261=ORIENTED_EDGE('',*,*,#32559,.T.);
#47262=ORIENTED_EDGE('',*,*,#32560,.F.);
#47263=ORIENTED_EDGE('',*,*,#32559,.F.);
#47264=ORIENTED_EDGE('',*,*,#32553,.F.);
#47265=ORIENTED_EDGE('',*,*,#32561,.F.);
#47266=ORIENTED_EDGE('',*,*,#32562,.T.);
#47267=ORIENTED_EDGE('',*,*,#32563,.T.);
#47268=ORIENTED_EDGE('',*,*,#32564,.T.);
#47269=ORIENTED_EDGE('',*,*,#32565,.F.);
#47270=ORIENTED_EDGE('',*,*,#32564,.F.);
#47271=ORIENTED_EDGE('',*,*,#32566,.F.);
#47272=ORIENTED_EDGE('',*,*,#32567,.F.);
#47273=ORIENTED_EDGE('',*,*,#32566,.T.);
#47274=ORIENTED_EDGE('',*,*,#32563,.F.);
#47275=ORIENTED_EDGE('',*,*,#32568,.T.);
#47276=ORIENTED_EDGE('',*,*,#32569,.F.);
#47277=ORIENTED_EDGE('',*,*,#32568,.F.);
#47278=ORIENTED_EDGE('',*,*,#32562,.F.);
#47279=ORIENTED_EDGE('',*,*,#32570,.F.);
#47280=ORIENTED_EDGE('',*,*,#32571,.T.);
#47281=ORIENTED_EDGE('',*,*,#32572,.T.);
#47282=ORIENTED_EDGE('',*,*,#32573,.T.);
#47283=ORIENTED_EDGE('',*,*,#32574,.F.);
#47284=ORIENTED_EDGE('',*,*,#32573,.F.);
#47285=ORIENTED_EDGE('',*,*,#32575,.F.);
#47286=ORIENTED_EDGE('',*,*,#32576,.F.);
#47287=ORIENTED_EDGE('',*,*,#32575,.T.);
#47288=ORIENTED_EDGE('',*,*,#32572,.F.);
#47289=ORIENTED_EDGE('',*,*,#32577,.T.);
#47290=ORIENTED_EDGE('',*,*,#32578,.F.);
#47291=ORIENTED_EDGE('',*,*,#32577,.F.);
#47292=ORIENTED_EDGE('',*,*,#32571,.F.);
#47293=ORIENTED_EDGE('',*,*,#32579,.F.);
#47294=ORIENTED_EDGE('',*,*,#32580,.T.);
#47295=ORIENTED_EDGE('',*,*,#32581,.T.);
#47296=ORIENTED_EDGE('',*,*,#32582,.T.);
#47297=ORIENTED_EDGE('',*,*,#32583,.F.);
#47298=ORIENTED_EDGE('',*,*,#32582,.F.);
#47299=ORIENTED_EDGE('',*,*,#32584,.F.);
#47300=ORIENTED_EDGE('',*,*,#32585,.F.);
#47301=ORIENTED_EDGE('',*,*,#32584,.T.);
#47302=ORIENTED_EDGE('',*,*,#32581,.F.);
#47303=ORIENTED_EDGE('',*,*,#32586,.T.);
#47304=ORIENTED_EDGE('',*,*,#32587,.F.);
#47305=ORIENTED_EDGE('',*,*,#32586,.F.);
#47306=ORIENTED_EDGE('',*,*,#32580,.F.);
#47307=ORIENTED_EDGE('',*,*,#32588,.F.);
#47308=ORIENTED_EDGE('',*,*,#32589,.F.);
#47309=ORIENTED_EDGE('',*,*,#32590,.F.);
#47310=ORIENTED_EDGE('',*,*,#32591,.F.);
#47311=ORIENTED_EDGE('',*,*,#32592,.T.);
#47312=ORIENTED_EDGE('',*,*,#32593,.T.);
#47313=ORIENTED_EDGE('',*,*,#32589,.T.);
#47314=ORIENTED_EDGE('',*,*,#32594,.F.);
#47315=ORIENTED_EDGE('',*,*,#32590,.T.);
#47316=ORIENTED_EDGE('',*,*,#32593,.F.);
#47317=ORIENTED_EDGE('',*,*,#32595,.T.);
#47318=ORIENTED_EDGE('',*,*,#32596,.F.);
#47319=ORIENTED_EDGE('',*,*,#32595,.F.);
#47320=ORIENTED_EDGE('',*,*,#32592,.F.);
#47321=ORIENTED_EDGE('',*,*,#32597,.T.);
#47322=ORIENTED_EDGE('',*,*,#32598,.F.);
#47323=ORIENTED_EDGE('',*,*,#32597,.F.);
#47324=ORIENTED_EDGE('',*,*,#32599,.F.);
#47325=ORIENTED_EDGE('',*,*,#32600,.F.);
#47326=ORIENTED_EDGE('',*,*,#32601,.F.);
#47327=ORIENTED_EDGE('',*,*,#32602,.T.);
#47328=ORIENTED_EDGE('',*,*,#32603,.F.);
#47329=ORIENTED_EDGE('',*,*,#32602,.F.);
#47330=ORIENTED_EDGE('',*,*,#32604,.F.);
#47331=ORIENTED_EDGE('',*,*,#32605,.T.);
#47332=ORIENTED_EDGE('',*,*,#32606,.F.);
#47333=ORIENTED_EDGE('',*,*,#32605,.F.);
#47334=ORIENTED_EDGE('',*,*,#32607,.F.);
#47335=ORIENTED_EDGE('',*,*,#32608,.T.);
#47336=ORIENTED_EDGE('',*,*,#32609,.F.);
#47337=ORIENTED_EDGE('',*,*,#32608,.F.);
#47338=ORIENTED_EDGE('',*,*,#32610,.F.);
#47339=ORIENTED_EDGE('',*,*,#32611,.T.);
#47340=ORIENTED_EDGE('',*,*,#32612,.F.);
#47341=ORIENTED_EDGE('',*,*,#32611,.F.);
#47342=ORIENTED_EDGE('',*,*,#32613,.F.);
#47343=ORIENTED_EDGE('',*,*,#32614,.T.);
#47344=ORIENTED_EDGE('',*,*,#32615,.F.);
#47345=ORIENTED_EDGE('',*,*,#32614,.F.);
#47346=ORIENTED_EDGE('',*,*,#32616,.F.);
#47347=ORIENTED_EDGE('',*,*,#32600,.T.);
#47348=ORIENTED_EDGE('',*,*,#32607,.T.);
#47349=ORIENTED_EDGE('',*,*,#32604,.T.);
#47350=ORIENTED_EDGE('',*,*,#32601,.T.);
#47351=ORIENTED_EDGE('',*,*,#32616,.T.);
#47352=ORIENTED_EDGE('',*,*,#32613,.T.);
#47353=ORIENTED_EDGE('',*,*,#32610,.T.);
#47354=ORIENTED_EDGE('',*,*,#32598,.T.);
#47355=ORIENTED_EDGE('',*,*,#32617,.F.);
#47356=ORIENTED_EDGE('',*,*,#32262,.F.);
#47357=ORIENTED_EDGE('',*,*,#32161,.F.);
#47358=ORIENTED_EDGE('',*,*,#32263,.F.);
#47359=ORIENTED_EDGE('',*,*,#32618,.T.);
#47360=ORIENTED_EDGE('',*,*,#32617,.T.);
#47361=ORIENTED_EDGE('',*,*,#32618,.F.);
#47362=ORIENTED_EDGE('',*,*,#32271,.T.);
#47363=ORIENTED_EDGE('',*,*,#32619,.F.);
#47364=ORIENTED_EDGE('',*,*,#32286,.T.);
#47365=ORIENTED_EDGE('',*,*,#32288,.T.);
#47366=ORIENTED_EDGE('',*,*,#32280,.T.);
#47367=ORIENTED_EDGE('',*,*,#32620,.F.);
#47368=ORIENTED_EDGE('',*,*,#32295,.T.);
#47369=ORIENTED_EDGE('',*,*,#32297,.T.);
#47370=ORIENTED_EDGE('',*,*,#32289,.T.);
#47371=ORIENTED_EDGE('',*,*,#32621,.F.);
#47372=ORIENTED_EDGE('',*,*,#32304,.T.);
#47373=ORIENTED_EDGE('',*,*,#32306,.T.);
#47374=ORIENTED_EDGE('',*,*,#32298,.T.);
#47375=ORIENTED_EDGE('',*,*,#32622,.F.);
#47376=ORIENTED_EDGE('',*,*,#32313,.T.);
#47377=ORIENTED_EDGE('',*,*,#32315,.T.);
#47378=ORIENTED_EDGE('',*,*,#32307,.T.);
#47379=ORIENTED_EDGE('',*,*,#32623,.F.);
#47380=ORIENTED_EDGE('',*,*,#32322,.T.);
#47381=ORIENTED_EDGE('',*,*,#32324,.T.);
#47382=ORIENTED_EDGE('',*,*,#32316,.T.);
#47383=ORIENTED_EDGE('',*,*,#32624,.F.);
#47384=ORIENTED_EDGE('',*,*,#32331,.T.);
#47385=ORIENTED_EDGE('',*,*,#32333,.T.);
#47386=ORIENTED_EDGE('',*,*,#32325,.T.);
#47387=ORIENTED_EDGE('',*,*,#32625,.F.);
#47388=ORIENTED_EDGE('',*,*,#32340,.T.);
#47389=ORIENTED_EDGE('',*,*,#32342,.T.);
#47390=ORIENTED_EDGE('',*,*,#32334,.T.);
#47391=ORIENTED_EDGE('',*,*,#32626,.F.);
#47392=ORIENTED_EDGE('',*,*,#32349,.T.);
#47393=ORIENTED_EDGE('',*,*,#32351,.T.);
#47394=ORIENTED_EDGE('',*,*,#32343,.T.);
#47395=ORIENTED_EDGE('',*,*,#32627,.F.);
#47396=ORIENTED_EDGE('',*,*,#32358,.T.);
#47397=ORIENTED_EDGE('',*,*,#32360,.T.);
#47398=ORIENTED_EDGE('',*,*,#32352,.T.);
#47399=ORIENTED_EDGE('',*,*,#32628,.F.);
#47400=ORIENTED_EDGE('',*,*,#32367,.T.);
#47401=ORIENTED_EDGE('',*,*,#32369,.T.);
#47402=ORIENTED_EDGE('',*,*,#32361,.T.);
#47403=ORIENTED_EDGE('',*,*,#32629,.F.);
#47404=ORIENTED_EDGE('',*,*,#32376,.T.);
#47405=ORIENTED_EDGE('',*,*,#32378,.T.);
#47406=ORIENTED_EDGE('',*,*,#32370,.T.);
#47407=ORIENTED_EDGE('',*,*,#32630,.F.);
#47408=ORIENTED_EDGE('',*,*,#32385,.T.);
#47409=ORIENTED_EDGE('',*,*,#32387,.T.);
#47410=ORIENTED_EDGE('',*,*,#32379,.T.);
#47411=ORIENTED_EDGE('',*,*,#32631,.F.);
#47412=ORIENTED_EDGE('',*,*,#32394,.T.);
#47413=ORIENTED_EDGE('',*,*,#32396,.T.);
#47414=ORIENTED_EDGE('',*,*,#32388,.T.);
#47415=ORIENTED_EDGE('',*,*,#32632,.F.);
#47416=ORIENTED_EDGE('',*,*,#32403,.T.);
#47417=ORIENTED_EDGE('',*,*,#32405,.T.);
#47418=ORIENTED_EDGE('',*,*,#32397,.T.);
#47419=ORIENTED_EDGE('',*,*,#32633,.F.);
#47420=ORIENTED_EDGE('',*,*,#32412,.T.);
#47421=ORIENTED_EDGE('',*,*,#32414,.T.);
#47422=ORIENTED_EDGE('',*,*,#32406,.T.);
#47423=ORIENTED_EDGE('',*,*,#32634,.F.);
#47424=ORIENTED_EDGE('',*,*,#32421,.T.);
#47425=ORIENTED_EDGE('',*,*,#32423,.T.);
#47426=ORIENTED_EDGE('',*,*,#32415,.T.);
#47427=ORIENTED_EDGE('',*,*,#32635,.F.);
#47428=ORIENTED_EDGE('',*,*,#32431,.T.);
#47429=ORIENTED_EDGE('',*,*,#32433,.T.);
#47430=ORIENTED_EDGE('',*,*,#32636,.T.);
#47431=ORIENTED_EDGE('',*,*,#32270,.T.);
#47432=ORIENTED_EDGE('',*,*,#32636,.F.);
#47433=ORIENTED_EDGE('',*,*,#32434,.T.);
#47434=ORIENTED_EDGE('',*,*,#32424,.T.);
#47435=ORIENTED_EDGE('',*,*,#32637,.F.);
#47436=ORIENTED_EDGE('',*,*,#32441,.T.);
#47437=ORIENTED_EDGE('',*,*,#32443,.T.);
#47438=ORIENTED_EDGE('',*,*,#32435,.T.);
#47439=ORIENTED_EDGE('',*,*,#32638,.F.);
#47440=ORIENTED_EDGE('',*,*,#32450,.T.);
#47441=ORIENTED_EDGE('',*,*,#32452,.T.);
#47442=ORIENTED_EDGE('',*,*,#32444,.T.);
#47443=ORIENTED_EDGE('',*,*,#32639,.F.);
#47444=ORIENTED_EDGE('',*,*,#32459,.T.);
#47445=ORIENTED_EDGE('',*,*,#32461,.T.);
#47446=ORIENTED_EDGE('',*,*,#32453,.T.);
#47447=ORIENTED_EDGE('',*,*,#32640,.F.);
#47448=ORIENTED_EDGE('',*,*,#32468,.T.);
#47449=ORIENTED_EDGE('',*,*,#32470,.T.);
#47450=ORIENTED_EDGE('',*,*,#32462,.T.);
#47451=ORIENTED_EDGE('',*,*,#32641,.F.);
#47452=ORIENTED_EDGE('',*,*,#32477,.T.);
#47453=ORIENTED_EDGE('',*,*,#32479,.T.);
#47454=ORIENTED_EDGE('',*,*,#32471,.T.);
#47455=ORIENTED_EDGE('',*,*,#32642,.F.);
#47456=ORIENTED_EDGE('',*,*,#32486,.T.);
#47457=ORIENTED_EDGE('',*,*,#32488,.T.);
#47458=ORIENTED_EDGE('',*,*,#32480,.T.);
#47459=ORIENTED_EDGE('',*,*,#32643,.F.);
#47460=ORIENTED_EDGE('',*,*,#32495,.T.);
#47461=ORIENTED_EDGE('',*,*,#32497,.T.);
#47462=ORIENTED_EDGE('',*,*,#32489,.T.);
#47463=ORIENTED_EDGE('',*,*,#32644,.F.);
#47464=ORIENTED_EDGE('',*,*,#32504,.T.);
#47465=ORIENTED_EDGE('',*,*,#32506,.T.);
#47466=ORIENTED_EDGE('',*,*,#32498,.T.);
#47467=ORIENTED_EDGE('',*,*,#32645,.F.);
#47468=ORIENTED_EDGE('',*,*,#32513,.T.);
#47469=ORIENTED_EDGE('',*,*,#32515,.T.);
#47470=ORIENTED_EDGE('',*,*,#32507,.T.);
#47471=ORIENTED_EDGE('',*,*,#32646,.F.);
#47472=ORIENTED_EDGE('',*,*,#32522,.T.);
#47473=ORIENTED_EDGE('',*,*,#32524,.T.);
#47474=ORIENTED_EDGE('',*,*,#32516,.T.);
#47475=ORIENTED_EDGE('',*,*,#32647,.F.);
#47476=ORIENTED_EDGE('',*,*,#32531,.T.);
#47477=ORIENTED_EDGE('',*,*,#32533,.T.);
#47478=ORIENTED_EDGE('',*,*,#32525,.T.);
#47479=ORIENTED_EDGE('',*,*,#32648,.F.);
#47480=ORIENTED_EDGE('',*,*,#32540,.T.);
#47481=ORIENTED_EDGE('',*,*,#32542,.T.);
#47482=ORIENTED_EDGE('',*,*,#32534,.T.);
#47483=ORIENTED_EDGE('',*,*,#32649,.F.);
#47484=ORIENTED_EDGE('',*,*,#32549,.T.);
#47485=ORIENTED_EDGE('',*,*,#32551,.T.);
#47486=ORIENTED_EDGE('',*,*,#32543,.T.);
#47487=ORIENTED_EDGE('',*,*,#32650,.F.);
#47488=ORIENTED_EDGE('',*,*,#32558,.T.);
#47489=ORIENTED_EDGE('',*,*,#32560,.T.);
#47490=ORIENTED_EDGE('',*,*,#32552,.T.);
#47491=ORIENTED_EDGE('',*,*,#32651,.F.);
#47492=ORIENTED_EDGE('',*,*,#32567,.T.);
#47493=ORIENTED_EDGE('',*,*,#32569,.T.);
#47494=ORIENTED_EDGE('',*,*,#32561,.T.);
#47495=ORIENTED_EDGE('',*,*,#32652,.F.);
#47496=ORIENTED_EDGE('',*,*,#32576,.T.);
#47497=ORIENTED_EDGE('',*,*,#32578,.T.);
#47498=ORIENTED_EDGE('',*,*,#32570,.T.);
#47499=ORIENTED_EDGE('',*,*,#32653,.F.);
#47500=ORIENTED_EDGE('',*,*,#32585,.T.);
#47501=ORIENTED_EDGE('',*,*,#32587,.T.);
#47502=ORIENTED_EDGE('',*,*,#32579,.T.);
#47503=ORIENTED_EDGE('',*,*,#32654,.F.);
#47504=ORIENTED_EDGE('',*,*,#32594,.T.);
#47505=ORIENTED_EDGE('',*,*,#32596,.T.);
#47506=ORIENTED_EDGE('',*,*,#32591,.T.);
#47507=ORIENTED_EDGE('',*,*,#32655,.F.);
#47508=ORIENTED_EDGE('',*,*,#32277,.T.);
#47509=ORIENTED_EDGE('',*,*,#32279,.T.);
#47510=ORIENTED_EDGE('',*,*,#32656,.F.);
#47511=ORIENTED_EDGE('',*,*,#32657,.T.);
#47512=ORIENTED_EDGE('',*,*,#32430,.T.);
#47513=ORIENTED_EDGE('',*,*,#32635,.T.);
#47514=ORIENTED_EDGE('',*,*,#32419,.T.);
#47515=ORIENTED_EDGE('',*,*,#32634,.T.);
#47516=ORIENTED_EDGE('',*,*,#32410,.T.);
#47517=ORIENTED_EDGE('',*,*,#32633,.T.);
#47518=ORIENTED_EDGE('',*,*,#32401,.T.);
#47519=ORIENTED_EDGE('',*,*,#32632,.T.);
#47520=ORIENTED_EDGE('',*,*,#32392,.T.);
#47521=ORIENTED_EDGE('',*,*,#32631,.T.);
#47522=ORIENTED_EDGE('',*,*,#32383,.T.);
#47523=ORIENTED_EDGE('',*,*,#32630,.T.);
#47524=ORIENTED_EDGE('',*,*,#32374,.T.);
#47525=ORIENTED_EDGE('',*,*,#32629,.T.);
#47526=ORIENTED_EDGE('',*,*,#32365,.T.);
#47527=ORIENTED_EDGE('',*,*,#32628,.T.);
#47528=ORIENTED_EDGE('',*,*,#32356,.T.);
#47529=ORIENTED_EDGE('',*,*,#32627,.T.);
#47530=ORIENTED_EDGE('',*,*,#32347,.T.);
#47531=ORIENTED_EDGE('',*,*,#32626,.T.);
#47532=ORIENTED_EDGE('',*,*,#32338,.T.);
#47533=ORIENTED_EDGE('',*,*,#32625,.T.);
#47534=ORIENTED_EDGE('',*,*,#32329,.T.);
#47535=ORIENTED_EDGE('',*,*,#32624,.T.);
#47536=ORIENTED_EDGE('',*,*,#32320,.T.);
#47537=ORIENTED_EDGE('',*,*,#32623,.T.);
#47538=ORIENTED_EDGE('',*,*,#32311,.T.);
#47539=ORIENTED_EDGE('',*,*,#32622,.T.);
#47540=ORIENTED_EDGE('',*,*,#32302,.T.);
#47541=ORIENTED_EDGE('',*,*,#32621,.T.);
#47542=ORIENTED_EDGE('',*,*,#32293,.T.);
#47543=ORIENTED_EDGE('',*,*,#32620,.T.);
#47544=ORIENTED_EDGE('',*,*,#32284,.T.);
#47545=ORIENTED_EDGE('',*,*,#32619,.T.);
#47546=ORIENTED_EDGE('',*,*,#32275,.T.);
#47547=ORIENTED_EDGE('',*,*,#32655,.T.);
#47548=ORIENTED_EDGE('',*,*,#32588,.T.);
#47549=ORIENTED_EDGE('',*,*,#32654,.T.);
#47550=ORIENTED_EDGE('',*,*,#32583,.T.);
#47551=ORIENTED_EDGE('',*,*,#32653,.T.);
#47552=ORIENTED_EDGE('',*,*,#32574,.T.);
#47553=ORIENTED_EDGE('',*,*,#32652,.T.);
#47554=ORIENTED_EDGE('',*,*,#32565,.T.);
#47555=ORIENTED_EDGE('',*,*,#32651,.T.);
#47556=ORIENTED_EDGE('',*,*,#32556,.T.);
#47557=ORIENTED_EDGE('',*,*,#32650,.T.);
#47558=ORIENTED_EDGE('',*,*,#32547,.T.);
#47559=ORIENTED_EDGE('',*,*,#32649,.T.);
#47560=ORIENTED_EDGE('',*,*,#32538,.T.);
#47561=ORIENTED_EDGE('',*,*,#32648,.T.);
#47562=ORIENTED_EDGE('',*,*,#32529,.T.);
#47563=ORIENTED_EDGE('',*,*,#32647,.T.);
#47564=ORIENTED_EDGE('',*,*,#32520,.T.);
#47565=ORIENTED_EDGE('',*,*,#32646,.T.);
#47566=ORIENTED_EDGE('',*,*,#32511,.T.);
#47567=ORIENTED_EDGE('',*,*,#32645,.T.);
#47568=ORIENTED_EDGE('',*,*,#32502,.T.);
#47569=ORIENTED_EDGE('',*,*,#32644,.T.);
#47570=ORIENTED_EDGE('',*,*,#32493,.T.);
#47571=ORIENTED_EDGE('',*,*,#32643,.T.);
#47572=ORIENTED_EDGE('',*,*,#32484,.T.);
#47573=ORIENTED_EDGE('',*,*,#32642,.T.);
#47574=ORIENTED_EDGE('',*,*,#32475,.T.);
#47575=ORIENTED_EDGE('',*,*,#32641,.T.);
#47576=ORIENTED_EDGE('',*,*,#32466,.T.);
#47577=ORIENTED_EDGE('',*,*,#32640,.T.);
#47578=ORIENTED_EDGE('',*,*,#32457,.T.);
#47579=ORIENTED_EDGE('',*,*,#32639,.T.);
#47580=ORIENTED_EDGE('',*,*,#32448,.T.);
#47581=ORIENTED_EDGE('',*,*,#32638,.T.);
#47582=ORIENTED_EDGE('',*,*,#32439,.T.);
#47583=ORIENTED_EDGE('',*,*,#32637,.T.);
#47584=ORIENTED_EDGE('',*,*,#32428,.T.);
#47585=ORIENTED_EDGE('',*,*,#32657,.F.);
#47586=ORIENTED_EDGE('',*,*,#32656,.T.);
#47587=ORIENTED_EDGE('',*,*,#32609,.T.);
#47588=ORIENTED_EDGE('',*,*,#32612,.T.);
#47589=ORIENTED_EDGE('',*,*,#32615,.T.);
#47590=ORIENTED_EDGE('',*,*,#32599,.T.);
#47591=ORIENTED_EDGE('',*,*,#32603,.T.);
#47592=ORIENTED_EDGE('',*,*,#32606,.T.);
#48317=CONICAL_SURFACE('',#55126,1.25,1.02681050468488);
#48318=CONICAL_SURFACE('',#55137,2.7,0.785398163397448);
#48319=CONICAL_SURFACE('',#55175,4.7,0.785398163397448);
#50718=ADVANCED_FACE('',(#15631),#1198,.T.);
#50719=ADVANCED_FACE('',(#15632),#1199,.T.);
#50720=ADVANCED_FACE('',(#15633),#1200,.T.);
#50721=ADVANCED_FACE('',(#15634),#1201,.T.);
#50722=ADVANCED_FACE('',(#15635),#1202,.T.);
#50723=ADVANCED_FACE('',(#15636),#1203,.T.);
#50724=ADVANCED_FACE('',(#15637),#1204,.T.);
#50725=ADVANCED_FACE('',(#15638),#1205,.T.);
#50726=ADVANCED_FACE('',(#15639),#1206,.T.);
#50727=ADVANCED_FACE('',(#15640),#1207,.T.);
#50728=ADVANCED_FACE('',(#15641),#1208,.T.);
#50729=ADVANCED_FACE('',(#15642),#1209,.T.);
#50730=ADVANCED_FACE('',(#15643),#1210,.T.);
#50731=ADVANCED_FACE('',(#15644),#1211,.T.);
#50732=ADVANCED_FACE('',(#15645),#1212,.T.);
#50733=ADVANCED_FACE('',(#15646),#1213,.T.);
#50734=ADVANCED_FACE('',(#15647),#1214,.T.);
#50735=ADVANCED_FACE('',(#15648),#1215,.T.);
#50736=ADVANCED_FACE('',(#15649),#1216,.T.);
#50737=ADVANCED_FACE('',(#15650),#1217,.T.);
#50738=ADVANCED_FACE('',(#15651),#1218,.T.);
#50739=ADVANCED_FACE('',(#15652),#1219,.T.);
#50740=ADVANCED_FACE('',(#15653),#1220,.T.);
#50741=ADVANCED_FACE('',(#15654),#1221,.T.);
#50742=ADVANCED_FACE('',(#15655),#1222,.T.);
#50743=ADVANCED_FACE('',(#15656),#1223,.T.);
#50744=ADVANCED_FACE('',(#15657),#1224,.T.);
#50745=ADVANCED_FACE('',(#15658),#1225,.T.);
#50746=ADVANCED_FACE('',(#15659),#1226,.T.);
#50747=ADVANCED_FACE('',(#15660),#1227,.T.);
#50748=ADVANCED_FACE('',(#15661),#1228,.T.);
#50749=ADVANCED_FACE('',(#15662),#13065,.F.);
#50750=ADVANCED_FACE('',(#15663),#887,.F.);
#50751=ADVANCED_FACE('',(#15664),#13066,.T.);
#50752=ADVANCED_FACE('',(#15665),#1229,.T.);
#50753=ADVANCED_FACE('',(#15666),#888,.F.);
#50754=ADVANCED_FACE('',(#15667),#956,.F.);
#50755=ADVANCED_FACE('',(#15668),#1230,.T.);
#50756=ADVANCED_FACE('',(#15669,#1035),#13067,.T.);
#50757=ADVANCED_FACE('',(#15670),#13068,.F.);
#50758=ADVANCED_FACE('',(#15671),#13069,.F.);
#50759=ADVANCED_FACE('',(#15672),#13070,.F.);
#50760=ADVANCED_FACE('',(#15673),#13071,.T.);
#50761=ADVANCED_FACE('',(#15674),#13072,.F.);
#50762=ADVANCED_FACE('',(#15675),#13073,.F.);
#50763=ADVANCED_FACE('',(#15676),#13074,.F.);
#50764=ADVANCED_FACE('',(#15677),#13075,.T.);
#50765=ADVANCED_FACE('',(#15678),#13076,.F.);
#50766=ADVANCED_FACE('',(#15679),#13077,.F.);
#50767=ADVANCED_FACE('',(#15680),#13078,.F.);
#50768=ADVANCED_FACE('',(#15681),#13079,.T.);
#50769=ADVANCED_FACE('',(#15682),#13080,.F.);
#50770=ADVANCED_FACE('',(#15683),#13081,.F.);
#50771=ADVANCED_FACE('',(#15684),#13082,.F.);
#50772=ADVANCED_FACE('',(#15685),#13083,.T.);
#50773=ADVANCED_FACE('',(#15686),#13084,.F.);
#50774=ADVANCED_FACE('',(#15687),#13085,.F.);
#50775=ADVANCED_FACE('',(#15688),#13086,.F.);
#50776=ADVANCED_FACE('',(#15689),#13087,.T.);
#50777=ADVANCED_FACE('',(#15690),#13088,.F.);
#50778=ADVANCED_FACE('',(#15691),#13089,.F.);
#50779=ADVANCED_FACE('',(#15692),#13090,.F.);
#50780=ADVANCED_FACE('',(#15693),#13091,.T.);
#50781=ADVANCED_FACE('',(#15694),#13092,.F.);
#50782=ADVANCED_FACE('',(#15695),#13093,.F.);
#50783=ADVANCED_FACE('',(#15696),#13094,.F.);
#50784=ADVANCED_FACE('',(#15697),#13095,.T.);
#50785=ADVANCED_FACE('',(#15698),#13096,.F.);
#50786=ADVANCED_FACE('',(#15699),#13097,.F.);
#50787=ADVANCED_FACE('',(#15700),#13098,.F.);
#50788=ADVANCED_FACE('',(#15701),#13099,.T.);
#50789=ADVANCED_FACE('',(#15702),#13100,.F.);
#50790=ADVANCED_FACE('',(#15703),#13101,.F.);
#50791=ADVANCED_FACE('',(#15704),#13102,.F.);
#50792=ADVANCED_FACE('',(#15705),#13103,.T.);
#50793=ADVANCED_FACE('',(#15706),#13104,.F.);
#50794=ADVANCED_FACE('',(#15707),#13105,.F.);
#50795=ADVANCED_FACE('',(#15708),#13106,.F.);
#50796=ADVANCED_FACE('',(#15709),#13107,.T.);
#50797=ADVANCED_FACE('',(#15710),#13108,.F.);
#50798=ADVANCED_FACE('',(#15711),#13109,.F.);
#50799=ADVANCED_FACE('',(#15712),#13110,.F.);
#50800=ADVANCED_FACE('',(#15713),#13111,.T.);
#50801=ADVANCED_FACE('',(#15714),#13112,.F.);
#50802=ADVANCED_FACE('',(#15715),#13113,.F.);
#50803=ADVANCED_FACE('',(#15716),#13114,.F.);
#50804=ADVANCED_FACE('',(#15717),#13115,.T.);
#50805=ADVANCED_FACE('',(#15718),#13116,.F.);
#50806=ADVANCED_FACE('',(#15719),#13117,.F.);
#50807=ADVANCED_FACE('',(#15720),#13118,.F.);
#50808=ADVANCED_FACE('',(#15721),#13119,.T.);
#50809=ADVANCED_FACE('',(#15722),#13120,.F.);
#50810=ADVANCED_FACE('',(#15723),#13121,.F.);
#50811=ADVANCED_FACE('',(#15724),#13122,.F.);
#50812=ADVANCED_FACE('',(#15725),#13123,.T.);
#50813=ADVANCED_FACE('',(#15726),#13124,.F.);
#50814=ADVANCED_FACE('',(#15727),#13125,.F.);
#50815=ADVANCED_FACE('',(#15728),#13126,.F.);
#50816=ADVANCED_FACE('',(#15729),#13127,.T.);
#50817=ADVANCED_FACE('',(#15730),#13128,.F.);
#50818=ADVANCED_FACE('',(#15731),#13129,.F.);
#50819=ADVANCED_FACE('',(#15732),#13130,.F.);
#50820=ADVANCED_FACE('',(#15733),#13131,.T.);
#50821=ADVANCED_FACE('',(#15734),#13132,.F.);
#50822=ADVANCED_FACE('',(#15735),#13133,.F.);
#50823=ADVANCED_FACE('',(#15736),#13134,.F.);
#50824=ADVANCED_FACE('',(#15737),#13135,.T.);
#50825=ADVANCED_FACE('',(#15738),#13136,.F.);
#50826=ADVANCED_FACE('',(#15739),#13137,.F.);
#50827=ADVANCED_FACE('',(#15740),#13138,.F.);
#50828=ADVANCED_FACE('',(#15741),#13139,.T.);
#50829=ADVANCED_FACE('',(#15742),#13140,.F.);
#50830=ADVANCED_FACE('',(#15743),#13141,.F.);
#50831=ADVANCED_FACE('',(#15744),#13142,.F.);
#50832=ADVANCED_FACE('',(#15745),#13143,.T.);
#50833=ADVANCED_FACE('',(#15746),#13144,.F.);
#50834=ADVANCED_FACE('',(#15747),#13145,.F.);
#50835=ADVANCED_FACE('',(#15748),#13146,.F.);
#50836=ADVANCED_FACE('',(#15749),#13147,.T.);
#50837=ADVANCED_FACE('',(#15750),#13148,.F.);
#50838=ADVANCED_FACE('',(#15751),#13149,.F.);
#50839=ADVANCED_FACE('',(#15752),#13150,.F.);
#50840=ADVANCED_FACE('',(#15753),#13151,.T.);
#50841=ADVANCED_FACE('',(#15754),#13152,.F.);
#50842=ADVANCED_FACE('',(#15755),#13153,.F.);
#50843=ADVANCED_FACE('',(#15756),#13154,.F.);
#50844=ADVANCED_FACE('',(#15757),#13155,.T.);
#50845=ADVANCED_FACE('',(#15758),#13156,.F.);
#50846=ADVANCED_FACE('',(#15759),#13157,.F.);
#50847=ADVANCED_FACE('',(#15760),#13158,.F.);
#50848=ADVANCED_FACE('',(#15761),#13159,.T.);
#50849=ADVANCED_FACE('',(#15762),#13160,.F.);
#50850=ADVANCED_FACE('',(#15763),#13161,.F.);
#50851=ADVANCED_FACE('',(#15764),#13162,.F.);
#50852=ADVANCED_FACE('',(#15765),#13163,.T.);
#50853=ADVANCED_FACE('',(#15766),#13164,.F.);
#50854=ADVANCED_FACE('',(#15767),#13165,.F.);
#50855=ADVANCED_FACE('',(#15768),#13166,.F.);
#50856=ADVANCED_FACE('',(#15769),#13167,.T.);
#50857=ADVANCED_FACE('',(#15770),#13168,.F.);
#50858=ADVANCED_FACE('',(#15771),#13169,.F.);
#50859=ADVANCED_FACE('',(#15772),#13170,.F.);
#50860=ADVANCED_FACE('',(#15773),#13171,.T.);
#50861=ADVANCED_FACE('',(#15774),#13172,.F.);
#50862=ADVANCED_FACE('',(#15775),#13173,.F.);
#50863=ADVANCED_FACE('',(#15776),#13174,.F.);
#50864=ADVANCED_FACE('',(#15777),#13175,.T.);
#50865=ADVANCED_FACE('',(#15778),#13176,.F.);
#50866=ADVANCED_FACE('',(#15779),#13177,.F.);
#50867=ADVANCED_FACE('',(#15780),#13178,.F.);
#50868=ADVANCED_FACE('',(#15781),#13179,.T.);
#50869=ADVANCED_FACE('',(#15782),#13180,.F.);
#50870=ADVANCED_FACE('',(#15783),#13181,.F.);
#50871=ADVANCED_FACE('',(#15784),#13182,.F.);
#50872=ADVANCED_FACE('',(#15785),#13183,.T.);
#50873=ADVANCED_FACE('',(#15786),#13184,.F.);
#50874=ADVANCED_FACE('',(#15787),#13185,.F.);
#50875=ADVANCED_FACE('',(#15788),#13186,.F.);
#50876=ADVANCED_FACE('',(#15789),#13187,.T.);
#50877=ADVANCED_FACE('',(#15790),#13188,.F.);
#50878=ADVANCED_FACE('',(#15791),#13189,.F.);
#50879=ADVANCED_FACE('',(#15792),#13190,.F.);
#50880=ADVANCED_FACE('',(#15793),#13191,.T.);
#50881=ADVANCED_FACE('',(#15794),#13192,.F.);
#50882=ADVANCED_FACE('',(#15795),#13193,.F.);
#50883=ADVANCED_FACE('',(#15796),#13194,.F.);
#50884=ADVANCED_FACE('',(#15797),#13195,.T.);
#50885=ADVANCED_FACE('',(#15798),#13196,.F.);
#50886=ADVANCED_FACE('',(#15799),#13197,.F.);
#50887=ADVANCED_FACE('',(#15800),#13198,.F.);
#50888=ADVANCED_FACE('',(#15801),#13199,.T.);
#50889=ADVANCED_FACE('',(#15802),#13200,.F.);
#50890=ADVANCED_FACE('',(#15803),#13201,.F.);
#50891=ADVANCED_FACE('',(#15804),#13202,.F.);
#50892=ADVANCED_FACE('',(#15805),#13203,.T.);
#50893=ADVANCED_FACE('',(#15806),#13204,.F.);
#50894=ADVANCED_FACE('',(#15807),#13205,.F.);
#50895=ADVANCED_FACE('',(#15808),#13206,.F.);
#50896=ADVANCED_FACE('',(#15809),#13207,.T.);
#50897=ADVANCED_FACE('',(#15810),#13208,.F.);
#50898=ADVANCED_FACE('',(#15811),#13209,.F.);
#50899=ADVANCED_FACE('',(#15812),#13210,.F.);
#50900=ADVANCED_FACE('',(#15813),#13211,.T.);
#50901=ADVANCED_FACE('',(#15814),#48317,.F.);
#50902=ADVANCED_FACE('',(#15815),#13212,.F.);
#50903=ADVANCED_FACE('',(#15816),#13213,.F.);
#50904=ADVANCED_FACE('',(#15817),#13214,.F.);
#50905=ADVANCED_FACE('',(#15818),#13215,.F.);
#50906=ADVANCED_FACE('',(#15819),#13216,.F.);
#50907=ADVANCED_FACE('',(#15820),#13217,.F.);
#50908=ADVANCED_FACE('',(#15821,#1036),#13218,.T.);
#50909=ADVANCED_FACE('',(#15822),#13219,.T.);
#50910=ADVANCED_FACE('',(#15823),#48318,.T.);
#50911=ADVANCED_FACE('',(#15824),#1231,.T.);
#50912=ADVANCED_FACE('',(#15825),#48319,.T.);
#50913=ADVANCED_FACE('',(#15826,#1037),#13220,.T.);
#51026=CLOSED_SHELL('',(#50718,#50719,#50720,#50721,#50722,#50723,#50724,
#50725,#50726,#50727,#50728,#50729,#50730,#50731,#50732,#50733,#50734,#50735,
#50736,#50737,#50738,#50739,#50740,#50741,#50742,#50743,#50744,#50745,#50746,
#50747,#50748,#50749,#50750,#50751,#50752,#50753,#50754,#50755,#50756,#50757,
#50758,#50759,#50760,#50761,#50762,#50763,#50764,#50765,#50766,#50767,#50768,
#50769,#50770,#50771,#50772,#50773,#50774,#50775,#50776,#50777,#50778,#50779,
#50780,#50781,#50782,#50783,#50784,#50785,#50786,#50787,#50788,#50789,#50790,
#50791,#50792,#50793,#50794,#50795,#50796,#50797,#50798,#50799,#50800,#50801,
#50802,#50803,#50804,#50805,#50806,#50807,#50808,#50809,#50810,#50811,#50812,
#50813,#50814,#50815,#50816,#50817,#50818,#50819,#50820,#50821,#50822,#50823,
#50824,#50825,#50826,#50827,#50828,#50829,#50830,#50831,#50832,#50833,#50834,
#50835,#50836,#50837,#50838,#50839,#50840,#50841,#50842,#50843,#50844,#50845,
#50846,#50847,#50848,#50849,#50850,#50851,#50852,#50853,#50854,#50855,#50856,
#50857,#50858,#50859,#50860,#50861,#50862,#50863,#50864,#50865,#50866,#50867,
#50868,#50869,#50870,#50871,#50872,#50873,#50874,#50875,#50876,#50877,#50878,
#50879,#50880,#50881,#50882,#50883,#50884,#50885,#50886,#50887,#50888,#50889,
#50890,#50891,#50892,#50893,#50894,#50895,#50896,#50897,#50898,#50899,#50900,
#50901,#50902,#50903,#50904,#50905,#50906,#50907,#50908,#50909,#50910,#50911,
#50912,#50913));
#54858=AXIS2_PLACEMENT_3D('',#87476,#66847,#66848);
#54859=AXIS2_PLACEMENT_3D('',#87477,#66849,#66850);
#54860=AXIS2_PLACEMENT_3D('',#87493,#66852,#66853);
#54861=AXIS2_PLACEMENT_3D('',#87501,#66854,#66855);
#54862=AXIS2_PLACEMENT_3D('',#87549,#66857,#66858);
#54863=AXIS2_PLACEMENT_3D('',#87597,#66860,#66861);
#54864=AXIS2_PLACEMENT_3D('',#87651,#66863,#66864);
#54865=AXIS2_PLACEMENT_3D('',#87699,#66866,#66867);
#54866=AXIS2_PLACEMENT_3D('',#87747,#66869,#66870);
#54867=AXIS2_PLACEMENT_3D('',#87795,#66872,#66873);
#54868=AXIS2_PLACEMENT_3D('',#87849,#66875,#66876);
#54869=AXIS2_PLACEMENT_3D('',#87897,#66878,#66879);
#54870=AXIS2_PLACEMENT_3D('',#87945,#66881,#66882);
#54871=AXIS2_PLACEMENT_3D('',#87999,#66884,#66885);
#54872=AXIS2_PLACEMENT_3D('',#88047,#66887,#66888);
#54873=AXIS2_PLACEMENT_3D('',#88095,#66890,#66891);
#54874=AXIS2_PLACEMENT_3D('',#88149,#66893,#66894);
#54875=AXIS2_PLACEMENT_3D('',#88197,#66896,#66897);
#54876=AXIS2_PLACEMENT_3D('',#88202,#66899,#66900);
#54877=AXIS2_PLACEMENT_3D('',#88244,#66901,#66902);
#54878=AXIS2_PLACEMENT_3D('',#88257,#66904,#66905);
#54879=AXIS2_PLACEMENT_3D('',#88264,#66906,#66907);
#54880=AXIS2_PLACEMENT_3D('',#88288,#66909,#66910);
#54881=AXIS2_PLACEMENT_3D('',#88313,#66912,#66913);
#54882=AXIS2_PLACEMENT_3D('',#88338,#66915,#66916);
#54883=AXIS2_PLACEMENT_3D('',#88362,#66918,#66919);
#54884=AXIS2_PLACEMENT_3D('',#88387,#66921,#66922);
#54885=AXIS2_PLACEMENT_3D('',#88412,#66924,#66925);
#54886=AXIS2_PLACEMENT_3D('',#88436,#66927,#66928);
#54887=AXIS2_PLACEMENT_3D('',#88461,#66930,#66931);
#54888=AXIS2_PLACEMENT_3D('',#88486,#66933,#66934);
#54889=AXIS2_PLACEMENT_3D('',#88510,#66936,#66937);
#54890=AXIS2_PLACEMENT_3D('',#88534,#66939,#66940);
#54891=AXIS2_PLACEMENT_3D('',#88559,#66942,#66943);
#54892=AXIS2_PLACEMENT_3D('',#88584,#66945,#66946);
#54893=AXIS2_PLACEMENT_3D('',#88608,#66948,#66949);
#54894=AXIS2_PLACEMENT_3D('',#88701,#66950,#66951);
#54895=AXIS2_PLACEMENT_3D('',#88703,#66952,#66953);
#54896=AXIS2_PLACEMENT_3D('',#89307,#66954,#66955);
#54897=AXIS2_PLACEMENT_3D('',#89309,#66956,#66957);
#54898=AXIS2_PLACEMENT_3D('',#89310,#66958,#66959);
#54899=AXIS2_PLACEMENT_3D('',#89406,#66960,#66961);
#54900=AXIS2_PLACEMENT_3D('',#89407,#66962,#66963);
#54901=AXIS2_PLACEMENT_3D('',#89820,#66964,#66965);
#54902=AXIS2_PLACEMENT_3D('',#89821,#66966,#66967);
#54903=AXIS2_PLACEMENT_3D('',#89823,#66968,#66969);
#54904=AXIS2_PLACEMENT_3D('',#89824,#66970,#66971);
#54905=AXIS2_PLACEMENT_3D('',#89825,#66972,#66973);
#54906=AXIS2_PLACEMENT_3D('',#89826,#66974,#66975);
#54907=AXIS2_PLACEMENT_3D('',#89828,#66976,#66977);
#54908=AXIS2_PLACEMENT_3D('',#89829,#66978,#66979);
#54909=AXIS2_PLACEMENT_3D('',#89838,#66984,#66985);
#54910=AXIS2_PLACEMENT_3D('',#89840,#66986,#66987);
#54911=AXIS2_PLACEMENT_3D('',#89842,#66989,#66990);
#54912=AXIS2_PLACEMENT_3D('',#89846,#66993,#66994);
#54913=AXIS2_PLACEMENT_3D('',#89847,#66995,#66996);
#54914=AXIS2_PLACEMENT_3D('',#89848,#66997,#66998);
#54915=AXIS2_PLACEMENT_3D('',#89857,#67003,#67004);
#54916=AXIS2_PLACEMENT_3D('',#89859,#67005,#67006);
#54917=AXIS2_PLACEMENT_3D('',#89861,#67008,#67009);
#54918=AXIS2_PLACEMENT_3D('',#89865,#67012,#67013);
#54919=AXIS2_PLACEMENT_3D('',#89866,#67014,#67015);
#54920=AXIS2_PLACEMENT_3D('',#89867,#67016,#67017);
#54921=AXIS2_PLACEMENT_3D('',#89876,#67022,#67023);
#54922=AXIS2_PLACEMENT_3D('',#89878,#67024,#67025);
#54923=AXIS2_PLACEMENT_3D('',#89880,#67027,#67028);
#54924=AXIS2_PLACEMENT_3D('',#89884,#67031,#67032);
#54925=AXIS2_PLACEMENT_3D('',#89885,#67033,#67034);
#54926=AXIS2_PLACEMENT_3D('',#89886,#67035,#67036);
#54927=AXIS2_PLACEMENT_3D('',#89895,#67041,#67042);
#54928=AXIS2_PLACEMENT_3D('',#89897,#67043,#67044);
#54929=AXIS2_PLACEMENT_3D('',#89899,#67046,#67047);
#54930=AXIS2_PLACEMENT_3D('',#89903,#67050,#67051);
#54931=AXIS2_PLACEMENT_3D('',#89904,#67052,#67053);
#54932=AXIS2_PLACEMENT_3D('',#89905,#67054,#67055);
#54933=AXIS2_PLACEMENT_3D('',#89914,#67060,#67061);
#54934=AXIS2_PLACEMENT_3D('',#89916,#67062,#67063);
#54935=AXIS2_PLACEMENT_3D('',#89918,#67065,#67066);
#54936=AXIS2_PLACEMENT_3D('',#89922,#67069,#67070);
#54937=AXIS2_PLACEMENT_3D('',#89923,#67071,#67072);
#54938=AXIS2_PLACEMENT_3D('',#89924,#67073,#67074);
#54939=AXIS2_PLACEMENT_3D('',#89933,#67079,#67080);
#54940=AXIS2_PLACEMENT_3D('',#89935,#67081,#67082);
#54941=AXIS2_PLACEMENT_3D('',#89937,#67084,#67085);
#54942=AXIS2_PLACEMENT_3D('',#89941,#67088,#67089);
#54943=AXIS2_PLACEMENT_3D('',#89942,#67090,#67091);
#54944=AXIS2_PLACEMENT_3D('',#89943,#67092,#67093);
#54945=AXIS2_PLACEMENT_3D('',#89952,#67098,#67099);
#54946=AXIS2_PLACEMENT_3D('',#89954,#67100,#67101);
#54947=AXIS2_PLACEMENT_3D('',#89956,#67103,#67104);
#54948=AXIS2_PLACEMENT_3D('',#89960,#67107,#67108);
#54949=AXIS2_PLACEMENT_3D('',#89961,#67109,#67110);
#54950=AXIS2_PLACEMENT_3D('',#89962,#67111,#67112);
#54951=AXIS2_PLACEMENT_3D('',#89971,#67117,#67118);
#54952=AXIS2_PLACEMENT_3D('',#89973,#67119,#67120);
#54953=AXIS2_PLACEMENT_3D('',#89975,#67122,#67123);
#54954=AXIS2_PLACEMENT_3D('',#89979,#67126,#67127);
#54955=AXIS2_PLACEMENT_3D('',#89980,#67128,#67129);
#54956=AXIS2_PLACEMENT_3D('',#89981,#67130,#67131);
#54957=AXIS2_PLACEMENT_3D('',#89990,#67136,#67137);
#54958=AXIS2_PLACEMENT_3D('',#89992,#67138,#67139);
#54959=AXIS2_PLACEMENT_3D('',#89994,#67141,#67142);
#54960=AXIS2_PLACEMENT_3D('',#89998,#67145,#67146);
#54961=AXIS2_PLACEMENT_3D('',#89999,#67147,#67148);
#54962=AXIS2_PLACEMENT_3D('',#90000,#67149,#67150);
#54963=AXIS2_PLACEMENT_3D('',#90009,#67155,#67156);
#54964=AXIS2_PLACEMENT_3D('',#90011,#67157,#67158);
#54965=AXIS2_PLACEMENT_3D('',#90013,#67160,#67161);
#54966=AXIS2_PLACEMENT_3D('',#90017,#67164,#67165);
#54967=AXIS2_PLACEMENT_3D('',#90018,#67166,#67167);
#54968=AXIS2_PLACEMENT_3D('',#90019,#67168,#67169);
#54969=AXIS2_PLACEMENT_3D('',#90028,#67174,#67175);
#54970=AXIS2_PLACEMENT_3D('',#90030,#67176,#67177);
#54971=AXIS2_PLACEMENT_3D('',#90032,#67179,#67180);
#54972=AXIS2_PLACEMENT_3D('',#90036,#67183,#67184);
#54973=AXIS2_PLACEMENT_3D('',#90037,#67185,#67186);
#54974=AXIS2_PLACEMENT_3D('',#90038,#67187,#67188);
#54975=AXIS2_PLACEMENT_3D('',#90047,#67193,#67194);
#54976=AXIS2_PLACEMENT_3D('',#90049,#67195,#67196);
#54977=AXIS2_PLACEMENT_3D('',#90051,#67198,#67199);
#54978=AXIS2_PLACEMENT_3D('',#90055,#67202,#67203);
#54979=AXIS2_PLACEMENT_3D('',#90056,#67204,#67205);
#54980=AXIS2_PLACEMENT_3D('',#90057,#67206,#67207);
#54981=AXIS2_PLACEMENT_3D('',#90066,#67212,#67213);
#54982=AXIS2_PLACEMENT_3D('',#90068,#67214,#67215);
#54983=AXIS2_PLACEMENT_3D('',#90070,#67217,#67218);
#54984=AXIS2_PLACEMENT_3D('',#90074,#67221,#67222);
#54985=AXIS2_PLACEMENT_3D('',#90075,#67223,#67224);
#54986=AXIS2_PLACEMENT_3D('',#90076,#67225,#67226);
#54987=AXIS2_PLACEMENT_3D('',#90085,#67231,#67232);
#54988=AXIS2_PLACEMENT_3D('',#90087,#67233,#67234);
#54989=AXIS2_PLACEMENT_3D('',#90089,#67236,#67237);
#54990=AXIS2_PLACEMENT_3D('',#90093,#67240,#67241);
#54991=AXIS2_PLACEMENT_3D('',#90094,#67242,#67243);
#54992=AXIS2_PLACEMENT_3D('',#90095,#67244,#67245);
#54993=AXIS2_PLACEMENT_3D('',#90104,#67250,#67251);
#54994=AXIS2_PLACEMENT_3D('',#90106,#67252,#67253);
#54995=AXIS2_PLACEMENT_3D('',#90108,#67255,#67256);
#54996=AXIS2_PLACEMENT_3D('',#90112,#67259,#67260);
#54997=AXIS2_PLACEMENT_3D('',#90113,#67261,#67262);
#54998=AXIS2_PLACEMENT_3D('',#90114,#67263,#67264);
#54999=AXIS2_PLACEMENT_3D('',#90123,#67269,#67270);
#55000=AXIS2_PLACEMENT_3D('',#90125,#67271,#67272);
#55001=AXIS2_PLACEMENT_3D('',#90127,#67274,#67275);
#55002=AXIS2_PLACEMENT_3D('',#90131,#67278,#67279);
#55003=AXIS2_PLACEMENT_3D('',#90132,#67280,#67281);
#55004=AXIS2_PLACEMENT_3D('',#90133,#67282,#67283);
#55005=AXIS2_PLACEMENT_3D('',#90142,#67288,#67289);
#55006=AXIS2_PLACEMENT_3D('',#90144,#67290,#67291);
#55007=AXIS2_PLACEMENT_3D('',#90146,#67293,#67294);
#55008=AXIS2_PLACEMENT_3D('',#90150,#67297,#67298);
#55009=AXIS2_PLACEMENT_3D('',#90151,#67299,#67300);
#55010=AXIS2_PLACEMENT_3D('',#90152,#67301,#67302);
#55011=AXIS2_PLACEMENT_3D('',#90161,#67307,#67308);
#55012=AXIS2_PLACEMENT_3D('',#90163,#67309,#67310);
#55013=AXIS2_PLACEMENT_3D('',#90166,#67312,#67313);
#55014=AXIS2_PLACEMENT_3D('',#90167,#67314,#67315);
#55015=AXIS2_PLACEMENT_3D('',#90171,#67318,#67319);
#55016=AXIS2_PLACEMENT_3D('',#90173,#67320,#67321);
#55017=AXIS2_PLACEMENT_3D('',#90174,#67322,#67323);
#55018=AXIS2_PLACEMENT_3D('',#90175,#67324,#67325);
#55019=AXIS2_PLACEMENT_3D('',#90184,#67330,#67331);
#55020=AXIS2_PLACEMENT_3D('',#90186,#67332,#67333);
#55021=AXIS2_PLACEMENT_3D('',#90188,#67335,#67336);
#55022=AXIS2_PLACEMENT_3D('',#90192,#67339,#67340);
#55023=AXIS2_PLACEMENT_3D('',#90193,#67341,#67342);
#55024=AXIS2_PLACEMENT_3D('',#90194,#67343,#67344);
#55025=AXIS2_PLACEMENT_3D('',#90203,#67349,#67350);
#55026=AXIS2_PLACEMENT_3D('',#90205,#67351,#67352);
#55027=AXIS2_PLACEMENT_3D('',#90207,#67354,#67355);
#55028=AXIS2_PLACEMENT_3D('',#90211,#67358,#67359);
#55029=AXIS2_PLACEMENT_3D('',#90212,#67360,#67361);
#55030=AXIS2_PLACEMENT_3D('',#90213,#67362,#67363);
#55031=AXIS2_PLACEMENT_3D('',#90222,#67368,#67369);
#55032=AXIS2_PLACEMENT_3D('',#90224,#67370,#67371);
#55033=AXIS2_PLACEMENT_3D('',#90226,#67373,#67374);
#55034=AXIS2_PLACEMENT_3D('',#90230,#67377,#67378);
#55035=AXIS2_PLACEMENT_3D('',#90231,#67379,#67380);
#55036=AXIS2_PLACEMENT_3D('',#90232,#67381,#67382);
#55037=AXIS2_PLACEMENT_3D('',#90241,#67387,#67388);
#55038=AXIS2_PLACEMENT_3D('',#90243,#67389,#67390);
#55039=AXIS2_PLACEMENT_3D('',#90245,#67392,#67393);
#55040=AXIS2_PLACEMENT_3D('',#90249,#67396,#67397);
#55041=AXIS2_PLACEMENT_3D('',#90250,#67398,#67399);
#55042=AXIS2_PLACEMENT_3D('',#90251,#67400,#67401);
#55043=AXIS2_PLACEMENT_3D('',#90260,#67406,#67407);
#55044=AXIS2_PLACEMENT_3D('',#90262,#67408,#67409);
#55045=AXIS2_PLACEMENT_3D('',#90264,#67411,#67412);
#55046=AXIS2_PLACEMENT_3D('',#90268,#67415,#67416);
#55047=AXIS2_PLACEMENT_3D('',#90269,#67417,#67418);
#55048=AXIS2_PLACEMENT_3D('',#90270,#67419,#67420);
#55049=AXIS2_PLACEMENT_3D('',#90279,#67425,#67426);
#55050=AXIS2_PLACEMENT_3D('',#90281,#67427,#67428);
#55051=AXIS2_PLACEMENT_3D('',#90283,#67430,#67431);
#55052=AXIS2_PLACEMENT_3D('',#90287,#67434,#67435);
#55053=AXIS2_PLACEMENT_3D('',#90288,#67436,#67437);
#55054=AXIS2_PLACEMENT_3D('',#90289,#67438,#67439);
#55055=AXIS2_PLACEMENT_3D('',#90298,#67444,#67445);
#55056=AXIS2_PLACEMENT_3D('',#90300,#67446,#67447);
#55057=AXIS2_PLACEMENT_3D('',#90302,#67449,#67450);
#55058=AXIS2_PLACEMENT_3D('',#90306,#67453,#67454);
#55059=AXIS2_PLACEMENT_3D('',#90307,#67455,#67456);
#55060=AXIS2_PLACEMENT_3D('',#90308,#67457,#67458);
#55061=AXIS2_PLACEMENT_3D('',#90317,#67463,#67464);
#55062=AXIS2_PLACEMENT_3D('',#90319,#67465,#67466);
#55063=AXIS2_PLACEMENT_3D('',#90321,#67468,#67469);
#55064=AXIS2_PLACEMENT_3D('',#90325,#67472,#67473);
#55065=AXIS2_PLACEMENT_3D('',#90326,#67474,#67475);
#55066=AXIS2_PLACEMENT_3D('',#90327,#67476,#67477);
#55067=AXIS2_PLACEMENT_3D('',#90336,#67482,#67483);
#55068=AXIS2_PLACEMENT_3D('',#90338,#67484,#67485);
#55069=AXIS2_PLACEMENT_3D('',#90340,#67487,#67488);
#55070=AXIS2_PLACEMENT_3D('',#90344,#67491,#67492);
#55071=AXIS2_PLACEMENT_3D('',#90345,#67493,#67494);
#55072=AXIS2_PLACEMENT_3D('',#90346,#67495,#67496);
#55073=AXIS2_PLACEMENT_3D('',#90355,#67501,#67502);
#55074=AXIS2_PLACEMENT_3D('',#90357,#67503,#67504);
#55075=AXIS2_PLACEMENT_3D('',#90359,#67506,#67507);
#55076=AXIS2_PLACEMENT_3D('',#90363,#67510,#67511);
#55077=AXIS2_PLACEMENT_3D('',#90364,#67512,#67513);
#55078=AXIS2_PLACEMENT_3D('',#90365,#67514,#67515);
#55079=AXIS2_PLACEMENT_3D('',#90374,#67520,#67521);
#55080=AXIS2_PLACEMENT_3D('',#90376,#67522,#67523);
#55081=AXIS2_PLACEMENT_3D('',#90378,#67525,#67526);
#55082=AXIS2_PLACEMENT_3D('',#90382,#67529,#67530);
#55083=AXIS2_PLACEMENT_3D('',#90383,#67531,#67532);
#55084=AXIS2_PLACEMENT_3D('',#90384,#67533,#67534);
#55085=AXIS2_PLACEMENT_3D('',#90393,#67539,#67540);
#55086=AXIS2_PLACEMENT_3D('',#90395,#67541,#67542);
#55087=AXIS2_PLACEMENT_3D('',#90397,#67544,#67545);
#55088=AXIS2_PLACEMENT_3D('',#90401,#67548,#67549);
#55089=AXIS2_PLACEMENT_3D('',#90402,#67550,#67551);
#55090=AXIS2_PLACEMENT_3D('',#90403,#67552,#67553);
#55091=AXIS2_PLACEMENT_3D('',#90412,#67558,#67559);
#55092=AXIS2_PLACEMENT_3D('',#90414,#67560,#67561);
#55093=AXIS2_PLACEMENT_3D('',#90416,#67563,#67564);
#55094=AXIS2_PLACEMENT_3D('',#90420,#67567,#67568);
#55095=AXIS2_PLACEMENT_3D('',#90421,#67569,#67570);
#55096=AXIS2_PLACEMENT_3D('',#90422,#67571,#67572);
#55097=AXIS2_PLACEMENT_3D('',#90431,#67577,#67578);
#55098=AXIS2_PLACEMENT_3D('',#90433,#67579,#67580);
#55099=AXIS2_PLACEMENT_3D('',#90435,#67582,#67583);
#55100=AXIS2_PLACEMENT_3D('',#90439,#67586,#67587);
#55101=AXIS2_PLACEMENT_3D('',#90440,#67588,#67589);
#55102=AXIS2_PLACEMENT_3D('',#90441,#67590,#67591);
#55103=AXIS2_PLACEMENT_3D('',#90450,#67596,#67597);
#55104=AXIS2_PLACEMENT_3D('',#90452,#67598,#67599);
#55105=AXIS2_PLACEMENT_3D('',#90454,#67601,#67602);
#55106=AXIS2_PLACEMENT_3D('',#90458,#67605,#67606);
#55107=AXIS2_PLACEMENT_3D('',#90459,#67607,#67608);
#55108=AXIS2_PLACEMENT_3D('',#90460,#67609,#67610);
#55109=AXIS2_PLACEMENT_3D('',#90469,#67615,#67616);
#55110=AXIS2_PLACEMENT_3D('',#90471,#67617,#67618);
#55111=AXIS2_PLACEMENT_3D('',#90473,#67620,#67621);
#55112=AXIS2_PLACEMENT_3D('',#90477,#67624,#67625);
#55113=AXIS2_PLACEMENT_3D('',#90478,#67626,#67627);
#55114=AXIS2_PLACEMENT_3D('',#90479,#67628,#67629);
#55115=AXIS2_PLACEMENT_3D('',#90488,#67634,#67635);
#55116=AXIS2_PLACEMENT_3D('',#90490,#67636,#67637);
#55117=AXIS2_PLACEMENT_3D('',#90492,#67639,#67640);
#55118=AXIS2_PLACEMENT_3D('',#90496,#67643,#67644);
#55119=AXIS2_PLACEMENT_3D('',#90497,#67645,#67646);
#55120=AXIS2_PLACEMENT_3D('',#90498,#67647,#67648);
#55121=AXIS2_PLACEMENT_3D('',#90501,#67649,#67650);
#55122=AXIS2_PLACEMENT_3D('',#90505,#67653,#67654);
#55123=AXIS2_PLACEMENT_3D('',#90511,#67658,#67659);
#55124=AXIS2_PLACEMENT_3D('',#90515,#67662,#67663);
#55125=AXIS2_PLACEMENT_3D('',#90516,#67664,#67665);
#55126=AXIS2_PLACEMENT_3D('',#90517,#67666,#67667);
#55127=AXIS2_PLACEMENT_3D('',#90521,#67669,#67670);
#55128=AXIS2_PLACEMENT_3D('',#90522,#67671,#67672);
#55129=AXIS2_PLACEMENT_3D('',#90531,#67677,#67678);
#55130=AXIS2_PLACEMENT_3D('',#90537,#67682,#67683);
#55131=AXIS2_PLACEMENT_3D('',#90543,#67687,#67688);
#55132=AXIS2_PLACEMENT_3D('',#90549,#67692,#67693);
#55133=AXIS2_PLACEMENT_3D('',#90555,#67697,#67698);
#55134=AXIS2_PLACEMENT_3D('',#90558,#67701,#67702);
#55135=AXIS2_PLACEMENT_3D('',#90559,#67703,#67704);
#55136=AXIS2_PLACEMENT_3D('',#90561,#67705,#67706);
#55137=AXIS2_PLACEMENT_3D('',#90562,#67707,#67708);
#55138=AXIS2_PLACEMENT_3D('',#90564,#67710,#67711);
#55139=AXIS2_PLACEMENT_3D('',#90565,#67712,#67713);
#55140=AXIS2_PLACEMENT_3D('',#90566,#67714,#67715);
#55141=AXIS2_PLACEMENT_3D('',#90567,#67716,#67717);
#55142=AXIS2_PLACEMENT_3D('',#90568,#67718,#67719);
#55143=AXIS2_PLACEMENT_3D('',#90569,#67720,#67721);
#55144=AXIS2_PLACEMENT_3D('',#90570,#67722,#67723);
#55145=AXIS2_PLACEMENT_3D('',#90571,#67724,#67725);
#55146=AXIS2_PLACEMENT_3D('',#90572,#67726,#67727);
#55147=AXIS2_PLACEMENT_3D('',#90573,#67728,#67729);
#55148=AXIS2_PLACEMENT_3D('',#90574,#67730,#67731);
#55149=AXIS2_PLACEMENT_3D('',#90575,#67732,#67733);
#55150=AXIS2_PLACEMENT_3D('',#90576,#67734,#67735);
#55151=AXIS2_PLACEMENT_3D('',#90577,#67736,#67737);
#55152=AXIS2_PLACEMENT_3D('',#90578,#67738,#67739);
#55153=AXIS2_PLACEMENT_3D('',#90579,#67740,#67741);
#55154=AXIS2_PLACEMENT_3D('',#90580,#67742,#67743);
#55155=AXIS2_PLACEMENT_3D('',#90581,#67744,#67745);
#55156=AXIS2_PLACEMENT_3D('',#90583,#67747,#67748);
#55157=AXIS2_PLACEMENT_3D('',#90584,#67749,#67750);
#55158=AXIS2_PLACEMENT_3D('',#90585,#67751,#67752);
#55159=AXIS2_PLACEMENT_3D('',#90586,#67753,#67754);
#55160=AXIS2_PLACEMENT_3D('',#90587,#67755,#67756);
#55161=AXIS2_PLACEMENT_3D('',#90588,#67757,#67758);
#55162=AXIS2_PLACEMENT_3D('',#90589,#67759,#67760);
#55163=AXIS2_PLACEMENT_3D('',#90590,#67761,#67762);
#55164=AXIS2_PLACEMENT_3D('',#90591,#67763,#67764);
#55165=AXIS2_PLACEMENT_3D('',#90592,#67765,#67766);
#55166=AXIS2_PLACEMENT_3D('',#90593,#67767,#67768);
#55167=AXIS2_PLACEMENT_3D('',#90594,#67769,#67770);
#55168=AXIS2_PLACEMENT_3D('',#90595,#67771,#67772);
#55169=AXIS2_PLACEMENT_3D('',#90596,#67773,#67774);
#55170=AXIS2_PLACEMENT_3D('',#90597,#67775,#67776);
#55171=AXIS2_PLACEMENT_3D('',#90598,#67777,#67778);
#55172=AXIS2_PLACEMENT_3D('',#90599,#67779,#67780);
#55173=AXIS2_PLACEMENT_3D('',#90600,#67781,#67782);
#55174=AXIS2_PLACEMENT_3D('',#90601,#67783,#67784);
#55175=AXIS2_PLACEMENT_3D('',#90602,#67785,#67786);
#55176=AXIS2_PLACEMENT_3D('',#90604,#67787,#67788);
#55177=AXIS2_PLACEMENT_3D('',#90606,#67790,#67791);
#66847=DIRECTION('axis',(0.,0.,1.));
#66848=DIRECTION('refdir',(1.,0.,0.));
#66849=DIRECTION('center_axis',(1.,0.,0.));
#66850=DIRECTION('ref_axis',(0.,1.,0.));
#66851=DIRECTION('',(-1.,0.,0.));
#66852=DIRECTION('center_axis',(1.,0.,0.));
#66853=DIRECTION('ref_axis',(0.,1.,0.));
#66854=DIRECTION('center_axis',(1.,0.,0.));
#66855=DIRECTION('ref_axis',(0.,1.,0.));
#66856=DIRECTION('',(-1.,0.,0.));
#66857=DIRECTION('center_axis',(1.,0.,0.));
#66858=DIRECTION('ref_axis',(0.,1.,0.));
#66859=DIRECTION('',(-1.,0.,0.));
#66860=DIRECTION('center_axis',(1.,0.,0.));
#66861=DIRECTION('ref_axis',(0.,1.,0.));
#66862=DIRECTION('',(-1.,0.,0.));
#66863=DIRECTION('center_axis',(1.,0.,0.));
#66864=DIRECTION('ref_axis',(0.,1.,0.));
#66865=DIRECTION('',(-1.,0.,0.));
#66866=DIRECTION('center_axis',(1.,0.,0.));
#66867=DIRECTION('ref_axis',(0.,1.,0.));
#66868=DIRECTION('',(-1.,0.,0.));
#66869=DIRECTION('center_axis',(1.,0.,0.));
#66870=DIRECTION('ref_axis',(0.,1.,0.));
#66871=DIRECTION('',(-1.,0.,0.));
#66872=DIRECTION('center_axis',(1.,0.,0.));
#66873=DIRECTION('ref_axis',(0.,1.,0.));
#66874=DIRECTION('',(-1.,0.,0.));
#66875=DIRECTION('center_axis',(1.,0.,0.));
#66876=DIRECTION('ref_axis',(0.,1.,0.));
#66877=DIRECTION('',(-1.,0.,0.));
#66878=DIRECTION('center_axis',(1.,0.,0.));
#66879=DIRECTION('ref_axis',(0.,1.,0.));
#66880=DIRECTION('',(-1.,0.,0.));
#66881=DIRECTION('center_axis',(1.,0.,0.));
#66882=DIRECTION('ref_axis',(0.,1.,0.));
#66883=DIRECTION('',(-1.,0.,0.));
#66884=DIRECTION('center_axis',(1.,0.,0.));
#66885=DIRECTION('ref_axis',(0.,1.,0.));
#66886=DIRECTION('',(-1.,0.,0.));
#66887=DIRECTION('center_axis',(1.,0.,0.));
#66888=DIRECTION('ref_axis',(0.,1.,0.));
#66889=DIRECTION('',(-1.,0.,0.));
#66890=DIRECTION('center_axis',(1.,0.,0.));
#66891=DIRECTION('ref_axis',(0.,1.,0.));
#66892=DIRECTION('',(-1.,0.,0.));
#66893=DIRECTION('center_axis',(1.,0.,0.));
#66894=DIRECTION('ref_axis',(0.,1.,0.));
#66895=DIRECTION('',(-1.,0.,0.));
#66896=DIRECTION('center_axis',(1.,0.,0.));
#66897=DIRECTION('ref_axis',(0.,1.,0.));
#66898=DIRECTION('',(-1.,0.,0.));
#66899=DIRECTION('center_axis',(1.,0.,0.));
#66900=DIRECTION('ref_axis',(0.,1.,0.));
#66901=DIRECTION('center_axis',(1.,0.,0.));
#66902=DIRECTION('ref_axis',(0.,0.1768138132289,-0.984244316951566));
#66903=DIRECTION('',(1.,0.,0.));
#66904=DIRECTION('center_axis',(1.,0.,0.));
#66905=DIRECTION('ref_axis',(0.,1.,9.72557910080328E-14));
#66906=DIRECTION('center_axis',(1.,0.,0.));
#66907=DIRECTION('ref_axis',(0.,1.,9.72557910080328E-14));
#66908=DIRECTION('',(1.,0.,0.));
#66909=DIRECTION('center_axis',(1.,0.,0.));
#66910=DIRECTION('ref_axis',(0.,1.,9.72557910080328E-14));
#66911=DIRECTION('',(1.,0.,0.));
#66912=DIRECTION('center_axis',(1.,0.,0.));
#66913=DIRECTION('ref_axis',(0.,1.,9.72557910080328E-14));
#66914=DIRECTION('',(1.,0.,0.));
#66915=DIRECTION('center_axis',(1.,0.,0.));
#66916=DIRECTION('ref_axis',(0.,1.,9.72557910080328E-14));
#66917=DIRECTION('',(1.,0.,0.));
#66918=DIRECTION('center_axis',(1.,0.,0.));
#66919=DIRECTION('ref_axis',(0.,1.,9.72557910080328E-14));
#66920=DIRECTION('',(1.,0.,0.));
#66921=DIRECTION('center_axis',(1.,0.,0.));
#66922=DIRECTION('ref_axis',(0.,1.,9.72557910080328E-14));
#66923=DIRECTION('',(1.,0.,0.));
#66924=DIRECTION('center_axis',(1.,0.,0.));
#66925=DIRECTION('ref_axis',(0.,1.,9.72557910080328E-14));
#66926=DIRECTION('',(1.,0.,0.));
#66927=DIRECTION('center_axis',(1.,0.,0.));
#66928=DIRECTION('ref_axis',(0.,1.,9.72557910080328E-14));
#66929=DIRECTION('',(1.,0.,0.));
#66930=DIRECTION('center_axis',(1.,0.,0.));
#66931=DIRECTION('ref_axis',(0.,1.,9.72557910080328E-14));
#66932=DIRECTION('',(1.,0.,0.));
#66933=DIRECTION('center_axis',(1.,0.,0.));
#66934=DIRECTION('ref_axis',(0.,1.,9.72557910080328E-14));
#66935=DIRECTION('',(1.,0.,0.));
#66936=DIRECTION('center_axis',(1.,0.,0.));
#66937=DIRECTION('ref_axis',(0.,1.,9.72557910080328E-14));
#66938=DIRECTION('',(1.,0.,0.));
#66939=DIRECTION('center_axis',(1.,0.,0.));
#66940=DIRECTION('ref_axis',(0.,1.,9.72557910080328E-14));
#66941=DIRECTION('',(1.,0.,0.));
#66942=DIRECTION('center_axis',(1.,0.,0.));
#66943=DIRECTION('ref_axis',(0.,1.,9.72557910080328E-14));
#66944=DIRECTION('',(1.,0.,0.));
#66945=DIRECTION('center_axis',(1.,0.,0.));
#66946=DIRECTION('ref_axis',(0.,1.,9.72557910080328E-14));
#66947=DIRECTION('',(1.,0.,0.));
#66948=DIRECTION('center_axis',(1.,0.,0.));
#66949=DIRECTION('ref_axis',(0.,0.,-1.));
#66950=DIRECTION('center_axis',(1.,0.,0.));
#66951=DIRECTION('ref_axis',(0.,1.,0.));
#66952=DIRECTION('center_axis',(1.,0.,0.));
#66953=DIRECTION('ref_axis',(0.,1.,0.));
#66954=DIRECTION('center_axis',(1.,0.,0.));
#66955=DIRECTION('ref_axis',(0.,0.,-1.));
#66956=DIRECTION('center_axis',(1.,0.,0.));
#66957=DIRECTION('ref_axis',(0.,1.,0.));
#66958=DIRECTION('center_axis',(1.,0.,0.));
#66959=DIRECTION('ref_axis',(0.,1.,0.));
#66960=DIRECTION('center_axis',(-1.,0.,0.));
#66961=DIRECTION('ref_axis',(0.,1.,9.72557910080328E-14));
#66962=DIRECTION('center_axis',(1.,0.,0.));
#66963=DIRECTION('ref_axis',(0.,1.,9.72557910080328E-14));
#66964=DIRECTION('center_axis',(1.,0.,0.));
#66965=DIRECTION('ref_axis',(0.,0.,-1.));
#66966=DIRECTION('center_axis',(1.,0.,0.));
#66967=DIRECTION('ref_axis',(0.,1.,0.));
#66968=DIRECTION('center_axis',(0.,-1.,-1.22464679914735E-16));
#66969=DIRECTION('ref_axis',(0.,-1.22464679914735E-16,1.));
#66970=DIRECTION('center_axis',(-1.,0.,0.));
#66971=DIRECTION('ref_axis',(0.,1.,0.));
#66972=DIRECTION('center_axis',(1.,0.,0.));
#66973=DIRECTION('ref_axis',(0.,1.,0.));
#66974=DIRECTION('center_axis',(-1.,0.,0.));
#66975=DIRECTION('ref_axis',(0.,0.,1.));
#66976=DIRECTION('center_axis',(1.,0.,0.));
#66977=DIRECTION('ref_axis',(0.,0.,-1.));
#66978=DIRECTION('center_axis',(0.,-0.540769022303984,-0.841171126772902));
#66979=DIRECTION('ref_axis',(0.,0.841171126772902,-0.540769022303984));
#66980=DIRECTION('',(1.,0.,0.));
#66981=DIRECTION('',(0.,-0.841171126772902,0.540769022303984));
#66982=DIRECTION('',(1.,0.,0.));
#66983=DIRECTION('',(0.,0.841171126772902,-0.540769022303984));
#66984=DIRECTION('center_axis',(1.,0.,0.));
#66985=DIRECTION('ref_axis',(0.,-0.17364817766693,-0.984807753012208));
#66986=DIRECTION('center_axis',(1.,0.,0.));
#66987=DIRECTION('ref_axis',(0.,0.,-1.));
#66988=DIRECTION('',(0.,-0.975396199161154,-0.220459190468382));
#66989=DIRECTION('center_axis',(0.,-0.220459190468382,0.975396199161154));
#66990=DIRECTION('ref_axis',(0.,-0.975396199161154,-0.220459190468382));
#66991=DIRECTION('',(-1.,0.,0.));
#66992=DIRECTION('',(0.,0.975396199161154,0.220459190468382));
#66993=DIRECTION('center_axis',(1.,0.,0.));
#66994=DIRECTION('ref_axis',(0.,-0.17364817766693,-0.984807753012208));
#66995=DIRECTION('center_axis',(-1.,0.,0.));
#66996=DIRECTION('ref_axis',(0.,1.,0.));
#66997=DIRECTION('center_axis',(0.,-0.678621359023949,-0.734488291994154));
#66998=DIRECTION('ref_axis',(0.,0.734488291994153,-0.678621359023949));
#66999=DIRECTION('',(1.,0.,0.));
#67000=DIRECTION('',(0.,-0.734488291994153,0.678621359023949));
#67001=DIRECTION('',(1.,0.,0.));
#67002=DIRECTION('',(0.,0.734488291994153,-0.678621359023949));
#67003=DIRECTION('center_axis',(1.,0.,0.));
#67004=DIRECTION('ref_axis',(0.,-0.342020143325669,-0.939692620785908));
#67005=DIRECTION('center_axis',(1.,0.,0.));
#67006=DIRECTION('ref_axis',(0.,0.,-1.));
#67007=DIRECTION('',(0.,-0.998860075867306,-0.0477341475084725));
#67008=DIRECTION('center_axis',(0.,-0.0477341475084725,0.998860075867306));
#67009=DIRECTION('ref_axis',(0.,-0.998860075867306,-0.0477341475084725));
#67010=DIRECTION('',(-1.,0.,0.));
#67011=DIRECTION('',(0.,0.998860075867306,0.0477341475084725));
#67012=DIRECTION('center_axis',(1.,0.,0.));
#67013=DIRECTION('ref_axis',(0.,-0.342020143325669,-0.939692620785908));
#67014=DIRECTION('center_axis',(-1.,0.,0.));
#67015=DIRECTION('ref_axis',(0.,1.,0.));
#67016=DIRECTION('center_axis',(0.,-0.795854129148947,-0.605488402132173));
#67017=DIRECTION('ref_axis',(0.,0.605488402132173,-0.795854129148947));
#67018=DIRECTION('',(1.,0.,0.));
#67019=DIRECTION('',(0.,-0.605488402132173,0.795854129148947));
#67020=DIRECTION('',(1.,0.,0.));
#67021=DIRECTION('',(0.,0.605488402132173,-0.795854129148947));
#67022=DIRECTION('center_axis',(1.,0.,0.));
#67023=DIRECTION('ref_axis',(0.,-0.5,-0.866025403784438));
#67024=DIRECTION('center_axis',(1.,0.,0.));
#67025=DIRECTION('ref_axis',(0.,0.,-1.));
#67026=DIRECTION('',(0.,-0.991974094615816,0.126441273368837));
#67027=DIRECTION('center_axis',(0.,0.126441273368837,0.991974094615816));
#67028=DIRECTION('ref_axis',(0.,-0.991974094615816,0.126441273368837));
#67029=DIRECTION('',(-1.,0.,0.));
#67030=DIRECTION('',(0.,0.991974094615816,-0.126441273368837));
#67031=DIRECTION('center_axis',(1.,0.,0.));
#67032=DIRECTION('ref_axis',(0.,-0.5,-0.866025403784438));
#67033=DIRECTION('center_axis',(-1.,0.,0.));
#67034=DIRECTION('ref_axis',(0.,1.,0.));
#67035=DIRECTION('center_axis',(0.,-0.888905274281375,-0.458091053563321));
#67036=DIRECTION('ref_axis',(0.,0.458091053563321,-0.888905274281375));
#67037=DIRECTION('',(1.,0.,0.));
#67038=DIRECTION('',(0.,-0.458091053563321,0.888905274281375));
#67039=DIRECTION('',(1.,0.,0.));
#67040=DIRECTION('',(0.,0.458091053563321,-0.888905274281375));
#67041=DIRECTION('center_axis',(1.,0.,0.));
#67042=DIRECTION('ref_axis',(0.,-0.64278760968654,-0.766044443118978));
#67043=DIRECTION('center_axis',(1.,0.,0.));
#67044=DIRECTION('ref_axis',(0.,0.,-1.));
#67045=DIRECTION('',(0.,-0.954947482462536,0.296774840137206));
#67046=DIRECTION('center_axis',(0.,0.296774840137206,0.954947482462536));
#67047=DIRECTION('ref_axis',(0.,-0.954947482462536,0.296774840137206));
#67048=DIRECTION('',(-1.,0.,0.));
#67049=DIRECTION('',(0.,0.954947482462536,-0.296774840137206));
#67050=DIRECTION('center_axis',(1.,0.,0.));
#67051=DIRECTION('ref_axis',(0.,-0.64278760968654,-0.766044443118978));
#67052=DIRECTION('center_axis',(-1.,0.,0.));
#67053=DIRECTION('ref_axis',(0.,1.,0.));
#67054=DIRECTION('center_axis',(0.,-0.954947482462536,-0.296774840137206));
#67055=DIRECTION('ref_axis',(0.,0.296774840137206,-0.954947482462536));
#67056=DIRECTION('',(1.,0.,0.));
#67057=DIRECTION('',(0.,-0.296774840137206,0.954947482462536));
#67058=DIRECTION('',(1.,0.,0.));
#67059=DIRECTION('',(0.,0.296774840137206,-0.954947482462536));
#67060=DIRECTION('center_axis',(1.,0.,0.));
#67061=DIRECTION('ref_axis',(0.,-0.766044443118978,-0.642787609686539));
#67062=DIRECTION('center_axis',(1.,0.,0.));
#67063=DIRECTION('ref_axis',(0.,0.,-1.));
#67064=DIRECTION('',(0.,-0.888905274281375,0.458091053563321));
#67065=DIRECTION('center_axis',(0.,0.458091053563321,0.888905274281375));
#67066=DIRECTION('ref_axis',(0.,-0.888905274281375,0.458091053563321));
#67067=DIRECTION('',(-1.,0.,0.));
#67068=DIRECTION('',(0.,0.888905274281375,-0.458091053563321));
#67069=DIRECTION('center_axis',(1.,0.,0.));
#67070=DIRECTION('ref_axis',(0.,-0.766044443118978,-0.642787609686539));
#67071=DIRECTION('center_axis',(-1.,0.,0.));
#67072=DIRECTION('ref_axis',(0.,1.,0.));
#67073=DIRECTION('center_axis',(0.,-0.991974094615816,-0.126441273368837));
#67074=DIRECTION('ref_axis',(0.,0.126441273368837,-0.991974094615816));
#67075=DIRECTION('',(1.,0.,0.));
#67076=DIRECTION('',(0.,-0.126441273368837,0.991974094615816));
#67077=DIRECTION('',(1.,0.,0.));
#67078=DIRECTION('',(0.,0.126441273368837,-0.991974094615816));
#67079=DIRECTION('center_axis',(1.,0.,0.));
#67080=DIRECTION('ref_axis',(0.,-0.866025403784439,-0.5));
#67081=DIRECTION('center_axis',(1.,0.,0.));
#67082=DIRECTION('ref_axis',(0.,0.,-1.));
#67083=DIRECTION('',(0.,-0.795854129148946,0.605488402132173));
#67084=DIRECTION('center_axis',(0.,0.605488402132173,0.795854129148946));
#67085=DIRECTION('ref_axis',(0.,-0.795854129148946,0.605488402132173));
#67086=DIRECTION('',(-1.,0.,0.));
#67087=DIRECTION('',(0.,0.795854129148946,-0.605488402132173));
#67088=DIRECTION('center_axis',(1.,0.,0.));
#67089=DIRECTION('ref_axis',(0.,-0.866025403784439,-0.5));
#67090=DIRECTION('center_axis',(-1.,0.,0.));
#67091=DIRECTION('ref_axis',(0.,1.,0.));
#67092=DIRECTION('center_axis',(0.,-0.998860075867306,0.0477341475084739));
#67093=DIRECTION('ref_axis',(0.,-0.0477341475084739,-0.998860075867306));
#67094=DIRECTION('',(1.,0.,0.));
#67095=DIRECTION('',(0.,0.0477341475084739,0.998860075867306));
#67096=DIRECTION('',(1.,0.,0.));
#67097=DIRECTION('',(0.,-0.0477341475084739,-0.998860075867306));
#67098=DIRECTION('center_axis',(1.,0.,0.));
#67099=DIRECTION('ref_axis',(0.,-0.939692620785909,-0.342020143325668));
#67100=DIRECTION('center_axis',(1.,0.,0.));
#67101=DIRECTION('ref_axis',(0.,0.,-1.));
#67102=DIRECTION('',(0.,-0.678621359023948,0.734488291994154));
#67103=DIRECTION('center_axis',(0.,0.734488291994154,0.678621359023948));
#67104=DIRECTION('ref_axis',(0.,-0.678621359023948,0.734488291994154));
#67105=DIRECTION('',(-1.,0.,0.));
#67106=DIRECTION('',(0.,0.678621359023948,-0.734488291994154));
#67107=DIRECTION('center_axis',(1.,0.,0.));
#67108=DIRECTION('ref_axis',(0.,-0.939692620785909,-0.342020143325668));
#67109=DIRECTION('center_axis',(-1.,0.,0.));
#67110=DIRECTION('ref_axis',(0.,1.,0.));
#67111=DIRECTION('center_axis',(0.,-0.975396199161154,0.220459190468383));
#67112=DIRECTION('ref_axis',(0.,-0.220459190468383,-0.975396199161154));
#67113=DIRECTION('',(1.,0.,0.));
#67114=DIRECTION('',(0.,0.220459190468383,0.975396199161154));
#67115=DIRECTION('',(1.,0.,0.));
#67116=DIRECTION('',(0.,-0.220459190468383,-0.975396199161154));
#67117=DIRECTION('center_axis',(1.,0.,0.));
#67118=DIRECTION('ref_axis',(0.,-0.984807753012208,-0.17364817766693));
#67119=DIRECTION('center_axis',(1.,0.,0.));
#67120=DIRECTION('ref_axis',(0.,0.,-1.));
#67121=DIRECTION('',(0.,-0.540769022303984,0.841171126772902));
#67122=DIRECTION('center_axis',(0.,0.841171126772902,0.540769022303984));
#67123=DIRECTION('ref_axis',(0.,-0.540769022303984,0.841171126772902));
#67124=DIRECTION('',(-1.,0.,0.));
#67125=DIRECTION('',(0.,0.540769022303984,-0.841171126772902));
#67126=DIRECTION('center_axis',(1.,0.,0.));
#67127=DIRECTION('ref_axis',(0.,-0.984807753012208,-0.17364817766693));
#67128=DIRECTION('center_axis',(-1.,0.,0.));
#67129=DIRECTION('ref_axis',(0.,1.,0.));
#67130=DIRECTION('center_axis',(0.,-0.922295402517783,0.386485692483643));
#67131=DIRECTION('ref_axis',(0.,-0.386485692483643,-0.922295402517783));
#67132=DIRECTION('',(1.,0.,0.));
#67133=DIRECTION('',(0.,0.386485692483643,0.922295402517783));
#67134=DIRECTION('',(1.,0.,0.));
#67135=DIRECTION('',(0.,-0.386485692483643,-0.922295402517783));
#67136=DIRECTION('center_axis',(1.,0.,0.));
#67137=DIRECTION('ref_axis',(0.,-1.,1.83697019872103E-16));
#67138=DIRECTION('center_axis',(1.,0.,0.));
#67139=DIRECTION('ref_axis',(0.,0.,-1.));
#67140=DIRECTION('',(0.,-0.386485692483642,0.922295402517783));
#67141=DIRECTION('center_axis',(0.,0.922295402517783,0.386485692483642));
#67142=DIRECTION('ref_axis',(0.,-0.386485692483642,0.922295402517783));
#67143=DIRECTION('',(-1.,0.,0.));
#67144=DIRECTION('',(0.,0.386485692483642,-0.922295402517783));
#67145=DIRECTION('center_axis',(1.,0.,0.));
#67146=DIRECTION('ref_axis',(0.,-1.,1.83697019872103E-16));
#67147=DIRECTION('center_axis',(-1.,0.,0.));
#67148=DIRECTION('ref_axis',(0.,1.,0.));
#67149=DIRECTION('center_axis',(0.,-0.841171126772902,0.540769022303984));
#67150=DIRECTION('ref_axis',(0.,-0.540769022303984,-0.841171126772902));
#67151=DIRECTION('',(1.,0.,0.));
#67152=DIRECTION('',(0.,0.540769022303984,0.841171126772902));
#67153=DIRECTION('',(1.,0.,0.));
#67154=DIRECTION('',(0.,-0.540769022303984,-0.841171126772902));
#67155=DIRECTION('center_axis',(1.,0.,0.));
#67156=DIRECTION('ref_axis',(0.,-0.984807753012208,0.17364817766693));
#67157=DIRECTION('center_axis',(1.,0.,0.));
#67158=DIRECTION('ref_axis',(0.,0.,-1.));
#67159=DIRECTION('',(0.,-0.220459190468382,0.975396199161154));
#67160=DIRECTION('center_axis',(0.,0.975396199161154,0.220459190468382));
#67161=DIRECTION('ref_axis',(0.,-0.220459190468382,0.975396199161154));
#67162=DIRECTION('',(-1.,0.,0.));
#67163=DIRECTION('',(0.,0.220459190468382,-0.975396199161154));
#67164=DIRECTION('center_axis',(1.,0.,0.));
#67165=DIRECTION('ref_axis',(0.,-0.984807753012208,0.17364817766693));
#67166=DIRECTION('center_axis',(-1.,0.,0.));
#67167=DIRECTION('ref_axis',(0.,1.,0.));
#67168=DIRECTION('center_axis',(0.,-0.734488291994154,0.678621359023949));
#67169=DIRECTION('ref_axis',(0.,-0.678621359023949,-0.734488291994154));
#67170=DIRECTION('',(1.,0.,0.));
#67171=DIRECTION('',(0.,0.678621359023949,0.734488291994154));
#67172=DIRECTION('',(1.,0.,0.));
#67173=DIRECTION('',(0.,-0.678621359023949,-0.734488291994154));
#67174=DIRECTION('center_axis',(1.,0.,0.));
#67175=DIRECTION('ref_axis',(0.,-0.939692620785908,0.342020143325669));
#67176=DIRECTION('center_axis',(1.,0.,0.));
#67177=DIRECTION('ref_axis',(0.,0.,-1.));
#67178=DIRECTION('',(0.,-0.0477341475084726,0.998860075867306));
#67179=DIRECTION('center_axis',(0.,0.998860075867306,0.0477341475084726));
#67180=DIRECTION('ref_axis',(0.,-0.0477341475084726,0.998860075867306));
#67181=DIRECTION('',(-1.,0.,0.));
#67182=DIRECTION('',(0.,0.0477341475084726,-0.998860075867306));
#67183=DIRECTION('center_axis',(1.,0.,0.));
#67184=DIRECTION('ref_axis',(0.,-0.939692620785908,0.342020143325669));
#67185=DIRECTION('center_axis',(-1.,0.,0.));
#67186=DIRECTION('ref_axis',(0.,1.,0.));
#67187=DIRECTION('center_axis',(0.,-0.605488402132173,0.795854129148947));
#67188=DIRECTION('ref_axis',(0.,-0.795854129148947,-0.605488402132173));
#67189=DIRECTION('',(1.,0.,0.));
#67190=DIRECTION('',(0.,0.795854129148947,0.605488402132173));
#67191=DIRECTION('',(1.,0.,0.));
#67192=DIRECTION('',(0.,-0.795854129148947,-0.605488402132173));
#67193=DIRECTION('center_axis',(1.,0.,0.));
#67194=DIRECTION('ref_axis',(0.,-0.866025403784438,0.5));
#67195=DIRECTION('center_axis',(1.,0.,0.));
#67196=DIRECTION('ref_axis',(0.,0.,-1.));
#67197=DIRECTION('',(0.,0.126441273368837,0.991974094615816));
#67198=DIRECTION('center_axis',(0.,0.991974094615816,-0.126441273368837));
#67199=DIRECTION('ref_axis',(0.,0.126441273368837,0.991974094615816));
#67200=DIRECTION('',(-1.,0.,0.));
#67201=DIRECTION('',(0.,-0.126441273368837,-0.991974094615816));
#67202=DIRECTION('center_axis',(1.,0.,0.));
#67203=DIRECTION('ref_axis',(0.,-0.866025403784438,0.5));
#67204=DIRECTION('center_axis',(-1.,0.,0.));
#67205=DIRECTION('ref_axis',(0.,1.,0.));
#67206=DIRECTION('center_axis',(0.,-0.458091053563321,0.888905274281375));
#67207=DIRECTION('ref_axis',(0.,-0.888905274281375,-0.458091053563321));
#67208=DIRECTION('',(1.,0.,0.));
#67209=DIRECTION('',(0.,0.888905274281375,0.458091053563321));
#67210=DIRECTION('',(1.,0.,0.));
#67211=DIRECTION('',(0.,-0.888905274281375,-0.458091053563321));
#67212=DIRECTION('center_axis',(1.,0.,0.));
#67213=DIRECTION('ref_axis',(0.,-0.766044443118978,0.642787609686539));
#67214=DIRECTION('center_axis',(1.,0.,0.));
#67215=DIRECTION('ref_axis',(0.,0.,-1.));
#67216=DIRECTION('',(0.,0.296774840137206,0.954947482462536));
#67217=DIRECTION('center_axis',(0.,0.954947482462536,-0.296774840137206));
#67218=DIRECTION('ref_axis',(0.,0.296774840137206,0.954947482462536));
#67219=DIRECTION('',(-1.,0.,0.));
#67220=DIRECTION('',(0.,-0.296774840137206,-0.954947482462536));
#67221=DIRECTION('center_axis',(1.,0.,0.));
#67222=DIRECTION('ref_axis',(0.,-0.766044443118978,0.642787609686539));
#67223=DIRECTION('center_axis',(-1.,0.,0.));
#67224=DIRECTION('ref_axis',(0.,1.,0.));
#67225=DIRECTION('center_axis',(0.,-0.296774840137206,0.954947482462536));
#67226=DIRECTION('ref_axis',(0.,-0.954947482462536,-0.296774840137206));
#67227=DIRECTION('',(1.,0.,0.));
#67228=DIRECTION('',(0.,0.954947482462536,0.296774840137206));
#67229=DIRECTION('',(1.,0.,0.));
#67230=DIRECTION('',(0.,-0.954947482462536,-0.296774840137206));
#67231=DIRECTION('center_axis',(1.,0.,0.));
#67232=DIRECTION('ref_axis',(0.,-0.642787609686539,0.766044443118978));
#67233=DIRECTION('center_axis',(1.,0.,0.));
#67234=DIRECTION('ref_axis',(0.,0.,-1.));
#67235=DIRECTION('',(0.,0.458091053563321,0.888905274281375));
#67236=DIRECTION('center_axis',(0.,0.888905274281375,-0.458091053563321));
#67237=DIRECTION('ref_axis',(0.,0.458091053563321,0.888905274281375));
#67238=DIRECTION('',(-1.,0.,0.));
#67239=DIRECTION('',(0.,-0.458091053563321,-0.888905274281375));
#67240=DIRECTION('center_axis',(1.,0.,0.));
#67241=DIRECTION('ref_axis',(0.,-0.642787609686539,0.766044443118978));
#67242=DIRECTION('center_axis',(-1.,0.,0.));
#67243=DIRECTION('ref_axis',(0.,1.,0.));
#67244=DIRECTION('center_axis',(0.,-0.126441273368836,0.991974094615816));
#67245=DIRECTION('ref_axis',(0.,-0.991974094615816,-0.126441273368836));
#67246=DIRECTION('',(1.,0.,0.));
#67247=DIRECTION('',(0.,0.991974094615816,0.126441273368836));
#67248=DIRECTION('',(1.,0.,0.));
#67249=DIRECTION('',(0.,-0.991974094615816,-0.126441273368836));
#67250=DIRECTION('center_axis',(1.,0.,0.));
#67251=DIRECTION('ref_axis',(0.,-0.5,0.866025403784439));
#67252=DIRECTION('center_axis',(1.,0.,0.));
#67253=DIRECTION('ref_axis',(0.,0.,-1.));
#67254=DIRECTION('',(0.,0.605488402132173,0.795854129148946));
#67255=DIRECTION('center_axis',(0.,0.795854129148946,-0.605488402132173));
#67256=DIRECTION('ref_axis',(0.,0.605488402132173,0.795854129148946));
#67257=DIRECTION('',(-1.,0.,0.));
#67258=DIRECTION('',(0.,-0.605488402132173,-0.795854129148946));
#67259=DIRECTION('center_axis',(1.,0.,0.));
#67260=DIRECTION('ref_axis',(0.,-0.5,0.866025403784439));
#67261=DIRECTION('center_axis',(-1.,0.,0.));
#67262=DIRECTION('ref_axis',(0.,1.,0.));
#67263=DIRECTION('center_axis',(0.,0.0477341475084734,0.998860075867306));
#67264=DIRECTION('ref_axis',(0.,-0.998860075867306,0.0477341475084734));
#67265=DIRECTION('',(1.,0.,0.));
#67266=DIRECTION('',(0.,0.998860075867306,-0.0477341475084734));
#67267=DIRECTION('',(1.,0.,0.));
#67268=DIRECTION('',(0.,-0.998860075867306,0.0477341475084734));
#67269=DIRECTION('center_axis',(1.,0.,0.));
#67270=DIRECTION('ref_axis',(0.,-0.342020143325669,0.939692620785909));
#67271=DIRECTION('center_axis',(1.,0.,0.));
#67272=DIRECTION('ref_axis',(0.,0.,-1.));
#67273=DIRECTION('',(0.,0.734488291994154,0.678621359023948));
#67274=DIRECTION('center_axis',(0.,0.678621359023948,-0.734488291994154));
#67275=DIRECTION('ref_axis',(0.,0.734488291994154,0.678621359023948));
#67276=DIRECTION('',(-1.,0.,0.));
#67277=DIRECTION('',(0.,-0.734488291994154,-0.678621359023948));
#67278=DIRECTION('center_axis',(1.,0.,0.));
#67279=DIRECTION('ref_axis',(0.,-0.342020143325669,0.939692620785909));
#67280=DIRECTION('center_axis',(-1.,0.,0.));
#67281=DIRECTION('ref_axis',(0.,1.,0.));
#67282=DIRECTION('center_axis',(0.,0.220459190468383,0.975396199161154));
#67283=DIRECTION('ref_axis',(0.,-0.975396199161154,0.220459190468383));
#67284=DIRECTION('',(1.,0.,0.));
#67285=DIRECTION('',(0.,0.975396199161154,-0.220459190468383));
#67286=DIRECTION('',(1.,0.,0.));
#67287=DIRECTION('',(0.,-0.975396199161154,0.220459190468383));
#67288=DIRECTION('center_axis',(1.,0.,0.));
#67289=DIRECTION('ref_axis',(0.,-0.17364817766693,0.984807753012208));
#67290=DIRECTION('center_axis',(1.,0.,0.));
#67291=DIRECTION('ref_axis',(0.,0.,-1.));
#67292=DIRECTION('',(0.,0.841171126772902,0.540769022303984));
#67293=DIRECTION('center_axis',(0.,0.540769022303984,-0.841171126772902));
#67294=DIRECTION('ref_axis',(0.,0.841171126772902,0.540769022303984));
#67295=DIRECTION('',(-1.,0.,0.));
#67296=DIRECTION('',(0.,-0.841171126772902,-0.540769022303984));
#67297=DIRECTION('center_axis',(1.,0.,0.));
#67298=DIRECTION('ref_axis',(0.,-0.17364817766693,0.984807753012208));
#67299=DIRECTION('center_axis',(-1.,0.,0.));
#67300=DIRECTION('ref_axis',(0.,1.,0.));
#67301=DIRECTION('center_axis',(0.,0.386485692483643,0.922295402517783));
#67302=DIRECTION('ref_axis',(0.,-0.922295402517783,0.386485692483643));
#67303=DIRECTION('',(1.,0.,0.));
#67304=DIRECTION('',(0.,0.922295402517783,-0.386485692483643));
#67305=DIRECTION('',(1.,0.,0.));
#67306=DIRECTION('',(0.,-0.922295402517783,0.386485692483643));
#67307=DIRECTION('center_axis',(1.,0.,0.));
#67308=DIRECTION('ref_axis',(0.,1.22464679914735E-16,1.));
#67309=DIRECTION('center_axis',(1.,0.,0.));
#67310=DIRECTION('ref_axis',(0.,0.,-1.));
#67311=DIRECTION('',(0.,0.922295402517783,0.386485692483642));
#67312=DIRECTION('center_axis',(1.,0.,0.));
#67313=DIRECTION('ref_axis',(0.,0.,-1.));
#67314=DIRECTION('center_axis',(0.,0.386485692483643,-0.922295402517783));
#67315=DIRECTION('ref_axis',(0.,0.922295402517783,0.386485692483642));
#67316=DIRECTION('',(-1.,0.,0.));
#67317=DIRECTION('',(0.,-0.922295402517783,-0.386485692483642));
#67318=DIRECTION('center_axis',(1.,0.,0.));
#67319=DIRECTION('ref_axis',(0.,1.22464679914735E-16,1.));
#67320=DIRECTION('center_axis',(-1.,0.,0.));
#67321=DIRECTION('ref_axis',(0.,1.,0.));
#67322=DIRECTION('center_axis',(-1.,0.,0.));
#67323=DIRECTION('ref_axis',(0.,1.,0.));
#67324=DIRECTION('center_axis',(0.,0.540769022303985,0.841171126772901));
#67325=DIRECTION('ref_axis',(0.,-0.841171126772902,0.540769022303985));
#67326=DIRECTION('',(1.,0.,0.));
#67327=DIRECTION('',(0.,0.841171126772902,-0.540769022303985));
#67328=DIRECTION('',(1.,0.,0.));
#67329=DIRECTION('',(0.,-0.841171126772902,0.540769022303985));
#67330=DIRECTION('center_axis',(1.,0.,0.));
#67331=DIRECTION('ref_axis',(0.,0.173648177666931,0.984807753012208));
#67332=DIRECTION('center_axis',(1.,0.,0.));
#67333=DIRECTION('ref_axis',(0.,0.,-1.));
#67334=DIRECTION('',(0.,0.975396199161154,0.220459190468382));
#67335=DIRECTION('center_axis',(0.,0.220459190468382,-0.975396199161154));
#67336=DIRECTION('ref_axis',(0.,0.975396199161154,0.220459190468382));
#67337=DIRECTION('',(-1.,0.,0.));
#67338=DIRECTION('',(0.,-0.975396199161154,-0.220459190468382));
#67339=DIRECTION('center_axis',(1.,0.,0.));
#67340=DIRECTION('ref_axis',(0.,0.173648177666931,0.984807753012208));
#67341=DIRECTION('center_axis',(-1.,0.,0.));
#67342=DIRECTION('ref_axis',(0.,1.,0.));
#67343=DIRECTION('center_axis',(0.,0.678621359023948,0.734488291994154));
#67344=DIRECTION('ref_axis',(0.,-0.734488291994154,0.678621359023948));
#67345=DIRECTION('',(1.,0.,0.));
#67346=DIRECTION('',(0.,0.734488291994154,-0.678621359023948));
#67347=DIRECTION('',(1.,0.,0.));
#67348=DIRECTION('',(0.,-0.734488291994154,0.678621359023948));
#67349=DIRECTION('center_axis',(1.,0.,0.));
#67350=DIRECTION('ref_axis',(0.,0.342020143325669,0.939692620785908));
#67351=DIRECTION('center_axis',(1.,0.,0.));
#67352=DIRECTION('ref_axis',(0.,0.,-1.));
#67353=DIRECTION('',(0.,0.998860075867306,0.0477341475084732));
#67354=DIRECTION('center_axis',(0.,0.0477341475084731,-0.998860075867306));
#67355=DIRECTION('ref_axis',(0.,0.998860075867306,0.0477341475084732));
#67356=DIRECTION('',(-1.,0.,0.));
#67357=DIRECTION('',(0.,-0.998860075867306,-0.0477341475084732));
#67358=DIRECTION('center_axis',(1.,0.,0.));
#67359=DIRECTION('ref_axis',(0.,0.342020143325669,0.939692620785908));
#67360=DIRECTION('center_axis',(-1.,0.,0.));
#67361=DIRECTION('ref_axis',(0.,1.,0.));
#67362=DIRECTION('center_axis',(0.,0.795854129148946,0.605488402132173));
#67363=DIRECTION('ref_axis',(0.,-0.605488402132173,0.795854129148946));
#67364=DIRECTION('',(1.,0.,0.));
#67365=DIRECTION('',(0.,0.605488402132173,-0.795854129148946));
#67366=DIRECTION('',(1.,0.,0.));
#67367=DIRECTION('',(0.,-0.605488402132173,0.795854129148946));
#67368=DIRECTION('center_axis',(1.,0.,0.));
#67369=DIRECTION('ref_axis',(0.,0.5,0.866025403784439));
#67370=DIRECTION('center_axis',(1.,0.,0.));
#67371=DIRECTION('ref_axis',(0.,0.,-1.));
#67372=DIRECTION('',(0.,0.991974094615816,-0.126441273368836));
#67373=DIRECTION('center_axis',(0.,-0.126441273368836,-0.991974094615816));
#67374=DIRECTION('ref_axis',(0.,0.991974094615816,-0.126441273368836));
#67375=DIRECTION('',(-1.,0.,0.));
#67376=DIRECTION('',(0.,-0.991974094615816,0.126441273368836));
#67377=DIRECTION('center_axis',(1.,0.,0.));
#67378=DIRECTION('ref_axis',(0.,0.5,0.866025403784439));
#67379=DIRECTION('center_axis',(-1.,0.,0.));
#67380=DIRECTION('ref_axis',(0.,1.,0.));
#67381=DIRECTION('center_axis',(0.,0.888905274281375,0.458091053563321));
#67382=DIRECTION('ref_axis',(0.,-0.458091053563321,0.888905274281375));
#67383=DIRECTION('',(1.,0.,0.));
#67384=DIRECTION('',(0.,0.458091053563321,-0.888905274281375));
#67385=DIRECTION('',(1.,0.,0.));
#67386=DIRECTION('',(0.,-0.458091053563321,0.888905274281375));
#67387=DIRECTION('center_axis',(1.,0.,0.));
#67388=DIRECTION('ref_axis',(0.,0.642787609686539,0.766044443118978));
#67389=DIRECTION('center_axis',(1.,0.,0.));
#67390=DIRECTION('ref_axis',(0.,0.,-1.));
#67391=DIRECTION('',(0.,0.954947482462536,-0.296774840137206));
#67392=DIRECTION('center_axis',(0.,-0.296774840137206,-0.954947482462536));
#67393=DIRECTION('ref_axis',(0.,0.954947482462536,-0.296774840137206));
#67394=DIRECTION('',(-1.,0.,0.));
#67395=DIRECTION('',(0.,-0.954947482462536,0.296774840137206));
#67396=DIRECTION('center_axis',(1.,0.,0.));
#67397=DIRECTION('ref_axis',(0.,0.642787609686539,0.766044443118978));
#67398=DIRECTION('center_axis',(-1.,0.,0.));
#67399=DIRECTION('ref_axis',(0.,1.,0.));
#67400=DIRECTION('center_axis',(0.,0.954947482462536,0.296774840137206));
#67401=DIRECTION('ref_axis',(0.,-0.296774840137206,0.954947482462536));
#67402=DIRECTION('',(1.,0.,0.));
#67403=DIRECTION('',(0.,0.296774840137206,-0.954947482462536));
#67404=DIRECTION('',(1.,0.,0.));
#67405=DIRECTION('',(0.,-0.296774840137206,0.954947482462536));
#67406=DIRECTION('center_axis',(1.,0.,0.));
#67407=DIRECTION('ref_axis',(0.,0.766044443118978,0.642787609686539));
#67408=DIRECTION('center_axis',(1.,0.,0.));
#67409=DIRECTION('ref_axis',(0.,0.,-1.));
#67410=DIRECTION('',(0.,0.888905274281375,-0.458091053563321));
#67411=DIRECTION('center_axis',(0.,-0.458091053563321,-0.888905274281375));
#67412=DIRECTION('ref_axis',(0.,0.888905274281375,-0.458091053563321));
#67413=DIRECTION('',(-1.,0.,0.));
#67414=DIRECTION('',(0.,-0.888905274281375,0.458091053563321));
#67415=DIRECTION('center_axis',(1.,0.,0.));
#67416=DIRECTION('ref_axis',(0.,0.766044443118978,0.642787609686539));
#67417=DIRECTION('center_axis',(-1.,0.,0.));
#67418=DIRECTION('ref_axis',(0.,1.,0.));
#67419=DIRECTION('center_axis',(0.,0.991974094615816,0.126441273368836));
#67420=DIRECTION('ref_axis',(0.,-0.126441273368836,0.991974094615816));
#67421=DIRECTION('',(1.,0.,0.));
#67422=DIRECTION('',(0.,0.126441273368836,-0.991974094615816));
#67423=DIRECTION('',(1.,0.,0.));
#67424=DIRECTION('',(0.,-0.126441273368836,0.991974094615816));
#67425=DIRECTION('center_axis',(1.,0.,0.));
#67426=DIRECTION('ref_axis',(0.,0.866025403784439,0.5));
#67427=DIRECTION('center_axis',(1.,0.,0.));
#67428=DIRECTION('ref_axis',(0.,0.,-1.));
#67429=DIRECTION('',(0.,0.795854129148946,-0.605488402132173));
#67430=DIRECTION('center_axis',(0.,-0.605488402132173,-0.795854129148946));
#67431=DIRECTION('ref_axis',(0.,0.795854129148946,-0.605488402132173));
#67432=DIRECTION('',(-1.,0.,0.));
#67433=DIRECTION('',(0.,-0.795854129148946,0.605488402132173));
#67434=DIRECTION('center_axis',(1.,0.,0.));
#67435=DIRECTION('ref_axis',(0.,0.866025403784439,0.5));
#67436=DIRECTION('center_axis',(-1.,0.,0.));
#67437=DIRECTION('ref_axis',(0.,1.,0.));
#67438=DIRECTION('center_axis',(0.,0.998860075867306,-0.0477341475084733));
#67439=DIRECTION('ref_axis',(0.,0.0477341475084733,0.998860075867306));
#67440=DIRECTION('',(1.,0.,0.));
#67441=DIRECTION('',(0.,-0.0477341475084733,-0.998860075867306));
#67442=DIRECTION('',(1.,0.,0.));
#67443=DIRECTION('',(0.,0.0477341475084733,0.998860075867306));
#67444=DIRECTION('center_axis',(1.,0.,0.));
#67445=DIRECTION('ref_axis',(0.,0.939692620785908,0.342020143325669));
#67446=DIRECTION('center_axis',(1.,0.,0.));
#67447=DIRECTION('ref_axis',(0.,0.,-1.));
#67448=DIRECTION('',(0.,0.678621359023948,-0.734488291994154));
#67449=DIRECTION('center_axis',(0.,-0.734488291994154,-0.678621359023948));
#67450=DIRECTION('ref_axis',(0.,0.678621359023948,-0.734488291994154));
#67451=DIRECTION('',(-1.,0.,0.));
#67452=DIRECTION('',(0.,-0.678621359023948,0.734488291994154));
#67453=DIRECTION('center_axis',(1.,0.,0.));
#67454=DIRECTION('ref_axis',(0.,0.939692620785908,0.342020143325669));
#67455=DIRECTION('center_axis',(-1.,0.,0.));
#67456=DIRECTION('ref_axis',(0.,1.,0.));
#67457=DIRECTION('center_axis',(0.,0.975396199161154,-0.220459190468382));
#67458=DIRECTION('ref_axis',(0.,0.220459190468382,0.975396199161154));
#67459=DIRECTION('',(1.,0.,0.));
#67460=DIRECTION('',(0.,-0.220459190468382,-0.975396199161154));
#67461=DIRECTION('',(1.,0.,0.));
#67462=DIRECTION('',(0.,0.220459190468382,0.975396199161154));
#67463=DIRECTION('center_axis',(1.,0.,0.));
#67464=DIRECTION('ref_axis',(0.,0.984807753012208,0.17364817766693));
#67465=DIRECTION('center_axis',(1.,0.,0.));
#67466=DIRECTION('ref_axis',(0.,0.,-1.));
#67467=DIRECTION('',(0.,0.540769022303984,-0.841171126772902));
#67468=DIRECTION('center_axis',(0.,-0.841171126772902,-0.540769022303984));
#67469=DIRECTION('ref_axis',(0.,0.540769022303984,-0.841171126772902));
#67470=DIRECTION('',(-1.,0.,0.));
#67471=DIRECTION('',(0.,-0.540769022303984,0.841171126772902));
#67472=DIRECTION('center_axis',(1.,0.,0.));
#67473=DIRECTION('ref_axis',(0.,0.984807753012208,0.17364817766693));
#67474=DIRECTION('center_axis',(-1.,0.,0.));
#67475=DIRECTION('ref_axis',(0.,1.,0.));
#67476=DIRECTION('center_axis',(0.,0.922295402517783,-0.386485692483643));
#67477=DIRECTION('ref_axis',(0.,0.386485692483643,0.922295402517783));
#67478=DIRECTION('',(1.,0.,0.));
#67479=DIRECTION('',(0.,-0.386485692483643,-0.922295402517783));
#67480=DIRECTION('',(1.,0.,0.));
#67481=DIRECTION('',(0.,0.386485692483643,0.922295402517783));
#67482=DIRECTION('center_axis',(1.,0.,0.));
#67483=DIRECTION('ref_axis',(0.,1.,-6.12323399573677E-17));
#67484=DIRECTION('center_axis',(1.,0.,0.));
#67485=DIRECTION('ref_axis',(0.,0.,-1.));
#67486=DIRECTION('',(0.,0.386485692483643,-0.922295402517783));
#67487=DIRECTION('center_axis',(0.,-0.922295402517783,-0.386485692483643));
#67488=DIRECTION('ref_axis',(0.,0.386485692483643,-0.922295402517783));
#67489=DIRECTION('',(-1.,0.,0.));
#67490=DIRECTION('',(0.,-0.386485692483643,0.922295402517783));
#67491=DIRECTION('center_axis',(1.,0.,0.));
#67492=DIRECTION('ref_axis',(0.,1.,-6.12323399573677E-17));
#67493=DIRECTION('center_axis',(-1.,0.,0.));
#67494=DIRECTION('ref_axis',(0.,1.,0.));
#67495=DIRECTION('center_axis',(0.,0.841171126772902,-0.540769022303984));
#67496=DIRECTION('ref_axis',(0.,0.540769022303984,0.841171126772902));
#67497=DIRECTION('',(1.,0.,0.));
#67498=DIRECTION('',(0.,-0.540769022303984,-0.841171126772902));
#67499=DIRECTION('',(1.,0.,0.));
#67500=DIRECTION('',(0.,0.540769022303984,0.841171126772902));
#67501=DIRECTION('center_axis',(1.,0.,0.));
#67502=DIRECTION('ref_axis',(0.,0.984807753012208,-0.17364817766693));
#67503=DIRECTION('center_axis',(1.,0.,0.));
#67504=DIRECTION('ref_axis',(0.,0.,-1.));
#67505=DIRECTION('',(0.,0.220459190468382,-0.975396199161154));
#67506=DIRECTION('center_axis',(0.,-0.975396199161154,-0.220459190468382));
#67507=DIRECTION('ref_axis',(0.,0.220459190468382,-0.975396199161154));
#67508=DIRECTION('',(-1.,0.,0.));
#67509=DIRECTION('',(0.,-0.220459190468382,0.975396199161154));
#67510=DIRECTION('center_axis',(1.,0.,0.));
#67511=DIRECTION('ref_axis',(0.,0.984807753012208,-0.17364817766693));
#67512=DIRECTION('center_axis',(-1.,0.,0.));
#67513=DIRECTION('ref_axis',(0.,1.,0.));
#67514=DIRECTION('center_axis',(0.,0.734488291994154,-0.678621359023948));
#67515=DIRECTION('ref_axis',(0.,0.678621359023948,0.734488291994154));
#67516=DIRECTION('',(1.,0.,0.));
#67517=DIRECTION('',(0.,-0.678621359023948,-0.734488291994154));
#67518=DIRECTION('',(1.,0.,0.));
#67519=DIRECTION('',(0.,0.678621359023948,0.734488291994154));
#67520=DIRECTION('center_axis',(1.,0.,0.));
#67521=DIRECTION('ref_axis',(0.,0.939692620785908,-0.342020143325669));
#67522=DIRECTION('center_axis',(1.,0.,0.));
#67523=DIRECTION('ref_axis',(0.,0.,-1.));
#67524=DIRECTION('',(0.,0.0477341475084732,-0.998860075867306));
#67525=DIRECTION('center_axis',(0.,-0.998860075867306,-0.0477341475084731));
#67526=DIRECTION('ref_axis',(0.,0.0477341475084732,-0.998860075867306));
#67527=DIRECTION('',(-1.,0.,0.));
#67528=DIRECTION('',(0.,-0.0477341475084732,0.998860075867306));
#67529=DIRECTION('center_axis',(1.,0.,0.));
#67530=DIRECTION('ref_axis',(0.,0.939692620785908,-0.342020143325669));
#67531=DIRECTION('center_axis',(-1.,0.,0.));
#67532=DIRECTION('ref_axis',(0.,1.,0.));
#67533=DIRECTION('center_axis',(0.,0.605488402132173,-0.795854129148946));
#67534=DIRECTION('ref_axis',(0.,0.795854129148946,0.605488402132173));
#67535=DIRECTION('',(1.,0.,0.));
#67536=DIRECTION('',(0.,-0.795854129148946,-0.605488402132173));
#67537=DIRECTION('',(1.,0.,0.));
#67538=DIRECTION('',(0.,0.795854129148946,0.605488402132173));
#67539=DIRECTION('center_axis',(1.,0.,0.));
#67540=DIRECTION('ref_axis',(0.,0.866025403784439,-0.5));
#67541=DIRECTION('center_axis',(1.,0.,0.));
#67542=DIRECTION('ref_axis',(0.,0.,-1.));
#67543=DIRECTION('',(0.,-0.126441273368837,-0.991974094615816));
#67544=DIRECTION('center_axis',(0.,-0.991974094615816,0.126441273368837));
#67545=DIRECTION('ref_axis',(0.,-0.126441273368837,-0.991974094615816));
#67546=DIRECTION('',(-1.,0.,0.));
#67547=DIRECTION('',(0.,0.126441273368837,0.991974094615816));
#67548=DIRECTION('center_axis',(1.,0.,0.));
#67549=DIRECTION('ref_axis',(0.,0.866025403784439,-0.5));
#67550=DIRECTION('center_axis',(-1.,0.,0.));
#67551=DIRECTION('ref_axis',(0.,1.,0.));
#67552=DIRECTION('center_axis',(0.,0.458091053563321,-0.888905274281375));
#67553=DIRECTION('ref_axis',(0.,0.888905274281375,0.458091053563321));
#67554=DIRECTION('',(1.,0.,0.));
#67555=DIRECTION('',(0.,-0.888905274281375,-0.458091053563321));
#67556=DIRECTION('',(1.,0.,0.));
#67557=DIRECTION('',(0.,0.888905274281375,0.458091053563321));
#67558=DIRECTION('center_axis',(1.,0.,0.));
#67559=DIRECTION('ref_axis',(0.,0.766044443118978,-0.642787609686539));
#67560=DIRECTION('center_axis',(1.,0.,0.));
#67561=DIRECTION('ref_axis',(0.,0.,-1.));
#67562=DIRECTION('',(0.,-0.296774840137206,-0.954947482462536));
#67563=DIRECTION('center_axis',(0.,-0.954947482462536,0.296774840137206));
#67564=DIRECTION('ref_axis',(0.,-0.296774840137206,-0.954947482462536));
#67565=DIRECTION('',(-1.,0.,0.));
#67566=DIRECTION('',(0.,0.296774840137206,0.954947482462536));
#67567=DIRECTION('center_axis',(1.,0.,0.));
#67568=DIRECTION('ref_axis',(0.,0.766044443118978,-0.642787609686539));
#67569=DIRECTION('center_axis',(-1.,0.,0.));
#67570=DIRECTION('ref_axis',(0.,1.,0.));
#67571=DIRECTION('center_axis',(0.,0.296774840137206,-0.954947482462536));
#67572=DIRECTION('ref_axis',(0.,0.954947482462536,0.296774840137206));
#67573=DIRECTION('',(1.,0.,0.));
#67574=DIRECTION('',(0.,-0.954947482462536,-0.296774840137206));
#67575=DIRECTION('',(1.,0.,0.));
#67576=DIRECTION('',(0.,0.954947482462536,0.296774840137206));
#67577=DIRECTION('center_axis',(1.,0.,0.));
#67578=DIRECTION('ref_axis',(0.,0.642787609686539,-0.766044443118978));
#67579=DIRECTION('center_axis',(1.,0.,0.));
#67580=DIRECTION('ref_axis',(0.,0.,-1.));
#67581=DIRECTION('',(0.,-0.458091053563321,-0.888905274281375));
#67582=DIRECTION('center_axis',(0.,-0.888905274281375,0.458091053563321));
#67583=DIRECTION('ref_axis',(0.,-0.458091053563321,-0.888905274281375));
#67584=DIRECTION('',(-1.,0.,0.));
#67585=DIRECTION('',(0.,0.458091053563321,0.888905274281375));
#67586=DIRECTION('center_axis',(1.,0.,0.));
#67587=DIRECTION('ref_axis',(0.,0.642787609686539,-0.766044443118978));
#67588=DIRECTION('center_axis',(-1.,0.,0.));
#67589=DIRECTION('ref_axis',(0.,1.,0.));
#67590=DIRECTION('center_axis',(0.,0.126441273368836,-0.991974094615816));
#67591=DIRECTION('ref_axis',(0.,0.991974094615816,0.126441273368836));
#67592=DIRECTION('',(1.,0.,0.));
#67593=DIRECTION('',(0.,-0.991974094615816,-0.126441273368836));
#67594=DIRECTION('',(1.,0.,0.));
#67595=DIRECTION('',(0.,0.991974094615816,0.126441273368836));
#67596=DIRECTION('center_axis',(1.,0.,0.));
#67597=DIRECTION('ref_axis',(0.,0.5,-0.866025403784439));
#67598=DIRECTION('center_axis',(1.,0.,0.));
#67599=DIRECTION('ref_axis',(0.,0.,-1.));
#67600=DIRECTION('',(0.,-0.605488402132173,-0.795854129148946));
#67601=DIRECTION('center_axis',(0.,-0.795854129148946,0.605488402132173));
#67602=DIRECTION('ref_axis',(0.,-0.605488402132173,-0.795854129148946));
#67603=DIRECTION('',(-1.,0.,0.));
#67604=DIRECTION('',(0.,0.605488402132173,0.795854129148946));
#67605=DIRECTION('center_axis',(1.,0.,0.));
#67606=DIRECTION('ref_axis',(0.,0.5,-0.866025403784439));
#67607=DIRECTION('center_axis',(-1.,0.,0.));
#67608=DIRECTION('ref_axis',(0.,1.,0.));
#67609=DIRECTION('center_axis',(0.,-0.0477341475084733,-0.998860075867306));
#67610=DIRECTION('ref_axis',(0.,0.998860075867306,-0.0477341475084733));
#67611=DIRECTION('',(1.,0.,0.));
#67612=DIRECTION('',(0.,-0.998860075867306,0.0477341475084733));
#67613=DIRECTION('',(1.,0.,0.));
#67614=DIRECTION('',(0.,0.998860075867306,-0.0477341475084733));
#67615=DIRECTION('center_axis',(1.,0.,0.));
#67616=DIRECTION('ref_axis',(0.,0.342020143325669,-0.939692620785908));
#67617=DIRECTION('center_axis',(1.,0.,0.));
#67618=DIRECTION('ref_axis',(0.,0.,-1.));
#67619=DIRECTION('',(0.,-0.734488291994154,-0.678621359023948));
#67620=DIRECTION('center_axis',(0.,-0.678621359023948,0.734488291994154));
#67621=DIRECTION('ref_axis',(0.,-0.734488291994154,-0.678621359023948));
#67622=DIRECTION('',(-1.,0.,0.));
#67623=DIRECTION('',(0.,0.734488291994154,0.678621359023948));
#67624=DIRECTION('center_axis',(1.,0.,0.));
#67625=DIRECTION('ref_axis',(0.,0.342020143325669,-0.939692620785908));
#67626=DIRECTION('center_axis',(-1.,0.,0.));
#67627=DIRECTION('ref_axis',(0.,1.,0.));
#67628=DIRECTION('center_axis',(0.,-0.220459190468382,-0.975396199161154));
#67629=DIRECTION('ref_axis',(0.,0.975396199161154,-0.220459190468382));
#67630=DIRECTION('',(1.,0.,0.));
#67631=DIRECTION('',(0.,-0.975396199161154,0.220459190468382));
#67632=DIRECTION('',(1.,0.,0.));
#67633=DIRECTION('',(0.,0.975396199161154,-0.220459190468382));
#67634=DIRECTION('center_axis',(1.,0.,0.));
#67635=DIRECTION('ref_axis',(0.,0.17364817766693,-0.984807753012208));
#67636=DIRECTION('center_axis',(1.,0.,0.));
#67637=DIRECTION('ref_axis',(0.,0.,-1.));
#67638=DIRECTION('',(0.,-0.841171126772902,-0.540769022303984));
#67639=DIRECTION('center_axis',(0.,-0.540769022303984,0.841171126772902));
#67640=DIRECTION('ref_axis',(0.,-0.841171126772902,-0.540769022303984));
#67641=DIRECTION('',(-1.,0.,0.));
#67642=DIRECTION('',(0.,0.841171126772902,0.540769022303984));
#67643=DIRECTION('center_axis',(1.,0.,0.));
#67644=DIRECTION('ref_axis',(0.,0.17364817766693,-0.984807753012208));
#67645=DIRECTION('center_axis',(-1.,0.,0.));
#67646=DIRECTION('ref_axis',(0.,1.,0.));
#67647=DIRECTION('center_axis',(1.,0.,0.));
#67648=DIRECTION('ref_axis',(0.,0.,-1.));
#67649=DIRECTION('center_axis',(1.,0.,0.));
#67650=DIRECTION('ref_axis',(0.,0.,-1.));
#67651=DIRECTION('',(0.,0.922295402517783,-0.386485692483643));
#67652=DIRECTION('',(0.,-0.922295402517783,-0.386485692483643));
#67653=DIRECTION('center_axis',(0.,-0.386485692483643,-0.922295402517783));
#67654=DIRECTION('ref_axis',(0.,0.922295402517783,-0.386485692483643));
#67655=DIRECTION('',(1.,0.,0.));
#67656=DIRECTION('',(0.,-0.922295402517783,0.386485692483643));
#67657=DIRECTION('',(1.,0.,0.));
#67658=DIRECTION('center_axis',(0.,-0.386485692483643,0.922295402517783));
#67659=DIRECTION('ref_axis',(0.,-0.922295402517783,-0.386485692483643));
#67660=DIRECTION('',(-1.,0.,0.));
#67661=DIRECTION('',(0.,0.922295402517783,0.386485692483643));
#67662=DIRECTION('center_axis',(1.,0.,0.));
#67663=DIRECTION('ref_axis',(0.,0.,-1.));
#67664=DIRECTION('center_axis',(-1.,0.,0.));
#67665=DIRECTION('ref_axis',(0.,1.,0.));
#67666=DIRECTION('center_axis',(1.,0.,0.));
#67667=DIRECTION('ref_axis',(0.,1.,0.));
#67668=DIRECTION('',(0.517550572850554,-0.855652619082103,-1.04787224114095E-16));
#67669=DIRECTION('center_axis',(-1.,0.,0.));
#67670=DIRECTION('ref_axis',(0.,1.,0.));
#67671=DIRECTION('center_axis',(0.,-0.5,0.866025403784439));
#67672=DIRECTION('ref_axis',(0.,-0.866025403784439,-0.5));
#67673=DIRECTION('',(0.,0.866025403784439,0.5));
#67674=DIRECTION('',(1.,0.,0.));
#67675=DIRECTION('',(0.,-0.866025403784439,-0.5));
#67676=DIRECTION('',(1.,0.,0.));
#67677=DIRECTION('center_axis',(0.,0.5,0.866025403784439));
#67678=DIRECTION('ref_axis',(0.,-0.866025403784439,0.5));
#67679=DIRECTION('',(0.,0.866025403784439,-0.5));
#67680=DIRECTION('',(0.,-0.866025403784439,0.5));
#67681=DIRECTION('',(1.,0.,0.));
#67682=DIRECTION('center_axis',(0.,1.,-3.84592537276713E-16));
#67683=DIRECTION('ref_axis',(0.,3.84592537276713E-16,1.));
#67684=DIRECTION('',(0.,-3.84592537276713E-16,-1.));
#67685=DIRECTION('',(0.,3.84592537276713E-16,1.));
#67686=DIRECTION('',(1.,0.,0.));
#67687=DIRECTION('center_axis',(0.,0.5,-0.866025403784439));
#67688=DIRECTION('ref_axis',(0.,0.866025403784439,0.5));
#67689=DIRECTION('',(0.,-0.866025403784439,-0.5));
#67690=DIRECTION('',(0.,0.866025403784439,0.5));
#67691=DIRECTION('',(1.,0.,0.));
#67692=DIRECTION('center_axis',(0.,-0.5,-0.866025403784439));
#67693=DIRECTION('ref_axis',(0.,0.866025403784439,-0.5));
#67694=DIRECTION('',(0.,-0.866025403784439,0.5));
#67695=DIRECTION('',(0.,0.866025403784439,-0.5));
#67696=DIRECTION('',(1.,0.,0.));
#67697=DIRECTION('center_axis',(0.,-1.,-1.92296268638356E-16));
#67698=DIRECTION('ref_axis',(0.,1.92296268638356E-16,-1.));
#67699=DIRECTION('',(0.,-1.92296268638356E-16,1.));
#67700=DIRECTION('',(0.,1.92296268638356E-16,-1.));
#67701=DIRECTION('center_axis',(1.,0.,0.));
#67702=DIRECTION('ref_axis',(0.,0.,-1.));
#67703=DIRECTION('center_axis',(-1.,0.,0.));
#67704=DIRECTION('ref_axis',(0.,0.,1.));
#67705=DIRECTION('center_axis',(1.,0.,0.));
#67706=DIRECTION('ref_axis',(0.,0.,-1.));
#67707=DIRECTION('center_axis',(1.,0.,0.));
#67708=DIRECTION('ref_axis',(0.,1.,0.));
#67709=DIRECTION('',(-0.707106781186548,0.707106781186547,8.65956056235493E-17));
#67710=DIRECTION('center_axis',(1.,0.,0.));
#67711=DIRECTION('ref_axis',(0.,1.,0.));
#67712=DIRECTION('center_axis',(1.,0.,0.));
#67713=DIRECTION('ref_axis',(0.,0.,-1.));
#67714=DIRECTION('center_axis',(1.,0.,0.));
#67715=DIRECTION('ref_axis',(0.,0.,-1.));
#67716=DIRECTION('center_axis',(1.,0.,0.));
#67717=DIRECTION('ref_axis',(0.,0.,-1.));
#67718=DIRECTION('center_axis',(1.,0.,0.));
#67719=DIRECTION('ref_axis',(0.,0.,-1.));
#67720=DIRECTION('center_axis',(1.,0.,0.));
#67721=DIRECTION('ref_axis',(0.,0.,-1.));
#67722=DIRECTION('center_axis',(1.,0.,0.));
#67723=DIRECTION('ref_axis',(0.,0.,-1.));
#67724=DIRECTION('center_axis',(1.,0.,0.));
#67725=DIRECTION('ref_axis',(0.,0.,-1.));
#67726=DIRECTION('center_axis',(1.,0.,0.));
#67727=DIRECTION('ref_axis',(0.,0.,-1.));
#67728=DIRECTION('center_axis',(1.,0.,0.));
#67729=DIRECTION('ref_axis',(0.,0.,-1.));
#67730=DIRECTION('center_axis',(1.,0.,0.));
#67731=DIRECTION('ref_axis',(0.,0.,-1.));
#67732=DIRECTION('center_axis',(1.,0.,0.));
#67733=DIRECTION('ref_axis',(0.,0.,-1.));
#67734=DIRECTION('center_axis',(1.,0.,0.));
#67735=DIRECTION('ref_axis',(0.,0.,-1.));
#67736=DIRECTION('center_axis',(1.,0.,0.));
#67737=DIRECTION('ref_axis',(0.,0.,-1.));
#67738=DIRECTION('center_axis',(1.,0.,0.));
#67739=DIRECTION('ref_axis',(0.,0.,-1.));
#67740=DIRECTION('center_axis',(1.,0.,0.));
#67741=DIRECTION('ref_axis',(0.,0.,-1.));
#67742=DIRECTION('center_axis',(1.,0.,0.));
#67743=DIRECTION('ref_axis',(0.,0.,-1.));
#67744=DIRECTION('center_axis',(1.,0.,0.));
#67745=DIRECTION('ref_axis',(0.,0.,-1.));
#67746=DIRECTION('',(-1.,0.,0.));
#67747=DIRECTION('center_axis',(1.,0.,0.));
#67748=DIRECTION('ref_axis',(0.,0.,-1.));
#67749=DIRECTION('center_axis',(1.,0.,0.));
#67750=DIRECTION('ref_axis',(0.,0.,-1.));
#67751=DIRECTION('center_axis',(1.,0.,0.));
#67752=DIRECTION('ref_axis',(0.,0.,-1.));
#67753=DIRECTION('center_axis',(1.,0.,0.));
#67754=DIRECTION('ref_axis',(0.,0.,-1.));
#67755=DIRECTION('center_axis',(1.,0.,0.));
#67756=DIRECTION('ref_axis',(0.,0.,-1.));
#67757=DIRECTION('center_axis',(1.,0.,0.));
#67758=DIRECTION('ref_axis',(0.,0.,-1.));
#67759=DIRECTION('center_axis',(1.,0.,0.));
#67760=DIRECTION('ref_axis',(0.,0.,-1.));
#67761=DIRECTION('center_axis',(1.,0.,0.));
#67762=DIRECTION('ref_axis',(0.,0.,-1.));
#67763=DIRECTION('center_axis',(1.,0.,0.));
#67764=DIRECTION('ref_axis',(0.,0.,-1.));
#67765=DIRECTION('center_axis',(1.,0.,0.));
#67766=DIRECTION('ref_axis',(0.,0.,-1.));
#67767=DIRECTION('center_axis',(1.,0.,0.));
#67768=DIRECTION('ref_axis',(0.,0.,-1.));
#67769=DIRECTION('center_axis',(1.,0.,0.));
#67770=DIRECTION('ref_axis',(0.,0.,-1.));
#67771=DIRECTION('center_axis',(1.,0.,0.));
#67772=DIRECTION('ref_axis',(0.,0.,-1.));
#67773=DIRECTION('center_axis',(1.,0.,0.));
#67774=DIRECTION('ref_axis',(0.,0.,-1.));
#67775=DIRECTION('center_axis',(1.,0.,0.));
#67776=DIRECTION('ref_axis',(0.,0.,-1.));
#67777=DIRECTION('center_axis',(1.,0.,0.));
#67778=DIRECTION('ref_axis',(0.,0.,-1.));
#67779=DIRECTION('center_axis',(1.,0.,0.));
#67780=DIRECTION('ref_axis',(0.,0.,-1.));
#67781=DIRECTION('center_axis',(1.,0.,0.));
#67782=DIRECTION('ref_axis',(0.,0.,-1.));
#67783=DIRECTION('center_axis',(1.,0.,0.));
#67784=DIRECTION('ref_axis',(0.,0.,-1.));
#67785=DIRECTION('center_axis',(-1.,0.,0.));
#67786=DIRECTION('ref_axis',(0.,1.,0.));
#67787=DIRECTION('center_axis',(1.,0.,0.));
#67788=DIRECTION('ref_axis',(0.,0.,-1.));
#67789=DIRECTION('',(-0.707106781186547,-0.707106781186548,-8.65956056235493E-17));
#67790=DIRECTION('center_axis',(1.,0.,0.));
#67791=DIRECTION('ref_axis',(0.,0.,-1.));
#87476=CARTESIAN_POINT('',(0.,0.,0.));
#87477=CARTESIAN_POINT('Origin',(-7.7,0.,0.));
#87478=CARTESIAN_POINT('',(-15.1358238829104,-2.94538307225005,0.00197110619363838));
#87479=CARTESIAN_POINT('',(-15.2801761170896,-2.94466557400741,0.00313752023776137));
#87480=CARTESIAN_POINT('',(-7.7,-2.942,-3.60291088309151E-16));
#87481=CARTESIAN_POINT('',(-15.458,1.29046914982061,2.6465053321022));
#87482=CARTESIAN_POINT('Ctrl Pts',(-15.1358238829104,-2.94538307225005,
0.00197110619363838));
#87483=CARTESIAN_POINT('Ctrl Pts',(-15.1415696469556,-2.9461379076381,0.107826186325021));
#87484=CARTESIAN_POINT('Ctrl Pts',(-15.1473154110008,-2.94092576030921,
0.213601568550446));
#87485=CARTESIAN_POINT('Ctrl Pts',(-15.153061175046,-2.92950004699259,0.31869564336318));
#87486=CARTESIAN_POINT('Ctrl Pts',(-15.2059089097093,-2.82440992130234,
1.28531796490334));
#87487=CARTESIAN_POINT('Ctrl Pts',(-15.2587566443725,-2.19366807307829,
2.19430342932105));
#87488=CARTESIAN_POINT('Ctrl Pts',(-15.3116043790358,-1.32498508042342,
2.63183072499184));
#87489=CARTESIAN_POINT('Ctrl Pts',(-15.3604029193572,-0.522860593656641,
3.03583467171792));
#87490=CARTESIAN_POINT('Ctrl Pts',(-15.4092014596786,0.48213979207355,3.03785896067201));
#87491=CARTESIAN_POINT('Ctrl Pts',(-15.458,1.29201644558801,2.64838508500723));
#87492=CARTESIAN_POINT('',(-15.458,-1.28892185405329,2.64462557919714));
#87493=CARTESIAN_POINT('Origin',(-15.458,0.,0.));
#87494=CARTESIAN_POINT('Ctrl Pts',(-15.458,-1.28892185405329,2.64462557919715));
#87495=CARTESIAN_POINT('Ctrl Pts',(-15.4051522653367,-2.16707535766418,
2.21663635799285));
#87496=CARTESIAN_POINT('Ctrl Pts',(-15.3523045306734,-2.80781137912627,
1.32067398609183));
#87497=CARTESIAN_POINT('Ctrl Pts',(-15.2994567960101,-2.92486432853091,
0.356906459573303));
#87498=CARTESIAN_POINT('Ctrl Pts',(-15.2930299030366,-2.93909931481463,
0.239701232447736));
#87499=CARTESIAN_POINT('Ctrl Pts',(-15.2866030100631,-2.94558936356448,
0.121493210473513));
#87500=CARTESIAN_POINT('Ctrl Pts',(-15.2801761170896,-2.94466557400741,
0.00313752023776137));
#87501=CARTESIAN_POINT('Origin',(-7.7,0.,0.));
#87502=CARTESIAN_POINT('',(-14.1358238829104,-2.93775688134926,0.00129066909678663));
#87503=CARTESIAN_POINT('',(-14.2801761170896,-2.93759521907236,0.00112342388299112));
#87504=CARTESIAN_POINT('',(-7.7,-2.942,-3.60291088309151E-16));
#87505=CARTESIAN_POINT('Ctrl Pts',(-14.1358238829104,-2.93775688134926,
0.00129066909678663));
#87506=CARTESIAN_POINT('Ctrl Pts',(-14.1578165723092,-2.93937115251897,
0.409195620159363));
#87507=CARTESIAN_POINT('Ctrl Pts',(-14.1798092617081,-2.86019584296587,
0.816500692953316));
#87508=CARTESIAN_POINT('Ctrl Pts',(-14.2018019511069,-2.69719296954668,
1.18691526487588));
#87509=CARTESIAN_POINT('Ctrl Pts',(-14.2546496857702,-2.30550223779513,
2.07700972569356));
#87510=CARTESIAN_POINT('Ctrl Pts',(-14.3074974204334,-1.42976965241086,
2.75408897290262));
#87511=CARTESIAN_POINT('Ctrl Pts',(-14.3603451550967,-0.469734389951471,
2.90911082424985));
#87512=CARTESIAN_POINT('Ctrl Pts',(-14.41319288976,0.490300872507907,3.06413267559709));
#87513=CARTESIAN_POINT('Ctrl Pts',(-14.4660406244233,1.53463881204239,2.6970971310825));
#87514=CARTESIAN_POINT('Ctrl Pts',(-14.5188883590866,2.18656529744424,1.97550114427565));
#87515=CARTESIAN_POINT('Ctrl Pts',(-14.5717360937499,2.83849178284608,1.25390515746879));
#87516=CARTESIAN_POINT('Ctrl Pts',(-14.6245838284131,3.09800681411528,0.177748728369656));
#87517=CARTESIAN_POINT('Ctrl Pts',(-14.6774315630764,2.84666544889829,-0.761656087067673));
#87518=CARTESIAN_POINT('Ctrl Pts',(-14.7302792977397,2.59532408368129,-1.701060902505));
#87519=CARTESIAN_POINT('Ctrl Pts',(-14.783127032403,1.83312632197811,-2.50371410428052));
#87520=CARTESIAN_POINT('Ctrl Pts',(-14.8359747670663,0.907961517914752,
-2.80338699340931));
#87521=CARTESIAN_POINT('Ctrl Pts',(-14.8888225017296,-0.0172032861486045,
-3.10305988253811));
#87522=CARTESIAN_POINT('Ctrl Pts',(-14.9416702363928,-1.10533513257213,
-2.89975245902016));
#87523=CARTESIAN_POINT('Ctrl Pts',(-14.9945179710561,-1.85968185420569,
-2.28596915792989));
#87524=CARTESIAN_POINT('Ctrl Pts',(-15.0416199416742,-2.53201374022922,
-1.73891821623806));
#87525=CARTESIAN_POINT('Ctrl Pts',(-15.0887219122923,-2.93919516860669,
-0.865795623332123));
#87526=CARTESIAN_POINT('Ctrl Pts',(-15.1358238829104,-2.94538307225005,
0.00197110619363838));
#87527=CARTESIAN_POINT('Ctrl Pts',(-15.2801761170896,-2.94466557400741,
0.00313752023776137));
#87528=CARTESIAN_POINT('Ctrl Pts',(-15.2337552753998,-2.93799312917907,
-0.851734465675268));
#87529=CARTESIAN_POINT('Ctrl Pts',(-15.1873344337101,-2.54453802420963,
-1.71431035888275));
#87530=CARTESIAN_POINT('Ctrl Pts',(-15.1409135920203,-1.88906561096285,
-2.26235996115331));
#87531=CARTESIAN_POINT('Ctrl Pts',(-15.088065857357,-1.14284406664301,-2.88628617422528));
#87532=CARTESIAN_POINT('Ctrl Pts',(-15.0352181226937,-0.0570311006561663,
-3.10256591923317));
#87533=CARTESIAN_POINT('Ctrl Pts',(-14.9823703880304,0.871996126213134,
-2.81455814367286));
#87534=CARTESIAN_POINT('Ctrl Pts',(-14.9295226533672,1.80102335308244,-2.52655036811256));
#87535=CARTESIAN_POINT('Ctrl Pts',(-14.8766749187039,2.5732648408342,-1.73425507198407));
#87536=CARTESIAN_POINT('Ctrl Pts',(-14.8238271840406,2.83659880862163,-0.798275641797322));
#87537=CARTESIAN_POINT('Ctrl Pts',(-14.7709794493773,3.09993277640907,0.137703788389426));
#87538=CARTESIAN_POINT('Ctrl Pts',(-14.718131714714,2.85435922423218,1.21736735263443));
#87539=CARTESIAN_POINT('Ctrl Pts',(-14.6652839800507,2.21177553304593,1.9473366320817));
#87540=CARTESIAN_POINT('Ctrl Pts',(-14.6124362453875,1.56919184185968,2.67730591152896));
#87541=CARTESIAN_POINT('Ctrl Pts',(-14.5595885107242,0.529598011664078,
3.05758090617849));
#87542=CARTESIAN_POINT('Ctrl Pts',(-14.5067407760609,-0.432361259668386,
2.9148644525704));
#87543=CARTESIAN_POINT('Ctrl Pts',(-14.4538930413976,-1.39432053100085,
2.7721479989623));
#87544=CARTESIAN_POINT('Ctrl Pts',(-14.4010453067343,-2.27864524347017,
2.10644009709658));
#87545=CARTESIAN_POINT('Ctrl Pts',(-14.348197572071,-2.68172448593006,1.22146505496284));
#87546=CARTESIAN_POINT('Ctrl Pts',(-14.3255237537439,-2.85466180430726,
0.841774923356542));
#87547=CARTESIAN_POINT('Ctrl Pts',(-14.3028499354168,-2.93901350293065,
0.421723028943609));
#87548=CARTESIAN_POINT('Ctrl Pts',(-14.2801761170896,-2.93759521907236,
0.00112342388299112));
#87549=CARTESIAN_POINT('Origin',(-7.7,0.,0.));
#87550=CARTESIAN_POINT('',(-13.1358238829104,-2.94074805441212,-0.00260717695666907));
#87551=CARTESIAN_POINT('',(-13.2801761170896,-2.94111110959967,-0.00264487064251058));
#87552=CARTESIAN_POINT('',(-7.7,-2.942,-3.60291088309151E-16));
#87553=CARTESIAN_POINT('Ctrl Pts',(-13.1358238829104,-2.94074805441212,
-0.00260717695666907));
#87554=CARTESIAN_POINT('Ctrl Pts',(-13.1740634976629,-2.93465880245723,
0.704816327991579));
#87555=CARTESIAN_POINT('Ctrl Pts',(-13.2123031124153,-2.6782697242631,1.41619979630778));
#87556=CARTESIAN_POINT('Ctrl Pts',(-13.2505427271678,-2.21386422561743,
1.94484407522698));
#87557=CARTESIAN_POINT('Ctrl Pts',(-13.3033904618311,-1.572048696683,2.67543858472817));
#87558=CARTESIAN_POINT('Ctrl Pts',(-13.3562381964943,-0.53292878682618,
3.05700737618249));
#87559=CARTESIAN_POINT('Ctrl Pts',(-13.4090859311576,0.429171271208409,
2.91537721181919));
#87560=CARTESIAN_POINT('Ctrl Pts',(-13.4619336658209,1.391271329243,2.77374704745589));
#87561=CARTESIAN_POINT('Ctrl Pts',(-13.5147814004842,2.27635153545535,2.10891792727497));
#87562=CARTESIAN_POINT('Ctrl Pts',(-13.5676291351475,2.680401504673,1.22436176363895));
#87563=CARTESIAN_POINT('Ctrl Pts',(-13.6204768698108,3.08445147389065,0.339805600002934));
#87564=CARTESIAN_POINT('Ctrl Pts',(-13.673324604474,3.00747120611361,-0.764477607088176));
#87565=CARTESIAN_POINT('Ctrl Pts',(-13.7261723391373,2.48459999269888,-1.58441694249922));
#87566=CARTESIAN_POINT('Ctrl Pts',(-13.7790200738006,1.96172877928415,-2.40435627791026));
#87567=CARTESIAN_POINT('Ctrl Pts',(-13.8318678084639,0.992966620231722,
-2.93995174164124));
#87568=CARTESIAN_POINT('Ctrl Pts',(-13.8847155431272,0.0205212209196415,
-2.94672469674374));
#87569=CARTESIAN_POINT('Ctrl Pts',(-13.9375632777905,-0.951924178392424,
-2.95349765184624));
#87570=CARTESIAN_POINT('Ctrl Pts',(-13.9904110124537,-1.92805281796414,
-2.43144809832029));
#87571=CARTESIAN_POINT('Ctrl Pts',(-14.043258747117,-2.46229269869059,-1.61886848434418));
#87572=CARTESIAN_POINT('Ctrl Pts',(-14.0741137923815,-2.77420759545808,
-1.14444548532719));
#87573=CARTESIAN_POINT('Ctrl Pts',(-14.1049688376459,-2.93549211012882,
-0.570987031933492));
#87574=CARTESIAN_POINT('Ctrl Pts',(-14.1358238829104,-2.93775688134926,
0.00129066909678663));
#87575=CARTESIAN_POINT('Ctrl Pts',(-14.2801761170896,-2.93759521907236,
0.00112342388299112));
#87576=CARTESIAN_POINT('Ctrl Pts',(-14.2500022007535,-2.93570779200279,
-0.558603090240103));
#87577=CARTESIAN_POINT('Ctrl Pts',(-14.2198282844173,-2.78192330778483,
-1.11929958981901));
#87578=CARTESIAN_POINT('Ctrl Pts',(-14.1896543680812,-2.48287763479889,
-1.58713267790547));
#87579=CARTESIAN_POINT('Ctrl Pts',(-14.1368066334179,-1.95911776875739,
-2.40651318623828));
#87580=CARTESIAN_POINT('Ctrl Pts',(-14.0839588987546,-0.98976426422395,
-2.94103202050213));
#87581=CARTESIAN_POINT('Ctrl Pts',(-14.0311111640913,-0.0173102695312365,
-2.9467397656718));
#87582=CARTESIAN_POINT('Ctrl Pts',(-13.9782634294281,0.95514372516147,-2.95244751084146));
#87583=CARTESIAN_POINT('Ctrl Pts',(-13.9254156947648,1.93069821001345,-2.42934416691693));
#87584=CARTESIAN_POINT('Ctrl Pts',(-13.8725679601015,2.4640522158048,-1.61618788323316));
#87585=CARTESIAN_POINT('Ctrl Pts',(-13.8197202254382,2.99740622159616,-0.803031599549377));
#87586=CARTESIAN_POINT('Ctrl Pts',(-13.7668724907749,3.08855974832689,0.30017762389366));
#87587=CARTESIAN_POINT('Ctrl Pts',(-13.7140247561116,2.69590010018066,1.1898495617677));
#87588=CARTESIAN_POINT('Ctrl Pts',(-13.6611770214484,2.30324045203443,2.07952149964175));
#87589=CARTESIAN_POINT('Ctrl Pts',(-13.6083292867851,1.42676762901126,2.7556561519468));
#87590=CARTESIAN_POINT('Ctrl Pts',(-13.5554815521218,0.466565002411474,
2.90962599796443));
#87591=CARTESIAN_POINT('Ctrl Pts',(-13.5026338174585,-0.493637624188301,
3.06359584398207));
#87592=CARTESIAN_POINT('Ctrl Pts',(-13.4497860827952,-1.53757005436468,
2.69540088371229));
#87593=CARTESIAN_POINT('Ctrl Pts',(-13.3969383481319,-2.18871233098836,
1.9731070214835));
#87594=CARTESIAN_POINT('Ctrl Pts',(-13.3580176044512,-2.6682587450335,1.44115963616757));
#87595=CARTESIAN_POINT('Ctrl Pts',(-13.3190968607704,-2.93476077004709,
0.717153505126285));
#87596=CARTESIAN_POINT('Ctrl Pts',(-13.2801761170896,-2.94111110959967,
-0.00264487064251058));
#87597=CARTESIAN_POINT('Origin',(-7.7,0.,0.));
#87598=CARTESIAN_POINT('',(-12.1358238829104,-2.94666731984368,0.000555183168313277));
#87599=CARTESIAN_POINT('',(-12.2801761170896,-2.9465427897585,0.000779102665135559));
#87600=CARTESIAN_POINT('',(-7.7,-2.942,-3.60291088309151E-16));
#87601=CARTESIAN_POINT('Ctrl Pts',(-12.1358238829104,-2.94666731984368,
0.000555183168313277));
#87602=CARTESIAN_POINT('Ctrl Pts',(-12.1374626883532,-2.94674572763455,
0.0307149631628695));
#87603=CARTESIAN_POINT('Ctrl Pts',(-12.139101493796,-2.94632262466987,0.0608724894688986));
#87604=CARTESIAN_POINT('Ctrl Pts',(-12.1407402992388,-2.94539122482773,
0.0910143091064779));
#87605=CARTESIAN_POINT('Ctrl Pts',(-12.1935880339021,-2.91535570600564,
1.06301918831248));
#87606=CARTESIAN_POINT('Ctrl Pts',(-12.2464357685654,-2.35673450139353,
2.01869046311919));
#87607=CARTESIAN_POINT('Ctrl Pts',(-12.2992835032287,-1.52451995638186,
2.52179538823306));
#87608=CARTESIAN_POINT('Ctrl Pts',(-12.352131237892,-0.692305411370191,
3.02490031334693));
#87609=CARTESIAN_POINT('Ctrl Pts',(-12.4049789725552,0.413502474041036,
3.07543888876795));
#87610=CARTESIAN_POINT('Ctrl Pts',(-12.4578267072185,1.28813849951715,2.65034191401869));
#87611=CARTESIAN_POINT('Ctrl Pts',(-12.5106744418818,2.16277452499326,2.22524493926943));
#87612=CARTESIAN_POINT('Ctrl Pts',(-12.5635221765451,2.80623869053425,1.32451241434988));
#87613=CARTESIAN_POINT('Ctrl Pts',(-12.6163699112084,2.9248106062348,0.359299315654169));
#87614=CARTESIAN_POINT('Ctrl Pts',(-12.6692176458717,3.04338252193535,-0.605913783041536));
#87615=CARTESIAN_POINT('Ctrl Pts',(-12.7220653805349,2.63706218779547,-1.63560745551341));
#87616=CARTESIAN_POINT('Ctrl Pts',(-12.7749131151982,1.89132157897925,-2.25976011876333));
#87617=CARTESIAN_POINT('Ctrl Pts',(-12.8277608498615,1.14558097016303,-2.88391278201326));
#87618=CARTESIAN_POINT('Ctrl Pts',(-12.8806085845248,0.0604200866704679,
-3.10252443604124));
#87619=CARTESIAN_POINT('Ctrl Pts',(-12.9334563191881,-0.868820564034781,
-2.81580606293874));
#87620=CARTESIAN_POINT('Ctrl Pts',(-12.9863040538514,-1.79806121474003,
-2.52908768983624));
#87621=CARTESIAN_POINT('Ctrl Pts',(-13.0391517885146,-2.57138163265797,
-1.73703928960327));
#87622=CARTESIAN_POINT('Ctrl Pts',(-13.0919995231779,-2.83578626761092,
-0.801204975712751));
#87623=CARTESIAN_POINT('Ctrl Pts',(-13.1066076430888,-2.90887274212077,
-0.542522556095674));
#87624=CARTESIAN_POINT('Ctrl Pts',(-13.1212157629996,-2.9430742421444,-0.272853816597777));
#87625=CARTESIAN_POINT('Ctrl Pts',(-13.1358238829104,-2.94074805441212,
-0.00260717695666907));
#87626=CARTESIAN_POINT('Ctrl Pts',(-13.2801761170896,-2.94111110959967,
-0.00264487064251058));
#87627=CARTESIAN_POINT('Ctrl Pts',(-13.2662491261071,-2.94338344854597,
-0.260209977074633));
#87628=CARTESIAN_POINT('Ctrl Pts',(-13.2523221351246,-2.91234545461203,
-0.517236314255438));
#87629=CARTESIAN_POINT('Ctrl Pts',(-13.2383951441421,-2.84583880363258,
-0.764731501724886));
#87630=CARTESIAN_POINT('Ctrl Pts',(-13.1855474094788,-2.59347087658213,
-1.70388339851668));
#87631=CARTESIAN_POINT('Ctrl Pts',(-13.1326996748155,-1.83038289941027,
-2.50579442791246));
#87632=CARTESIAN_POINT('Ctrl Pts',(-13.0798519401522,-0.904899930405956,
-2.80441922491318));
#87633=CARTESIAN_POINT('Ctrl Pts',(-13.027004205489,0.0205830385983635,
-3.10304402191389));
#87634=CARTESIAN_POINT('Ctrl Pts',(-12.9741564708257,1.10846099943515,-2.89838258651955));
#87635=CARTESIAN_POINT('Ctrl Pts',(-12.9213087361624,1.86215333580489,-2.28385574206214));
#87636=CARTESIAN_POINT('Ctrl Pts',(-12.8684610014991,2.61584567217464,-1.66932889760473));
#87637=CARTESIAN_POINT('Ctrl Pts',(-12.8156132668358,3.03535238407735,-0.64493664408427));
#87638=CARTESIAN_POINT('Ctrl Pts',(-12.7627655321725,2.92918226774181,0.321719163828909));
#87639=CARTESIAN_POINT('Ctrl Pts',(-12.7099177975092,2.82301215140626,1.28837497174208));
#87640=CARTESIAN_POINT('Ctrl Pts',(-12.657070062846,2.19116520683245,2.19729433404797));
#87641=CARTESIAN_POINT('Ctrl Pts',(-12.6042223281827,1.32205898240464,2.6335853531165));
#87642=CARTESIAN_POINT('Ctrl Pts',(-12.5513745935194,0.45295275797683,3.06987637218503));
#87643=CARTESIAN_POINT('Ctrl Pts',(-12.4985268588561,-0.653412746304991,
3.03353904801619));
#87644=CARTESIAN_POINT('Ctrl Pts',(-12.4456791241928,-1.49201781655651,
2.54116011967247));
#87645=CARTESIAN_POINT('Ctrl Pts',(-12.3928313895296,-2.33062288680803,
2.04878119132876));
#87646=CARTESIAN_POINT('Ctrl Pts',(-12.3399836548663,-2.90146752302926,
1.10036065881016));
#87647=CARTESIAN_POINT('Ctrl Pts',(-12.287135920203,-2.94397977118869,0.128821568406056));
#87648=CARTESIAN_POINT('Ctrl Pts',(-12.2848159858319,-2.94584599357887,
0.0861724947403499));
#87649=CARTESIAN_POINT('Ctrl Pts',(-12.2824960514607,-2.94669407976322,
0.0434788698766825));
#87650=CARTESIAN_POINT('Ctrl Pts',(-12.2801761170896,-2.9465427897585,0.000779102665135559));
#87651=CARTESIAN_POINT('Origin',(-7.7,0.,0.));
#87652=CARTESIAN_POINT('',(-11.1358238829104,-2.93916360235934,0.00220716881453697));
#87653=CARTESIAN_POINT('',(-11.2801761170896,-2.93887905319533,0.00208280935630314));
#87654=CARTESIAN_POINT('',(-7.7,-2.942,-3.60291088309151E-16));
#87655=CARTESIAN_POINT('Ctrl Pts',(-11.1358238829104,-2.93916360235934,
0.00220716881453697));
#87656=CARTESIAN_POINT('Ctrl Pts',(-11.1537096137068,-2.94148269897771,
0.333540081468947));
#87657=CARTESIAN_POINT('Ctrl Pts',(-11.1715953445033,-2.88977704335533,
0.664170570633947));
#87658=CARTESIAN_POINT('Ctrl Pts',(-11.1894810752997,-2.78090778079409,
0.974764066720982));
#87659=CARTESIAN_POINT('Ctrl Pts',(-11.242328809963,-2.45922710884912,1.89248796943232));
#87660=CARTESIAN_POINT('Ctrl Pts',(-11.2951765446263,-1.63847927291341,
2.63527880115994));
#87661=CARTESIAN_POINT('Ctrl Pts',(-11.3480242792896,-0.693308867908512,
2.86407679451984));
#87662=CARTESIAN_POINT('Ctrl Pts',(-11.4008720139528,0.251861537096377,
3.09287478787973));
#87663=CARTESIAN_POINT('Ctrl Pts',(-11.4537197486161,1.32145451117044,2.80767994287192));
#87664=CARTESIAN_POINT('Ctrl Pts',(-11.5065674832794,2.02723577709945,2.13867439663664));
#87665=CARTESIAN_POINT('Ctrl Pts',(-11.5594152179427,2.73301704302846,1.46966885040136));
#87666=CARTESIAN_POINT('Ctrl Pts',(-11.612262952606,3.07498660081242,0.416852602938626));
#87667=CARTESIAN_POINT('Ctrl Pts',(-11.6651106872693,2.89704651038734,-0.539198096916202));
#87668=CARTESIAN_POINT('Ctrl Pts',(-11.7179584219326,2.71910641996226,-1.49524879677103));
#87669=CARTESIAN_POINT('Ctrl Pts',(-11.7708061565958,2.02125668132815,-2.35453394901796));
#87670=CARTESIAN_POINT('Ctrl Pts',(-11.8236538912591,1.12204291994308,-2.72481793114896));
#87671=CARTESIAN_POINT('Ctrl Pts',(-11.8765016259224,0.22282915855803,-3.09510191327996));
#87672=CARTESIAN_POINT('Ctrl Pts',(-11.9293493605857,-0.877748625577962,
-2.97638472529505));
#87673=CARTESIAN_POINT('Ctrl Pts',(-11.982197095249,-1.67731260112992,-2.42285688949995));
#87674=CARTESIAN_POINT('Ctrl Pts',(-12.0334060244694,-2.45208214030059,
-1.88649392247026));
#87675=CARTESIAN_POINT('Ctrl Pts',(-12.0846149536899,-2.94421725535864,
-0.941869096557914));
#87676=CARTESIAN_POINT('Ctrl Pts',(-12.1358238829104,-2.94666731984368,
0.000555183168313277));
#87677=CARTESIAN_POINT('Ctrl Pts',(-12.2801761170896,-2.9465427897585,0.000779102665135559));
#87678=CARTESIAN_POINT('Ctrl Pts',(-12.2296483167974,-2.94324771760488,
-0.929215011409908));
#87679=CARTESIAN_POINT('Ctrl Pts',(-12.1791205165053,-2.46588711038851,
-1.86212281851241));
#87680=CARTESIAN_POINT('Ctrl Pts',(-12.1285927162131,-1.70828039271164,
-2.40112264659498));
#87681=CARTESIAN_POINT('Ctrl Pts',(-12.0757449815499,-0.915888905977512,
-2.96487012290226));
#87682=CARTESIAN_POINT('Ctrl Pts',(-12.0228972468866,0.183073927588378,
-3.0977074272272));
#87683=CARTESIAN_POINT('Ctrl Pts',(-11.9700495122233,1.08696745191729,-2.73899865737196));
#87684=CARTESIAN_POINT('Ctrl Pts',(-11.91720177756,1.9908609762462,-2.38028988751671));
#87685=CARTESIAN_POINT('Ctrl Pts',(-11.8643540428967,2.69968519133814,-1.53003504348128));
#87686=CARTESIAN_POINT('Ctrl Pts',(-11.8115063082334,2.88988497988314,-0.576347710895525));
#87687=CARTESIAN_POINT('Ctrl Pts',(-11.7586585735702,3.08008476842813,0.37733962169024));
#87688=CARTESIAN_POINT('Ctrl Pts',(-11.7058108389069,2.75166013042619,1.43445944282634));
#87689=CARTESIAN_POINT('Ctrl Pts',(-11.6529631042436,2.05452619305162,2.11247106489354));
#87690=CARTESIAN_POINT('Ctrl Pts',(-11.6001153695803,1.35739225567705,2.79048268696074));
#87691=CARTESIAN_POINT('Ctrl Pts',(-11.547267634917,0.291549018929873,3.08938610995905));
#87692=CARTESIAN_POINT('Ctrl Pts',(-11.4944199002537,-0.656480873097509,
2.87274167728717));
#87693=CARTESIAN_POINT('Ctrl Pts',(-11.4415721655904,-1.6045107651249,2.65609724461528));
#87694=CARTESIAN_POINT('Ctrl Pts',(-11.3887244309272,-2.43472731243248,
1.92390495627319));
#87695=CARTESIAN_POINT('Ctrl Pts',(-11.3358766962639,-2.76816376222187,
1.0103866911436));
#87696=CARTESIAN_POINT('Ctrl Pts',(-11.3173098365391,-2.88530913902571,
0.689442650822292));
#87697=CARTESIAN_POINT('Ctrl Pts',(-11.2987429768144,-2.94113646385435,
0.346117368328329));
#87698=CARTESIAN_POINT('Ctrl Pts',(-11.2801761170896,-2.93887905319533,
0.00208280935630314));
#87699=CARTESIAN_POINT('Origin',(-7.7,0.,0.));
#87700=CARTESIAN_POINT('',(-10.1358238829104,-2.93881981982172,-0.00205406958497051));
#87701=CARTESIAN_POINT('',(-10.2801761170896,-2.93909999412443,-0.00218120945484637));
#87702=CARTESIAN_POINT('',(-7.7,-2.942,-3.60291088309151E-16));
#87703=CARTESIAN_POINT('Ctrl Pts',(-10.1358238829104,-2.93881981982172,
-0.00205406958497051));
#87704=CARTESIAN_POINT('Ctrl Pts',(-10.1699565390605,-2.93473247363868,
0.63043906752137));
#87705=CARTESIAN_POINT('Ctrl Pts',(-10.2040891952105,-2.7344359265845,1.2652927625898));
#87706=CARTESIAN_POINT('Ctrl Pts',(-10.2382218513606,-2.35764221671594,
1.76780548958973));
#87707=CARTESIAN_POINT('Ctrl Pts',(-10.2910695860239,-1.77425093552235,
2.54584805225045));
#87708=CARTESIAN_POINT('Ctrl Pts',(-10.3439173206872,-0.7677525585416,3.00663677490463));
#87709=CARTESIAN_POINT('Ctrl Pts',(-10.3967650553505,0.202419260911082,
2.93983664748256));
#87710=CARTESIAN_POINT('Ctrl Pts',(-10.4496127900137,1.17259108036376,2.87303652006049));
#87711=CARTESIAN_POINT('Ctrl Pts',(-10.502460524677,2.10643634228836,2.27864754256218));
#87712=CARTESIAN_POINT('Ctrl Pts',(-10.5553082593403,2.57768516873133,1.42798888019613));
#87713=CARTESIAN_POINT('Ctrl Pts',(-10.6081559940036,3.0489339951743,0.577330217830078));
#87714=CARTESIAN_POINT('Ctrl Pts',(-10.6610037286669,3.05758638613563,-0.529598129403716));
#87715=CARTESIAN_POINT('Ctrl Pts',(-10.7138514633302,2.59969280758565,-1.38751950517789));
#87716=CARTESIAN_POINT('Ctrl Pts',(-10.7666991979934,2.14179922903567,-2.24544088095207));
#87717=CARTESIAN_POINT('Ctrl Pts',(-10.8195469326567,1.21735968097438,-2.85435528526663));
#87718=CARTESIAN_POINT('Ctrl Pts',(-10.87239466732,0.248350640016974,-2.93631316972379));
#87719=CARTESIAN_POINT('Ctrl Pts',(-10.9252424019833,-0.720658400940432,
-3.01827105418095));
#87720=CARTESIAN_POINT('Ctrl Pts',(-10.9780901366466,-1.73423693479395,
-2.5732724187807));
#87721=CARTESIAN_POINT('Ctrl Pts',(-11.0309378713099,-2.3297194477436,-1.80444461423305));
#87722=CARTESIAN_POINT('Ctrl Pts',(-11.0658998751767,-2.72366749590564,
-1.29581806956093));
#87723=CARTESIAN_POINT('Ctrl Pts',(-11.1008618790436,-2.93463036489413,
-0.645463463449812));
#87724=CARTESIAN_POINT('Ctrl Pts',(-11.1358238829104,-2.93916360235934,
0.00220716881453697));
#87725=CARTESIAN_POINT('Ctrl Pts',(-11.2801761170896,-2.93887905319533,
0.00208280935630314));
#87726=CARTESIAN_POINT('Ctrl Pts',(-11.2458952421511,-2.9347110886804,-0.633124536715663));
#87727=CARTESIAN_POINT('Ctrl Pts',(-11.2116143672126,-2.73253231482323,
-1.27074980564275));
#87728=CARTESIAN_POINT('Ctrl Pts',(-11.177333492274,-2.35269386222101,-1.77438537823672));
#87729=CARTESIAN_POINT('Ctrl Pts',(-11.1244857576107,-1.76713116015959,
-2.55079494057035));
#87730=CARTESIAN_POINT('Ctrl Pts',(-11.0716380229475,-0.759349403765581,
-3.00876982332051));
#87731=CARTESIAN_POINT('Ctrl Pts',(-11.0187902882842,0.210631932906051,
-2.93925944229535));
#87732=CARTESIAN_POINT('Ctrl Pts',(-10.9659425536209,1.18061326957769,-2.86974906127019));
#87733=CARTESIAN_POINT('Ctrl Pts',(-10.9130948189576,2.11279418652695,-2.27275341646971));
#87734=CARTESIAN_POINT('Ctrl Pts',(-10.8602470842943,2.58166452491497,-1.42078153172831));
#87735=CARTESIAN_POINT('Ctrl Pts',(-10.807399349631,3.05053486330299,-0.568809646986925));
#87736=CARTESIAN_POINT('Ctrl Pts',(-10.7545516149678,3.05609462312976,0.538138477695383));
#87737=CARTESIAN_POINT('Ctrl Pts',(-10.7017038803045,2.5958059555438,1.39477715827506));
#87738=CARTESIAN_POINT('Ctrl Pts',(-10.6488561456412,2.13551728795784,2.25141583885473));
#87739=CARTESIAN_POINT('Ctrl Pts',(-10.5960084109779,1.20938019295914,2.85774507533179));
#87740=CARTESIAN_POINT('Ctrl Pts',(-10.5431606763146,0.240146021913272,
2.93699536402476));
#87741=CARTESIAN_POINT('Ctrl Pts',(-10.4903129416513,-0.729088149132603,
3.01624565271774));
#87742=CARTESIAN_POINT('Ctrl Pts',(-10.437465206988,-1.74141939622565,2.56841699362663));
#87743=CARTESIAN_POINT('Ctrl Pts',(-10.3846174723248,-2.3347515512458,1.79792855088024));
#87744=CARTESIAN_POINT('Ctrl Pts',(-10.3498036872464,-2.72561292414242,
1.29036433413454));
#87745=CARTESIAN_POINT('Ctrl Pts',(-10.314989902168,-2.93464543616332,0.642778666215291));
#87746=CARTESIAN_POINT('Ctrl Pts',(-10.2801761170896,-2.93909999412443,
-0.00218120945484637));
#87747=CARTESIAN_POINT('Origin',(-7.7,0.,0.));
#87748=CARTESIAN_POINT('',(-9.1358238829104,-2.94651094858123,-0.000827005293144168));
#87749=CARTESIAN_POINT('',(-9.28017611708961,-2.94664335289425,-0.000604394974247732));
#87750=CARTESIAN_POINT('',(-7.7,-2.942,-3.60291088309151E-16));
#87751=CARTESIAN_POINT('Ctrl Pts',(-9.1358238829104,-2.94651094858123,-0.000827005293144167));
#87752=CARTESIAN_POINT('Ctrl Pts',(-9.18620346441409,-2.94304481294294,
0.926466056987759));
#87753=CARTESIAN_POINT('Ctrl Pts',(-9.23658304591779,-2.46886221095953,
1.85681365907283));
#87754=CARTESIAN_POINT('Ctrl Pts',(-9.2869626274215,-1.71498223198426,2.39634075520239));
#87755=CARTESIAN_POINT('Ctrl Pts',(-9.33981036208479,-0.924168812981929,
2.96229989914274));
#87756=CARTESIAN_POINT('Ctrl Pts',(-9.39265809674808,0.174418680626146,
3.09820703168757));
#87757=CARTESIAN_POINT('Ctrl Pts',(-9.44550583141136,1.07931091990927,2.74202498333447));
#87758=CARTESIAN_POINT('Ctrl Pts',(-9.49835356607464,1.98420315919241,2.38584293498135));
#87759=CARTESIAN_POINT('Ctrl Pts',(-9.55120130073791,2.69540014415059,1.53757170573029));
#87760=CARTESIAN_POINT('Ctrl Pts',(-9.6040490354012,2.88826366721313,0.584419421068629));
#87761=CARTESIAN_POINT('Ctrl Pts',(-9.65689677006448,3.08112719027567,-0.368732863593014));
#87762=CARTESIAN_POINT('Ctrl Pts',(-9.70974450472777,2.75565725144258,-1.42676620366524));
#87763=CARTESIAN_POINT('Ctrl Pts',(-9.76259223939106,2.06042025326562,-2.1067229174712));
#87764=CARTESIAN_POINT('Ctrl Pts',(-9.81543997405434,1.36518325508866,-2.78667963127716));
#87765=CARTESIAN_POINT('Ctrl Pts',(-9.86828770871762,0.300179197567841,
-3.08855971881685));
#87766=CARTESIAN_POINT('Ctrl Pts',(-9.9211354433809,-0.648452332654128,
-2.87456477459487));
#87767=CARTESIAN_POINT('Ctrl Pts',(-9.97398317804418,-1.59708386287611,
-2.66056983037287));
#87768=CARTESIAN_POINT('Ctrl Pts',(-10.0268309127075,-2.42934286579924,
-1.93069985438918));
#87769=CARTESIAN_POINT('Ctrl Pts',(-10.0796786473708,-2.76533027455759,
-1.0181166650637));
#87770=CARTESIAN_POINT('Ctrl Pts',(-10.098393725884,-2.88431419646887,-0.694941676639214));
#87771=CARTESIAN_POINT('Ctrl Pts',(-10.1171088043972,-2.94106092887547,
-0.348852709221223));
#87772=CARTESIAN_POINT('Ctrl Pts',(-10.1358238829104,-2.93881981982172,
-0.00205406958497051));
#87773=CARTESIAN_POINT('Ctrl Pts',(-10.2801761170896,-2.93909999412443,
-0.00218120945484637));
#87774=CARTESIAN_POINT('Ctrl Pts',(-10.2621421675047,-2.94140750747045,
-0.336278000594554));
#87775=CARTESIAN_POINT('Ctrl Pts',(-10.2441082179198,-2.88881935641474,
-0.669670196702219));
#87776=CARTESIAN_POINT('Ctrl Pts',(-10.2260742683349,-2.77817338772164,
-0.982529647323611));
#87777=CARTESIAN_POINT('Ctrl Pts',(-10.1732265336716,-2.45393000623006,
-1.89935117637941));
#87778=CARTESIAN_POINT('Ctrl Pts',(-10.1203787990084,-1.63111018029966,
-2.63984600808933));
#87779=CARTESIAN_POINT('Ctrl Pts',(-10.0675310643451,-0.685304300627017,
-2.86600242422521));
#87780=CARTESIAN_POINT('Ctrl Pts',(-10.0146833296818,0.260501579045617,
-3.09215884036109));
#87781=CARTESIAN_POINT('Ctrl Pts',(-9.96183559501851,1.32929351246048,-2.80397684092295));
#87782=CARTESIAN_POINT('Ctrl Pts',(-9.90898786035523,2.03320287127863,-2.13300210134507));
#87783=CARTESIAN_POINT('Ctrl Pts',(-9.85614012569194,2.73711223009679,-1.4620273617672));
#87784=CARTESIAN_POINT('Ctrl Pts',(-9.80329239102865,3.07613901431823,-0.408259882049594));
#87785=CARTESIAN_POINT('Ctrl Pts',(-9.75044465636537,2.89552856401662,0.547289882130422));
#87786=CARTESIAN_POINT('Ctrl Pts',(-9.69759692170208,2.71491811371502,1.50283964631043));
#87787=CARTESIAN_POINT('Ctrl Pts',(-9.6447491870388,2.01467042889038,2.36017169495285));
#87788=CARTESIAN_POINT('Ctrl Pts',(-9.59190145237552,1.11442571902731,2.72794193429589));
#87789=CARTESIAN_POINT('Ctrl Pts',(-9.53905371771224,0.214181009164244,
3.09571217363894));
#87790=CARTESIAN_POINT('Ctrl Pts',(-9.48620598304895,-0.88606072573725,
2.9739206036826));
#87791=CARTESIAN_POINT('Ctrl Pts',(-9.43335824838567,-1.6840750495964,2.41816110039132));
#87792=CARTESIAN_POINT('Ctrl Pts',(-9.38229753795365,-2.45510485003712,
1.88119437422596));
#87793=CARTESIAN_POINT('Ctrl Pts',(-9.33123682752163,-2.94400105383844,
0.939112395821627));
#87794=CARTESIAN_POINT('Ctrl Pts',(-9.28017611708961,-2.94664335289425,
-0.000604394974247732));
#87795=CARTESIAN_POINT('Origin',(-7.7,0.,0.));
#87796=CARTESIAN_POINT('',(-8.1358238829104,-2.94119143690723,0.00265091043401527));
#87797=CARTESIAN_POINT('',(-8.28017611708961,-2.94082616552171,0.00261679703180889));
#87798=CARTESIAN_POINT('',(-7.7,-2.942,-3.60291088309151E-16));
#87799=CARTESIAN_POINT('Ctrl Pts',(-8.1358238829104,-2.94119143690723,0.00265091043401527));
#87800=CARTESIAN_POINT('Ctrl Pts',(-8.14960265510445,-2.94344974034563,
0.257457099259614));
#87801=CARTESIAN_POINT('Ctrl Pts',(-8.16338142729849,-2.91307886267284,
0.511733420342749));
#87802=CARTESIAN_POINT('Ctrl Pts',(-8.17716019949254,-2.84796435061584,
0.756777463120442));
#87803=CARTESIAN_POINT('Ctrl Pts',(-8.23000793415583,-2.5982211654136,1.69663062065564));
#87804=CARTESIAN_POINT('Ctrl Pts',(-8.28285566881911,-1.83737671270331,
2.50067101054199));
#87805=CARTESIAN_POINT('Ctrl Pts',(-8.33570340348239,-0.912731648410138,
2.80188044160635));
#87806=CARTESIAN_POINT('Ctrl Pts',(-8.38855113814568,0.0119134158830346,
3.10308987267071));
#87807=CARTESIAN_POINT('Ctrl Pts',(-8.44139887280896,1.1003590917591,2.90146834491308));
#87808=CARTESIAN_POINT('Ctrl Pts',(-8.49424660747225,1.85576545901611,2.289049504093));
#87809=CARTESIAN_POINT('Ctrl Pts',(-8.54709434213553,2.61117182627314,1.67663066327292));
#87810=CARTESIAN_POINT('Ctrl Pts',(-8.59994207679881,3.0335388849111,0.653414509390389));
#87811=CARTESIAN_POINT('Ctrl Pts',(-8.6527898114621,2.93006986026258,-0.313534184813269));
#87812=CARTESIAN_POINT('Ctrl Pts',(-8.70563754612538,2.82660083561406,-1.28048287901691));
#87813=CARTESIAN_POINT('Ctrl Pts',(-8.75848528078866,2.19729572767907,-2.19116411354167));
#87814=CARTESIAN_POINT('Ctrl Pts',(-8.81133301545195,1.32941177541667,-2.62988163278296));
#87815=CARTESIAN_POINT('Ctrl Pts',(-8.86418075011523,0.461527823154263,
-3.06859915202426));
#87816=CARTESIAN_POINT('Ctrl Pts',(-8.91702848477852,-0.644934973435559,
-3.0353529559821));
#87817=CARTESIAN_POINT('Ctrl Pts',(-8.9698762194418,-1.48491246668953,-2.54531884787264));
#87818=CARTESIAN_POINT('Ctrl Pts',(-9.02272395410509,-2.3248899599435,-2.05528473976319));
#87819=CARTESIAN_POINT('Ctrl Pts',(-9.07557168876836,-2.89838214986163,
-1.10846271958645));
#87820=CARTESIAN_POINT('Ctrl Pts',(-9.12841942343164,-2.9436085726224,-0.137046131830142));
#87821=CARTESIAN_POINT('Ctrl Pts',(-9.13088757659123,-2.94572078687236,
-0.0916779635326883));
#87822=CARTESIAN_POINT('Ctrl Pts',(-9.13335572975081,-2.94668075851954,
-0.0462561500620593));
#87823=CARTESIAN_POINT('Ctrl Pts',(-9.1358238829104,-2.94651094858123,-0.000827005293144167));
#87824=CARTESIAN_POINT('Ctrl Pts',(-9.28017611708961,-2.94664335289425,
-0.000604394974247732));
#87825=CARTESIAN_POINT('Ctrl Pts',(-9.27838909285835,-2.94673582815359,
-0.033492630595535));
#87826=CARTESIAN_POINT('Ctrl Pts',(-9.27660206862708,-2.94623270946163,
-0.0663779691882953));
#87827=CARTESIAN_POINT('Ctrl Pts',(-9.27481504439582,-2.94512524663853,
-0.099242942979859));
#87828=CARTESIAN_POINT('Ctrl Pts',(-9.22196730973253,-2.9123742070047,-1.07116004643351));
#87829=CARTESIAN_POINT('Ctrl Pts',(-9.16911957506925,-2.35108521492026,
-2.02526681671459));
#87830=CARTESIAN_POINT('Ctrl Pts',(-9.11627184040597,-1.51746837275248,
-2.52604465871351));
#87831=CARTESIAN_POINT('Ctrl Pts',(-9.06342410574268,-0.683851530584683,
-3.02682250071243));
#87832=CARTESIAN_POINT('Ctrl Pts',(-9.0105763710794,0.422093161666457,-3.07427141442917));
#87833=CARTESIAN_POINT('Ctrl Pts',(-8.95772863641611,1.29553805405546,-2.64673251965762));
#87834=CARTESIAN_POINT('Ctrl Pts',(-8.90488090175283,2.16898294644444,-2.21919362488608));
#87835=CARTESIAN_POINT('Ctrl Pts',(-8.85203316708954,2.8099280389713,-1.31666692162628));
#87836=CARTESIAN_POINT('Ctrl Pts',(-8.79918543242626,2.92580281968231,-0.351126388153944));
#87837=CARTESIAN_POINT('Ctrl Pts',(-8.74633769776298,3.04167760039333,0.614414145318391));
#87838=CARTESIAN_POINT('Ctrl Pts',(-8.6934899630997,2.63248206928852,1.64296850900325));
#87839=CARTESIAN_POINT('Ctrl Pts',(-8.64064222843642,1.88500062868308,2.26503521164317));
#87840=CARTESIAN_POINT('Ctrl Pts',(-8.58779449377313,1.13751918807765,2.88710191428309));
#87841=CARTESIAN_POINT('Ctrl Pts',(-8.53494675910984,0.051751837971596,
3.10268095587807));
#87842=CARTESIAN_POINT('Ctrl Pts',(-8.48209902444656,-0.876684069716822,
2.81336754122595));
#87843=CARTESIAN_POINT('Ctrl Pts',(-8.42925128978327,-1.80511997740523,
2.52405412657384));
#87844=CARTESIAN_POINT('Ctrl Pts',(-8.37640355512,-2.57622444267601,1.72984825567463));
#87845=CARTESIAN_POINT('Ctrl Pts',(-8.32355582045671,-2.83801344879435,
0.793278982818404));
#87846=CARTESIAN_POINT('Ctrl Pts',(-8.30909591933435,-2.90964269018971,
0.537020144742652));
#87847=CARTESIAN_POINT('Ctrl Pts',(-8.29463601821198,-2.94314211175223,
0.270103293504598));
#87848=CARTESIAN_POINT('Ctrl Pts',(-8.28017611708961,-2.94082616552171,
0.00261679703180889));
#87849=CARTESIAN_POINT('Origin',(-7.7,0.,0.));
#87850=CARTESIAN_POINT('',(-7.1358238829104,-2.93757269053894,-0.0010613151321931));
#87851=CARTESIAN_POINT('',(-7.28017611708961,-2.93772161116193,-0.00124778266073289));
#87852=CARTESIAN_POINT('',(-7.7,-2.942,-3.60291088309151E-16));
#87853=CARTESIAN_POINT('Ctrl Pts',(-7.1358238829104,-2.93757269053894,-0.0010613151321931));
#87854=CARTESIAN_POINT('Ctrl Pts',(-7.16584958045808,-2.93576229085772,
0.555920429035681));
#87855=CARTESIAN_POINT('Ctrl Pts',(-7.19587527800575,-2.78357509105504,
1.11381923203582));
#87856=CARTESIAN_POINT('Ctrl Pts',(-7.22590097555343,-2.48729794486864,
1.58017783952249));
#87857=CARTESIAN_POINT('Ctrl Pts',(-7.27874871021672,-1.96582543008058,
2.40100792705857));
#87858=CARTESIAN_POINT('Ctrl Pts',(-7.33159644488001,-0.997977548263203,
2.93825620062515));
#87859=CARTESIAN_POINT('Ctrl Pts',(-7.3844441795433,-0.0255452633823754,
2.94668636108162));
#87860=CARTESIAN_POINT('Ctrl Pts',(-7.43729191420658,0.946887021498432,
2.95511652153809));
#87861=CARTESIAN_POINT('Ctrl Pts',(-7.49013964886985,1.92390370944269,2.43472856888446));
#87862=CARTESIAN_POINT('Ctrl Pts',(-7.54298738353314,2.45952857579088,1.62306261614694));
#87863=CARTESIAN_POINT('Ctrl Pts',(-7.59583511819642,2.99515344213909,0.811396663409416));
#87864=CARTESIAN_POINT('Ctrl Pts',(-7.64868285285971,3.08938648689121,-0.291547289412031));
#87865=CARTESIAN_POINT('Ctrl Pts',(-7.70153058752299,2.69921340122809,-1.18231133196649));
#87866=CARTESIAN_POINT('Ctrl Pts',(-7.75437832218628,2.30904031556496,-2.07307537452096));
#87867=CARTESIAN_POINT('Ctrl Pts',(-7.80722605684956,1.43446109948659,-2.75165950680844));
#87868=CARTESIAN_POINT('Ctrl Pts',(-7.86007379151284,0.474692615678287,
-2.90831222390001));
#87869=CARTESIAN_POINT('Ctrl Pts',(-7.91292152617613,-0.485075868130016,
-3.06496494099157));
#87870=CARTESIAN_POINT('Ctrl Pts',(-7.96576926083941,-1.53003361966824,
-2.69968624288721));
#87871=CARTESIAN_POINT('Ctrl Pts',(-8.0186169955027,-2.18319153659025,-1.979213931243));
#87872=CARTESIAN_POINT('Ctrl Pts',(-8.05768595797193,-2.66605428000392,
-1.44658739799432));
#87873=CARTESIAN_POINT('Ctrl Pts',(-8.09675492044117,-2.93478813978928,
-0.719838240845876));
#87874=CARTESIAN_POINT('Ctrl Pts',(-8.1358238829104,-2.94119143690723,0.00265091043401527));
#87875=CARTESIAN_POINT('Ctrl Pts',(-8.28017611708961,-2.94082616552171,
0.00261679703180889));
#87876=CARTESIAN_POINT('Ctrl Pts',(-8.24178828354869,-2.93467784143329,
-0.707500583034972));
#87877=CARTESIAN_POINT('Ctrl Pts',(-8.20340045000778,-2.67610823149551,
-1.4216327364097));
#87878=CARTESIAN_POINT('Ctrl Pts',(-8.16501261646686,-2.20842183533617,
-1.95102149586555));
#87879=CARTESIAN_POINT('Ctrl Pts',(-8.11216488180358,-1.56456766879375,
-2.67982002688002));
#87880=CARTESIAN_POINT('Ctrl Pts',(-8.0593171471403,-0.524385788743001,
-3.0584844140957));
#87881=CARTESIAN_POINT('Ctrl Pts',(-8.00646941247701,0.437314731902111,
-2.91416672573489));
#87882=CARTESIAN_POINT('Ctrl Pts',(-7.95362167781373,1.39901525254722,-2.76984903737408));
#87883=CARTESIAN_POINT('Ctrl Pts',(-7.90077394315044,2.2822344137867,-2.1025492734368));
#87884=CARTESIAN_POINT('Ctrl Pts',(-7.84792620848715,2.68381150000848,-1.21686799306303));
#87885=CARTESIAN_POINT('Ctrl Pts',(-7.79507847382387,3.08538858623026,-0.331186712689277));
#87886=CARTESIAN_POINT('Ctrl Pts',(-7.74223073916059,3.00532359743435,0.772876084120949));
#87887=CARTESIAN_POINT('Ctrl Pts',(-7.68938300449731,2.48016358739293,1.59135177125903));
#87888=CARTESIAN_POINT('Ctrl Pts',(-7.63653526983403,1.9550035773515,2.40982745839712));
#87889=CARTESIAN_POINT('Ctrl Pts',(-7.58368753517074,0.98474854606456,2.94271603586306));
#87890=CARTESIAN_POINT('Ctrl Pts',(-7.53083980050746,0.0122882426526789,
2.94677126346982));
#87891=CARTESIAN_POINT('Ctrl Pts',(-7.47799206584417,-0.960172060759209,
2.95082649107658));
#87892=CARTESIAN_POINT('Ctrl Pts',(-7.42514433118089,-1.93483763629604,
2.42604836882414));
#87893=CARTESIAN_POINT('Ctrl Pts',(-7.37229659651761,-2.46680546536339,
1.61198097884942));
#87894=CARTESIAN_POINT('Ctrl Pts',(-7.34158977004161,-2.77590185184169,
1.13897250946104));
#87895=CARTESIAN_POINT('Ctrl Pts',(-7.31088294356561,-2.93553842718574,
0.568296682012325));
#87896=CARTESIAN_POINT('Ctrl Pts',(-7.28017611708961,-2.93772161116193,
-0.00124778266073289));
#87897=CARTESIAN_POINT('Origin',(-7.7,0.,0.));
#87898=CARTESIAN_POINT('',(-6.1358238829104,-2.94505049637757,-0.00196725817694088));
#87899=CARTESIAN_POINT('',(-6.28017611708961,-2.94535604779933,-0.00180876985891124));
#87900=CARTESIAN_POINT('',(-7.7,-2.942,-3.60291088309151E-16));
#87901=CARTESIAN_POINT('Ctrl Pts',(-6.1358238829104,-2.94505049637757,-0.00196725817694088));
#87902=CARTESIAN_POINT('Ctrl Pts',(-6.18209650581171,-2.93847787371737,
0.850848357286048));
#87903=CARTESIAN_POINT('Ctrl Pts',(-6.22836912871302,-2.54719747420371,
1.70892155386477));
#87904=CARTESIAN_POINT('Ctrl Pts',(-6.27464175161433,-1.89517178337686,
2.25653206991563));
#87905=CARTESIAN_POINT('Ctrl Pts',(-6.32748948627761,-1.15049645395035,
2.88195534260979));
#87906=CARTESIAN_POINT('Ctrl Pts',(-6.3803372209409,-0.0657098796553496,
3.10241694474892));
#87907=CARTESIAN_POINT('Ctrl Pts',(-6.43318495560419,0.864018279731717,
2.81728335162707));
#87908=CARTESIAN_POINT('Ctrl Pts',(-6.48603269026747,1.79374643911876,2.53214975850523));
#87909=CARTESIAN_POINT('Ctrl Pts',(-6.53888042493076,2.56841618359787,1.74142097012241));
#87910=CARTESIAN_POINT('Ctrl Pts',(-6.59172815959404,2.83441606285926,0.806038866104609));
#87911=CARTESIAN_POINT('Ctrl Pts',(-6.64457589425732,3.10041594212064,-0.129343237913193));
#87912=CARTESIAN_POINT('Ctrl Pts',(-6.69742362892061,2.8577459561643,-1.20937865756599));
#87913=CARTESIAN_POINT('Ctrl Pts',(-6.75027136358389,2.2171770319462,-1.94106648007633));
#87914=CARTESIAN_POINT('Ctrl Pts',(-6.80311909824717,1.57660810772809,-2.67275430258668));
#87915=CARTESIAN_POINT('Ctrl Pts',(-6.85596683291045,0.53814024524822,-3.05609452795455));
#87916=CARTESIAN_POINT('Ctrl Pts',(-6.90881456757374,-0.424199875648816,
-2.91610485692219));
#87917=CARTESIAN_POINT('Ctrl Pts',(-6.96166230223702,-1.38653999654583,
-2.77611518588984));
#87918=CARTESIAN_POINT('Ctrl Pts',(-7.01451003690031,-2.27275237586001,
-2.11279561845726));
#87919=CARTESIAN_POINT('Ctrl Pts',(-7.06735777156359,-2.67830999163772,
-1.2289298839882));
#87920=CARTESIAN_POINT('Ctrl Pts',(-7.09017980867919,-2.85344807501569,
-0.847236766472653));
#87921=CARTESIAN_POINT('Ctrl Pts',(-7.1130018457948,-2.938948745455,-0.424413945589069));
#87922=CARTESIAN_POINT('Ctrl Pts',(-7.1358238829104,-2.93757269053894,-0.0010613151321931));
#87923=CARTESIAN_POINT('Ctrl Pts',(-7.28017611708961,-2.93772161116193,
-0.00124778266073289));
#87924=CARTESIAN_POINT('Ctrl Pts',(-7.25803520890233,-2.93929577826156,
-0.411913199705981));
#87925=CARTESIAN_POINT('Ctrl Pts',(-7.23589430071504,-2.85900970571129,
-0.821990419652761));
#87926=CARTESIAN_POINT('Ctrl Pts',(-7.21375339252776,-2.69386683455209,
-1.19444269758718));
#87927=CARTESIAN_POINT('Ctrl Pts',(-7.16090565786447,-2.29969029207556,
-2.08344232635207));
#87928=CARTESIAN_POINT('Ctrl Pts',(-7.10805792320119,-1.4220671245246,-2.75808492618488));
#87929=CARTESIAN_POINT('Ctrl Pts',(-7.0552101885379,-0.461603659066119,
-2.9104181730562));
#87930=CARTESIAN_POINT('Ctrl Pts',(-7.00236245387462,0.498859806392379,
-3.06275141992753));
#87931=CARTESIAN_POINT('Ctrl Pts',(-6.94951471921134,1.5421635697584,-2.69277531383738));
#87932=CARTESIAN_POINT('Ctrl Pts',(-6.89666698454805,2.19207352029423,-1.9693718698468));
#87933=CARTESIAN_POINT('Ctrl Pts',(-6.84381924988477,2.84198347083005,-1.24596842585625));
#87934=CARTESIAN_POINT('Ctrl Pts',(-6.79097151522149,3.09849960853568,-0.169137643965288));
#87935=CARTESIAN_POINT('Ctrl Pts',(-6.7381237805582,2.84453069017054,0.769582375575847));
#87936=CARTESIAN_POINT('Ctrl Pts',(-6.68527604589492,2.59056177180539,1.70830239511698));
#87937=CARTESIAN_POINT('Ctrl Pts',(-6.63242831123163,1.82610779736946,2.50891165230829));
#87938=CARTESIAN_POINT('Ctrl Pts',(-6.57958057656835,0.900117051627725,
2.80595815604724));
#87939=CARTESIAN_POINT('Ctrl Pts',(-6.52673284190507,-0.0258736941140224,
3.10300465978619));
#87940=CARTESIAN_POINT('Ctrl Pts',(-6.47388510724178,-1.11340121116158,
2.89648841007276));
#87941=CARTESIAN_POINT('Ctrl Pts',(-6.4210373725785,-1.86604468884618,2.28067733345775));
#87942=CARTESIAN_POINT('Ctrl Pts',(-6.37408362074887,-2.53474761987163,
1.7335462094929));
#87943=CARTESIAN_POINT('Ctrl Pts',(-6.32712986891924,-2.93909873492038,
0.863324648112405));
#87944=CARTESIAN_POINT('Ctrl Pts',(-6.28017611708961,-2.94535604779933,
-0.00180876985891124));
#87945=CARTESIAN_POINT('Origin',(-7.7,0.,0.));
#87946=CARTESIAN_POINT('',(-5.1358238829104,-2.94346675723798,0.0024934893022114));
#87947=CARTESIAN_POINT('',(-5.28017611708961,-2.94309162548594,0.00256319306684998));
#87948=CARTESIAN_POINT('',(-7.7,-2.942,-3.60291088309151E-16));
#87949=CARTESIAN_POINT('Ctrl Pts',(-5.1358238829104,-2.94346675723798,0.0024934893022114));
#87950=CARTESIAN_POINT('Ctrl Pts',(-5.14549569650206,-2.94507633932214,
0.18099679752495));
#87951=CARTESIAN_POINT('Ctrl Pts',(-5.15516751009372,-2.93022859135991,
0.359232954535137));
#87952=CARTESIAN_POINT('Ctrl Pts',(-5.16483932368538,-2.89796164657921,
0.534257771161184));
#87953=CARTESIAN_POINT('Ctrl Pts',(-5.21768705834866,-2.72165190694203,
1.49061047387653));
#87954=CARTESIAN_POINT('Ctrl Pts',(-5.27053479301194,-2.02526828700205,
2.35108422924666));
#87955=CARTESIAN_POINT('Ctrl Pts',(-5.32338252767523,-1.12668717677613,
2.72290085694465));
#87956=CARTESIAN_POINT('Ctrl Pts',(-5.37623026233851,-0.228106066550204,
3.09471748464264));
#87957=CARTESIAN_POINT('Ctrl Pts',(-5.4290779970018,0.872672533961652,2.97787698466847));
#87958=CARTESIAN_POINT('Ctrl Pts',(-5.48192573166508,1.67317912706062,2.42571323116108));
#87959=CARTESIAN_POINT('Ctrl Pts',(-5.53477346632837,2.47368572015958,1.87354947765369));
#87960=CARTESIAN_POINT('Ctrl Pts',(-5.58762120099164,2.97392030584565,0.886062470613057));
#87961=CARTESIAN_POINT('Ctrl Pts',(-5.64046893565493,2.94554212522987,-0.0859922064235157));
#87962=CARTESIAN_POINT('Ctrl Pts',(-5.69331667031821,2.9171639446141,-1.05804688346009));
#87963=CARTESIAN_POINT('Ctrl Pts',(-5.7461644049815,2.3601729976965,-2.01466923049262));
#87964=CARTESIAN_POINT('Ctrl Pts',(-5.79901213964479,1.52881746953169,-2.51919237374194));
#87965=CARTESIAN_POINT('Ctrl Pts',(-5.85185987430807,0.697461941366897,
-3.02371551699126));
#87966=CARTESIAN_POINT('Ctrl Pts',(-5.90470760897135,-0.408258168045107,
-3.07613945645739));
#87967=CARTESIAN_POINT('Ctrl Pts',(-5.95755534363463,-1.28361772349481,
-2.65253437508267));
#87968=CARTESIAN_POINT('Ctrl Pts',(-6.01040307829791,-2.15897727894452,
-2.22892929370794));
#87969=CARTESIAN_POINT('Ctrl Pts',(-6.0632508129612,-2.80397628043193,-1.32929519149237));
#87970=CARTESIAN_POINT('Ctrl Pts',(-6.11609854762449,-2.92419373889664,
-0.364285668760009));
#87971=CARTESIAN_POINT('Ctrl Pts',(-6.12267365938646,-2.93915073242118,
-0.244222897786757));
#87972=CARTESIAN_POINT('Ctrl Pts',(-6.12924877114843,-2.94598443367894,
-0.12314815591822));
#87973=CARTESIAN_POINT('Ctrl Pts',(-6.1358238829104,-2.94505049637757,-0.00196725817694088));
#87974=CARTESIAN_POINT('Ctrl Pts',(-6.28017611708961,-2.94535604779933,
-0.00180876985891124));
#87975=CARTESIAN_POINT('Ctrl Pts',(-6.27428213425596,-2.94614151207547,
-0.110406726691919));
#87976=CARTESIAN_POINT('Ctrl Pts',(-6.2683881514223,-2.94065416034498,-0.21892450898504));
#87977=CARTESIAN_POINT('Ctrl Pts',(-6.26249416858865,-2.92862945740852,
-0.326712995330997));
#87978=CARTESIAN_POINT('Ctrl Pts',(-6.20964643392537,-2.82081130996463,
-1.29318634398818));
#87979=CARTESIAN_POINT('Ctrl Pts',(-6.15679869926208,-2.18741557675519,
-2.20102713778601));
#87980=CARTESIAN_POINT('Ctrl Pts',(-6.1039509645988,-1.31756673364422,-2.63583568958937));
#87981=CARTESIAN_POINT('Ctrl Pts',(-6.05110322993552,-0.447717890533236,
-3.07064424139274));
#87982=CARTESIAN_POINT('Ctrl Pts',(-5.99825549527223,0.658584062479277,
-3.03242055120164));
#87983=CARTESIAN_POINT('Ctrl Pts',(-5.94540776060895,1.49634839757276,-2.5386124858277));
#87984=CARTESIAN_POINT('Ctrl Pts',(-5.89256002594566,2.33411273266621,-2.04480442045378));
#87985=CARTESIAN_POINT('Ctrl Pts',(-5.83971229128238,2.90333944984063,-1.09541197989705));
#87986=CARTESIAN_POINT('Ctrl Pts',(-5.7868645566191,2.94419513434113,-0.123801821640741));
#87987=CARTESIAN_POINT('Ctrl Pts',(-5.73401682195581,2.98505081884163,0.847808336615591));
#87988=CARTESIAN_POINT('Ctrl Pts',(-5.68116908729253,2.49753547066817,1.8416362125715));
#87989=CARTESIAN_POINT('Ctrl Pts',(-5.62832135262925,1.70418393198402,2.40403182301857));
#87990=CARTESIAN_POINT('Ctrl Pts',(-5.57547361796596,0.910832393299871,
2.96642743346563));
#87991=CARTESIAN_POINT('Ctrl Pts',(-5.52262588330268,-0.188355335894953,
3.09739077840386));
#87992=CARTESIAN_POINT('Ctrl Pts',(-5.4697781486394,-1.09163593871943,2.73714136599013));
#87993=CARTESIAN_POINT('Ctrl Pts',(-5.41693041397611,-1.99491654154391,
2.3768919535764));
#87994=CARTESIAN_POINT('Ctrl Pts',(-5.36408267931283,-2.70229001799803,
1.5254297838107));
#87995=CARTESIAN_POINT('Ctrl Pts',(-5.31123494464955,-2.89086346732779,
0.571419542361142));
#87996=CARTESIAN_POINT('Ctrl Pts',(-5.30088200212957,-2.92780526046507,
0.384527648959713));
#87997=CARTESIAN_POINT('Ctrl Pts',(-5.29052905960959,-2.94483688929665,
0.19370023348868));
#87998=CARTESIAN_POINT('Ctrl Pts',(-5.28017611708961,-2.94309162548594,
0.00256319306684998));
#87999=CARTESIAN_POINT('Origin',(-7.7,0.,0.));
#88000=CARTESIAN_POINT('',(-4.1358238829104,-2.93721437885968,0.000152849678604627));
#88001=CARTESIAN_POINT('',(-4.2801761170896,-2.93720779641154,-5.3281763612922E-5));
#88002=CARTESIAN_POINT('',(-7.7,-2.942,-3.60291088309151E-16));
#88003=CARTESIAN_POINT('Ctrl Pts',(-4.1358238829104,-2.93721437885968,0.000152849678604627));
#88004=CARTESIAN_POINT('Ctrl Pts',(-4.16174262185569,-2.93743789235776,
0.481096322078444));
#88005=CARTESIAN_POINT('Ctrl Pts',(-4.18766136080098,-2.82590721058178,
0.961942138436253));
#88006=CARTESIAN_POINT('Ctrl Pts',(-4.21358009974627,-2.60205478700782,
1.38308494226313));
#88007=CARTESIAN_POINT('Ctrl Pts',(-4.26642783440955,-2.14562465320618,
2.24178579182884));
#88008=CARTESIAN_POINT('Ctrl Pts',(-4.31927556907284,-1.22222466387983,
2.85227550533413));
#88009=CARTESIAN_POINT('Ctrl Pts',(-4.37212330373612,-0.25335677173094,
2.93588545711232));
#88010=CARTESIAN_POINT('Ctrl Pts',(-4.42497103839941,0.715511120417946,
3.01949540889051));
#88011=CARTESIAN_POINT('Ctrl Pts',(-4.47781877306269,1.72984691538937,2.57622559894159));
#88012=CARTESIAN_POINT('Ctrl Pts',(-4.53066650772597,2.32663943477293,1.80841422559673));
#88013=CARTESIAN_POINT('Ctrl Pts',(-4.58351424238926,2.9234319541565,1.04060285225185));
#88014=CARTESIAN_POINT('Ctrl Pts',(-4.63636197705254,3.1026811979522,-0.0517500844889977));
#88015=CARTESIAN_POINT('Ctrl Pts',(-4.68920971171582,2.78256573751978,-0.970021127403228));
#88016=CARTESIAN_POINT('Ctrl Pts',(-4.74205744637911,2.46245027708737,-1.88829217031744));
#88017=CARTESIAN_POINT('Ctrl Pts',(-4.7949051810424,1.64297011242686,-2.63248131940505));
#88018=CARTESIAN_POINT('Ctrl Pts',(-4.84775291570568,0.698191187988024,
-2.86289052114596));
#88019=CARTESIAN_POINT('Ctrl Pts',(-4.90060065036896,-0.246587736450821,
-3.09329972288687));
#88020=CARTESIAN_POINT('Ctrl Pts',(-4.95344838503224,-1.316665420668,-2.80992897728107));
#88021=CARTESIAN_POINT('Ctrl Pts',(-5.00629611969553,-2.02358633310939,
-2.14212777944788));
#88022=CARTESIAN_POINT('Ctrl Pts',(-5.04947204076715,-2.60113164728262,
-1.59654277012084));
#88023=CARTESIAN_POINT('Ctrl Pts',(-5.09264796183877,-2.93628142551449,
-0.794362723217666));
#88024=CARTESIAN_POINT('Ctrl Pts',(-5.1358238829104,-2.94346675723798,0.0024934893022114));
#88025=CARTESIAN_POINT('Ctrl Pts',(-5.28017611708961,-2.94309162548594,
0.00256319306684998));
#88026=CARTESIAN_POINT('Ctrl Pts',(-5.2376813249463,-2.93592799807001,-0.781979828198723));
#88027=CARTESIAN_POINT('Ctrl Pts',(-5.195186532803,-2.61241459108027,-1.57173935609301));
#88028=CARTESIAN_POINT('Ctrl Pts',(-5.15269174065969,-2.05092138691181,
-2.11597101700905));
#88029=CARTESIAN_POINT('Ctrl Pts',(-5.09984400599641,-1.35263243496063,
-2.79279302179629));
#88030=CARTESIAN_POINT('Ctrl Pts',(-5.04699627133313,-0.28628110885286,
-3.08987871823736));
#88031=CARTESIAN_POINT('Ctrl Pts',(-4.99414853666985,0.661378020646438,
-2.8716181838679));
#88032=CARTESIAN_POINT('Ctrl Pts',(-4.94130080200656,1.60903715014574,-2.65335764949843));
#88033=CARTESIAN_POINT('Ctrl Pts',(-4.88845306734327,2.43800408303655,-1.91975088431843));
#88034=CARTESIAN_POINT('Ctrl Pts',(-4.83560533267999,2.76988247494261,-1.0056654290317));
#88035=CARTESIAN_POINT('Ctrl Pts',(-4.78275759801671,3.10176086684867,-0.0915799737449764));
#88036=CARTESIAN_POINT('Ctrl Pts',(-4.72990986335342,2.93655071776997,1.0029841716485));
#88037=CARTESIAN_POINT('Ctrl Pts',(-4.67706212869014,2.34966506772764,1.7783942053389));
#88038=CARTESIAN_POINT('Ctrl Pts',(-4.62421439402686,1.7627794176853,2.55380423902931));
#88039=CARTESIAN_POINT('Ctrl Pts',(-4.57136665936357,0.754218266679339,
3.01006016101665));
#88040=CARTESIAN_POINT('Ctrl Pts',(-4.51851892470029,-0.215643143023527,
2.93889603677497));
#88041=CARTESIAN_POINT('Ctrl Pts',(-4.46567119003701,-1.18550455272636,
2.86773191253328));
#88042=CARTESIAN_POINT('Ctrl Pts',(-4.41282345537372,-2.11666622112609,
2.26914774206261));
#88043=CARTESIAN_POINT('Ctrl Pts',(-4.35997572071044,-2.58408324300676,
1.41637765920455));
#88044=CARTESIAN_POINT('Ctrl Pts',(-4.33337585283683,-2.81934840816703,
0.987152609632971));
#88045=CARTESIAN_POINT('Ctrl Pts',(-4.30677598496322,-2.93712784426376,
0.49353173908822));
#88046=CARTESIAN_POINT('Ctrl Pts',(-4.2801761170896,-2.93720779641154,-5.3281763612922E-5));
#88047=CARTESIAN_POINT('Origin',(-7.7,0.,0.));
#88048=CARTESIAN_POINT('',(-3.1358238829104,-2.94290902102838,-0.00259068251834249));
#88049=CARTESIAN_POINT('',(-3.2801761170896,-2.94328604584299,-0.00252931999075325));
#88050=CARTESIAN_POINT('',(-7.7,-2.942,-3.60291088309151E-16));
#88051=CARTESIAN_POINT('Ctrl Pts',(-3.1358238829104,-2.94290902102838,-0.00259068251834249));
#88052=CARTESIAN_POINT('Ctrl Pts',(-3.17798954720932,-2.93577329752197,
0.77600050829119));
#88053=CARTESIAN_POINT('Ctrl Pts',(-3.22015521150824,-2.61779276653383,
1.5597441706684));
#88054=CARTESIAN_POINT('Ctrl Pts',(-3.26232087580717,-2.06400928767338,
2.10320678247858));
#88055=CARTESIAN_POINT('Ctrl Pts',(-3.31516861047045,-1.36993265356056,
2.78434790490345));
#88056=CARTESIAN_POINT('Ctrl Pts',(-3.36801634513374,-0.305444837903283,
3.08804341587024));
#88057=CARTESIAN_POINT('Ctrl Pts',(-3.42086407979702,0.64355018528268,2.87566622534601));
#88058=CARTESIAN_POINT('Ctrl Pts',(-3.4737118144603,1.59254520846861,2.66328903482179));
#88059=CARTESIAN_POINT('Ctrl Pts',(-3.52655954912359,2.42604743918324,1.93483914280656));
#88060=CARTESIAN_POINT('Ctrl Pts',(-3.57940728378687,2.76359033593641,1.02283014731745));
#88061=CARTESIAN_POINT('Ctrl Pts',(-3.63225501845015,3.1011332326896,0.110821151828297));
#88062=CARTESIAN_POINT('Ctrl Pts',(-3.68510275311344,2.94271679548128,-0.984746947134762));
#88063=CARTESIAN_POINT('Ctrl Pts',(-3.73795048777672,2.36065294704176,-1.76378307655536));
#88064=CARTESIAN_POINT('Ctrl Pts',(-3.79079822244,1.77858909860226,-2.54281920597594));
#88065=CARTESIAN_POINT('Ctrl Pts',(-3.84364595710329,0.772877838931594,
-3.00532336585409));
#88066=CARTESIAN_POINT('Ctrl Pts',(-3.89649369176657,-0.197406467007782,
-2.94017750459693));
#88067=CARTESIAN_POINT('Ctrl Pts',(-3.94934142642986,-1.16769077294716,
-2.87503164333976));
#88068=CARTESIAN_POINT('Ctrl Pts',(-4.00218916109314,-2.10254812515524,
-2.28223576094729));
#88069=CARTESIAN_POINT('Ctrl Pts',(-4.05503689575642,-2.57524666212081,
-1.43238182693799));
#88070=CARTESIAN_POINT('Ctrl Pts',(-4.08196589147441,-2.81611407032574,
-0.999331799426508));
#88071=CARTESIAN_POINT('Ctrl Pts',(-4.1088948871924,-2.93698215328553,-0.499536766247084));
#88072=CARTESIAN_POINT('Ctrl Pts',(-4.1358238829104,-2.93721437885968,0.000152849678604627));
#88073=CARTESIAN_POINT('Ctrl Pts',(-4.2801761170896,-2.93720779641154,-5.3281763612922E-5));
#88074=CARTESIAN_POINT('Ctrl Pts',(-4.25392825029993,-2.93728669053742,
-0.487106598654287));
#88075=CARTESIAN_POINT('Ctrl Pts',(-4.22768038351026,-2.82276056857575,
-0.974125008385675));
#88076=CARTESIAN_POINT('Ctrl Pts',(-4.20143251672059,-2.59342404981643,
-1.39920104976605));
#88077=CARTESIAN_POINT('Ctrl Pts',(-4.14858478205731,-2.13167545938383,
-2.25505368063311));
#88078=CARTESIAN_POINT('Ctrl Pts',(-4.09573704739402,-1.20450590315705,
-2.85980294712179));
#88079=CARTESIAN_POINT('Ctrl Pts',(-4.04288931273074,-0.23513801698091,
-2.93740055033165));
#88080=CARTESIAN_POINT('Ctrl Pts',(-3.99004157806746,0.734229869195233,
-3.01499815354152));
#88081=CARTESIAN_POINT('Ctrl Pts',(-3.93719384340417,1.74579608532074,-2.56544409347258));
#88082=CARTESIAN_POINT('Ctrl Pts',(-3.88434610874089,2.33781367422211,-1.7939451234042));
#88083=CARTESIAN_POINT('Ctrl Pts',(-3.8314983740776,2.92983126312348,-1.02244615333581));
#88084=CARTESIAN_POINT('Ctrl Pts',(-3.77865063941432,3.10230022480071,0.0709977267320187));
#88085=CARTESIAN_POINT('Ctrl Pts',(-3.72580290475104,2.77649410964299,0.98726507943176));
#88086=CARTESIAN_POINT('Ctrl Pts',(-3.67295517008775,2.45068799448526,1.90353243213151));
#88087=CARTESIAN_POINT('Ctrl Pts',(-3.62010743542447,1.62660680249256,2.64262325746317));
#88088=CARTESIAN_POINT('Ctrl Pts',(-3.56725970076119,0.680416694159909,
2.86716672049554));
#88089=CARTESIAN_POINT('Ctrl Pts',(-3.5144119660979,-0.26577341417273,3.09171018352791));
#88090=CARTESIAN_POINT('Ctrl Pts',(-3.46156423143462,-1.33407243884532,
2.801706284261));
#88091=CARTESIAN_POINT('Ctrl Pts',(-3.40871649677134,-2.03683674323611,
2.12953233551788));
#88092=CARTESIAN_POINT('Ctrl Pts',(-3.36586970354409,-2.6066094502324,1.58456104435399));
#88093=CARTESIAN_POINT('Ctrl Pts',(-3.32302291031685,-2.93610497497431,
0.788377658866007));
#88094=CARTESIAN_POINT('Ctrl Pts',(-3.2801761170896,-2.94328604584299,-0.00252931999075325));
#88095=CARTESIAN_POINT('Origin',(-7.7,0.,0.));
#88096=CARTESIAN_POINT('',(-2.1358238829104,-2.94549590326081,0.00172726763101459));
#88097=CARTESIAN_POINT('',(-2.2801761170896,-2.94520044895666,0.00189243946321858));
#88098=CARTESIAN_POINT('',(-7.7,-2.942,-3.60291088309151E-16));
#88099=CARTESIAN_POINT('Ctrl Pts',(-2.1358238829104,-2.94549590326081,0.00172726763101459));
#88100=CARTESIAN_POINT('Ctrl Pts',(-2.14138873789967,-2.94621118435907,
0.104248158404311));
#88101=CARTESIAN_POINT('Ctrl Pts',(-2.14695359288894,-2.94132097000673,
0.206700038959149));
#88102=CARTESIAN_POINT('Ctrl Pts',(-2.15251844787821,-2.93059923639254,
0.308537962920288));
#88103=CARTESIAN_POINT('Ctrl Pts',(-2.20536618254149,-2.8287781944668,1.2756617414436));
#88104=CARTESIAN_POINT('Ctrl Pts',(-2.25821391720478,-2.20102858389113,
2.18741447546925));
#88105=CARTESIAN_POINT('Ctrl Pts',(-2.31106165186806,-1.33389435847118,
2.62761108458551));
#88106=CARTESIAN_POINT('Ctrl Pts',(-2.36390938653134,-0.466760133051231,
3.06780769370176));
#88107=CARTESIAN_POINT('Ctrl Pts',(-2.41675712119463,0.63975870721301,3.03644817790864));
#88108=CARTESIAN_POINT('Ctrl Pts',(-2.46960485585791,1.48057073115753,2.54784698609512));
#88109=CARTESIAN_POINT('Ctrl Pts',(-2.5224525905212,2.32138275510203,2.05924579428162));
#88110=CARTESIAN_POINT('Ctrl Pts',(-2.57530032518448,2.89648796272684,1.11340292644773));
#88111=CARTESIAN_POINT('Ctrl Pts',(-2.62814805984776,2.94337049059091,0.142064852598672));
#88112=CARTESIAN_POINT('Ctrl Pts',(-2.68099579451105,2.99025301845499,-0.829273221250395));
#88113=CARTESIAN_POINT('Ctrl Pts',(-2.73384352917433,2.50891286655834,-1.82610650111461));
#88114=CARTESIAN_POINT('Ctrl Pts',(-2.78669126383761,1.71906563566131,-2.39341317509171));
#88115=CARTESIAN_POINT('Ctrl Pts',(-2.8395389985009,0.929218404764276,-2.9607198490688));
#88116=CARTESIAN_POINT('Ctrl Pts',(-2.89238673316418,-0.169135905133138,
-3.09849991715875));
#88117=CARTESIAN_POINT('Ctrl Pts',(-2.94523446782747,-1.0746341620639,-2.74386125494763));
#88118=CARTESIAN_POINT('Ctrl Pts',(-2.99808220249075,-1.98013241899465,
-2.38922259273651));
#88119=CARTESIAN_POINT('Ctrl Pts',(-3.05092993715403,-2.69277462295876,
-1.54216520022432));
#88120=CARTESIAN_POINT('Ctrl Pts',(-3.10377767181732,-2.88726299865664,
-0.589343137026765));
#88121=CARTESIAN_POINT('Ctrl Pts',(-3.11445974218168,-2.92657477857477,
-0.396749975018218));
#88122=CARTESIAN_POINT('Ctrl Pts',(-3.12514181254604,-2.94471675492428,
-0.199835669015806));
#88123=CARTESIAN_POINT('Ctrl Pts',(-3.1358238829104,-2.94290902102838,-0.00259068251834249));
#88124=CARTESIAN_POINT('Ctrl Pts',(-3.2801761170896,-2.94328604584299,-0.00252931999075325));
#88125=CARTESIAN_POINT('Ctrl Pts',(-3.27017517565356,-2.94496219156584,
-0.187136236427897));
#88126=CARTESIAN_POINT('Ctrl Pts',(-3.26017423421752,-2.92907832148784,
-0.371455688921979));
#88127=CARTESIAN_POINT('Ctrl Pts',(-3.25017329278148,-2.89459120843848,
-0.552226040806602));
#88128=CARTESIAN_POINT('Ctrl Pts',(-3.1973255581182,-2.71235178514105,-1.50746647016865));
#88129=CARTESIAN_POINT('Ctrl Pts',(-3.14447782345492,-2.01064335443715,
-2.36360333067339));
#88130=CARTESIAN_POINT('Ctrl Pts',(-3.09163008879163,-1.10977289024573,
-2.72983809441704));
#88131=CARTESIAN_POINT('Ctrl Pts',(-3.03878235412835,-0.208902426054322,
-3.09607285816069));
#88132=CARTESIAN_POINT('Ctrl Pts',(-2.98593461946506,0.89113007162461,-2.97240552514326));
#88133=CARTESIAN_POINT('Ctrl Pts',(-2.93308688480178,1.68819564156411,-2.41528619309179));
#88134=CARTESIAN_POINT('Ctrl Pts',(-2.8802391501385,2.48526121150361,-1.85816686104031));
#88135=CARTESIAN_POINT('Ctrl Pts',(-2.82739141547522,2.97935985370367,-0.86759552995479));
#88136=CARTESIAN_POINT('Ctrl Pts',(-2.77454368081193,2.94495173425786,0.10426431795293));
#88137=CARTESIAN_POINT('Ctrl Pts',(-2.72169594614865,2.91054361481204,1.07612416586066));
#88138=CARTESIAN_POINT('Ctrl Pts',(-2.66884821148536,2.34762873372032,2.02927253059059));
#88139=CARTESIAN_POINT('Ctrl Pts',(-2.61600047682208,1.51315923045204,2.52862830825837));
#88140=CARTESIAN_POINT('Ctrl Pts',(-2.5631527421588,0.678689727183778,3.02798408592614));
#88141=CARTESIAN_POINT('Ctrl Pts',(-2.51030500749551,-0.427334398261043,
3.07354727653178));
#88142=CARTESIAN_POINT('Ctrl Pts',(-2.45745727283223,-1.30004899242779,
2.64451975108657));
#88143=CARTESIAN_POINT('Ctrl Pts',(-2.40460953816895,-2.17276358659452,
2.21549222564138));
#88144=CARTESIAN_POINT('Ctrl Pts',(-2.35176180350566,-2.81216864948318,
1.31187398414536));
#88145=CARTESIAN_POINT('Ctrl Pts',(-2.29891406884238,-2.92639711020017,
0.346137294326151));
#88146=CARTESIAN_POINT('Ctrl Pts',(-2.29266808492479,-2.93989757778153,
0.231998516729099));
#88147=CARTESIAN_POINT('Ctrl Pts',(-2.2864221010072,-2.94606212951774,0.116992039186075));
#88148=CARTESIAN_POINT('Ctrl Pts',(-2.2801761170896,-2.94520044895666,0.00189243946321858));
#88149=CARTESIAN_POINT('Origin',(-7.7,0.,0.));
#88150=CARTESIAN_POINT('',(-1.13582388291039,-2.93784718745393,0.00133151008673116));
#88151=CARTESIAN_POINT('',(-1.2801761170896,-2.93764836154578,0.0011528133628201));
#88152=CARTESIAN_POINT('',(-7.7,-2.942,-3.60291088309151E-16));
#88153=CARTESIAN_POINT('Ctrl Pts',(-1.13582388291039,-2.93784718745393,
0.00133151008673116));
#88154=CARTESIAN_POINT('Ctrl Pts',(-1.1576356632533,-2.93947473760419,0.405867522931662));
#88155=CARTESIAN_POINT('Ctrl Pts',(-1.1794474435962,-2.86160462622403,0.809791925226849));
#88156=CARTESIAN_POINT('Ctrl Pts',(-1.20125922393911,-2.70117913249261,
1.1777113598064));
#88157=CARTESIAN_POINT('Ctrl Pts',(-1.25410695860239,-2.31248440915232,
2.06914288673587));
#88158=CARTESIAN_POINT('Ctrl Pts',(-1.30695469326567,-1.43915341522439,
2.74920947561571));
#88159=CARTESIAN_POINT('Ctrl Pts',(-1.35980242792896,-0.479674863775861,
2.90749655167124));
#88160=CARTESIAN_POINT('Ctrl Pts',(-1.41265016259224,0.47980368767267,3.06578362772676));
#88161=CARTESIAN_POINT('Ctrl Pts',(-1.46549789725552,1.52542979664179,2.70229119095795));
#88162=CARTESIAN_POINT('Ctrl Pts',(-1.51834563191881,2.17982640754776,1.98293454354379));
#88163=CARTESIAN_POINT('Ctrl Pts',(-1.57119336658209,2.83422301845374,1.26357789612962));
#88164=CARTESIAN_POINT('Ctrl Pts',(-1.62404110124538,3.09739013129655,0.188357038070054));
#88165=CARTESIAN_POINT('Ctrl Pts',(-1.67688883590866,2.84924391347341,-0.751921077245129));
#88166=CARTESIAN_POINT('Ctrl Pts',(-1.72973657057194,2.60109769565026,-1.6921991925603));
#88167=CARTESIAN_POINT('Ctrl Pts',(-1.78258430523523,1.8416381471612,-2.49753456513111));
#88168=CARTESIAN_POINT('Ctrl Pts',(-1.83543203989851,0.917511068992977,
-2.80031983874035));
#88169=CARTESIAN_POINT('Ctrl Pts',(-1.88827977456179,-0.00661600917524305,
-3.10310511234959));
#88170=CARTESIAN_POINT('Ctrl Pts',(-1.94112750922508,-1.0954106170226,-2.90334028699726));
#88171=CARTESIAN_POINT('Ctrl Pts',(-1.99397524388836,-1.85186168430837,
-2.2922104628106));
#88172=CARTESIAN_POINT('Ctrl Pts',(-2.04125812356237,-2.52865861839909,
-1.74543247646309));
#88173=CARTESIAN_POINT('Ctrl Pts',(-2.08854100323638,-2.93941837740121,
-0.869361548133691));
#88174=CARTESIAN_POINT('Ctrl Pts',(-2.1358238829104,-2.94549590326081,0.00172726763101459));
#88175=CARTESIAN_POINT('Ctrl Pts',(-2.2801761170896,-2.94520044895666,0.00189243946321858));
#88176=CARTESIAN_POINT('Ctrl Pts',(-2.23357436634391,-2.93877138617659,
-0.856874238130207));
#88177=CARTESIAN_POINT('Ctrl Pts',(-2.18697261559822,-2.54120861453645,
-1.72082480689521));
#88178=CARTESIAN_POINT('Ctrl Pts',(-2.14037086485253,-1.88113620379347,
-2.26824587484884));
#88179=CARTESIAN_POINT('Ctrl Pts',(-2.08752313018924,-1.13259497812453,
-2.88903721606212));
#88180=CARTESIAN_POINT('Ctrl Pts',(-2.03467539552596,-0.0464606682413524,
-3.10276476034627));
#88181=CARTESIAN_POINT('Ctrl Pts',(-1.98182766086268,0.881480161163561,
-2.81186872231317));
#88182=CARTESIAN_POINT('Ctrl Pts',(-1.92897992619939,1.80942099056847,-2.52097268428006));
#88183=CARTESIAN_POINT('Ctrl Pts',(-1.87613219153611,2.57916833949514,-1.72545306392968));
#88184=CARTESIAN_POINT('Ctrl Pts',(-1.82328445687283,2.83936093304215,-0.788438863463607));
#88185=CARTESIAN_POINT('Ctrl Pts',(-1.77043672220954,3.09955352658915,0.148575337002482));
#88186=CARTESIAN_POINT('Ctrl Pts',(-1.71758898754626,2.8501913647565,1.22708411758425));
#88187=CARTESIAN_POINT('Ctrl Pts',(-1.66474125288298,2.20509390103984,1.95478393112635));
#88188=CARTESIAN_POINT('Ctrl Pts',(-1.61189351821969,1.55999643732318,2.68248374466846));
#88189=CARTESIAN_POINT('Ctrl Pts',(-1.55904578355641,0.519163671722485,
3.05937459117085));
#88190=CARTESIAN_POINT('Ctrl Pts',(-1.50619804889312,-0.442286305680839,
2.91341713798924));
#88191=CARTESIAN_POINT('Ctrl Pts',(-1.45335031422984,-1.40373628308415,
2.76745968480763));
#88192=CARTESIAN_POINT('Ctrl Pts',(-1.40050257956656,-2.28580347229011,
2.09865393194203));
#88193=CARTESIAN_POINT('Ctrl Pts',(-1.34765484490327,-2.68587574865743,
1.21228971570189));
#88194=CARTESIAN_POINT('Ctrl Pts',(-1.32516193563205,-2.8561534241642,0.835037785715198));
#88195=CARTESIAN_POINT('Ctrl Pts',(-1.30266902636083,-2.93911768646335,
0.418375124404466));
#88196=CARTESIAN_POINT('Ctrl Pts',(-1.2801761170896,-2.93764836154578,0.0011528133628201));
#88197=CARTESIAN_POINT('Origin',(-7.7,0.,0.));
#88198=CARTESIAN_POINT('',(-0.249999999999999,-2.942,-3.60291088309151E-16));
#88199=CARTESIAN_POINT('',(-0.2801761170896,-2.94174543957041,-0.0025773274983063));
#88200=CARTESIAN_POINT('',(-7.7,-2.942,-3.60291088309151E-16));
#88201=CARTESIAN_POINT('',(-0.250000000000001,-2.21686865784453,1.93412961144453));
#88202=CARTESIAN_POINT('Origin',(-0.25,0.,0.));
#88203=CARTESIAN_POINT('Ctrl Pts',(-0.250000000000001,-2.21686865784453,
1.93412961144453));
#88204=CARTESIAN_POINT('Ctrl Pts',(-0.302847734663285,-1.57463683943972,
2.67024552677286));
#88205=CARTESIAN_POINT('Ctrl Pts',(-0.355695469326569,-0.542559076580902,
3.05509500507822));
#88206=CARTESIAN_POINT('Ctrl Pts',(-0.408543203989852,0.418376638715716,
2.91670525910205));
#88207=CARTESIAN_POINT('Ctrl Pts',(-0.461390938653135,1.37931235401231,
2.77831551312588));
#88208=CARTESIAN_POINT('Ctrl Pts',(-0.514238673316417,2.2691060217467,2.1166865428682));
#88209=CARTESIAN_POINT('Ctrl Pts',(-0.5670864079797,2.67678709245509,1.23355235122458));
#88210=CARTESIAN_POINT('Ctrl Pts',(-0.619934142642985,3.08446816316349,
0.350418159580932));
#88211=CARTESIAN_POINT('Ctrl Pts',(-0.672781877306269,3.01003663684585,
-0.754221253448677));
#88212=CARTESIAN_POINT('Ctrl Pts',(-0.725629611969553,2.48967051684404,
-1.57596292656688));
#88213=CARTESIAN_POINT('Ctrl Pts',(-0.778477346632837,1.96930439684224,
-2.39770459968508));
#88214=CARTESIAN_POINT('Ctrl Pts',(-0.831325081296121,1.00300368315625,
-2.93654853289187));
#88215=CARTESIAN_POINT('Ctrl Pts',(-0.884172815959405,0.0307377045118488,
-2.94662393799235));
#88216=CARTESIAN_POINT('Ctrl Pts',(-0.93702055062269,-0.941528274132556,
-2.95669934309284));
#88217=CARTESIAN_POINT('Ctrl Pts',(-0.989868285285974,-1.91975951773539,
-2.43800622008702));
#88218=CARTESIAN_POINT('Ctrl Pts',(-1.04271601994926,-2.45684591316047,
-1.62726142609455));
#88219=CARTESIAN_POINT('Ctrl Pts',(-1.07375197426964,-2.77226130306725,
-1.15113433091906));
#88220=CARTESIAN_POINT('Ctrl Pts',(-1.10478792859001,-2.93553134842917,
-0.574282264590201));
#88221=CARTESIAN_POINT('Ctrl Pts',(-1.13582388291039,-2.93784718745393,
0.00133151008673116));
#88222=CARTESIAN_POINT('Ctrl Pts',(-1.2801761170896,-2.93764836154578,0.0011528133628201));
#88223=CARTESIAN_POINT('Ctrl Pts',(-1.24982129169754,-2.93566546547934,
-0.561900647113437));
#88224=CARTESIAN_POINT('Ctrl Pts',(-1.21946646630548,-2.77990979285944,
-1.12597335710706));
#88225=CARTESIAN_POINT('Ctrl Pts',(-1.18911164091342,-2.47745937646832,
-1.59557717601159));
#88226=CARTESIAN_POINT('Ctrl Pts',(-1.13626390625014,-1.95089336438317,
-2.41315717187029));
#88227=CARTESIAN_POINT('Ctrl Pts',(-1.08341617158686,-0.97968397668418,
-2.94439448397298));
#88228=CARTESIAN_POINT('Ctrl Pts',(-1.03056843692357,-0.00723965287597085,
-2.94678989518399));
#88229=CARTESIAN_POINT('Ctrl Pts',(-0.977720702260289,0.965204670932211,
-2.94918530639499));
#88230=CARTESIAN_POINT('Ctrl Pts',(-0.924872967597005,1.93888393084963,
-2.4227388167143));
#88231=CARTESIAN_POINT('Ctrl Pts',(-0.872025232933722,2.46950402838423,
-1.60776891670247));
#88232=CARTESIAN_POINT('Ctrl Pts',(-0.819177498270439,3.00012412591883,
-0.792799016690619));
#88233=CARTESIAN_POINT('Ctrl Pts',(-0.766329763607154,3.08768506107063,
0.310694293652399));
#88234=CARTESIAN_POINT('Ctrl Pts',(-0.71348202894387,2.69191482003378,1.19902692584877));
#88235=CARTESIAN_POINT('Ctrl Pts',(-0.660634294280585,2.29614457899693,
2.08735955804518));
#88236=CARTESIAN_POINT('Ctrl Pts',(-0.607786559617304,1.41704316177144,
2.76053151209489));
#88237=CARTESIAN_POINT('Ctrl Pts',(-0.554938824954019,0.456472030616278,
2.91121453806236));
#88238=CARTESIAN_POINT('Ctrl Pts',(-0.502091090290737,-0.504099100538845,
3.06189756402983));
#88239=CARTESIAN_POINT('Ctrl Pts',(-0.449243355627451,-1.54613994562364,
2.69009166191506));
#88240=CARTESIAN_POINT('Ctrl Pts',(-0.396395620964168,-2.19510946333902,
1.96560658123782));
#88241=CARTESIAN_POINT('Ctrl Pts',(-0.357655786339312,-2.67083414582638,
1.43452549720582));
#88242=CARTESIAN_POINT('Ctrl Pts',(-0.318915951714456,-2.93533926593172,
0.713929847825713));
#88243=CARTESIAN_POINT('Ctrl Pts',(-0.2801761170896,-2.94174543957041,-0.0025773274983063));
#88244=CARTESIAN_POINT('Origin',(-17.306589891905,0.,0.));
#88245=CARTESIAN_POINT('',(-0.806589891905004,-2.36840213013048,0.00107342251797217));
#88246=CARTESIAN_POINT('',(-0.609410108094966,-2.37154478120365,-0.00207776223488526));
#88247=CARTESIAN_POINT('',(-17.306589891905,-2.37175,-2.3095687792789E-13));
#88248=CARTESIAN_POINT('',(-0.25,2.22665730523966,0.827839780511538));
#88249=CARTESIAN_POINT('Ctrl Pts',(-0.806589891905004,-2.36840213013048,
0.00107342251797246));
#88250=CARTESIAN_POINT('Ctrl Pts',(-0.775553937584626,-2.3665351718684,
-0.462968715513973));
#88251=CARTESIAN_POINT('Ctrl Pts',(-0.691670248600965,-2.01078495654127,
-1.71987561692049));
#88252=CARTESIAN_POINT('Ctrl Pts',(-0.55493882495402,0.029588806200308,
-2.80175461640703));
#88253=CARTESIAN_POINT('Ctrl Pts',(-0.400444815306063,2.30690749425437,
-1.5318400425519));
#88254=CARTESIAN_POINT('Ctrl Pts',(-0.29879854032139,2.47529789451049,0.147370939433083));
#88255=CARTESIAN_POINT('Ctrl Pts',(-0.25,2.22665730523966,0.827839780511538));
#88256=CARTESIAN_POINT('',(-0.250000000000001,1.50502666328431,-1.8330555925294));
#88257=CARTESIAN_POINT('Origin',(-0.249999999999999,0.,0.));
#88258=CARTESIAN_POINT('Ctrl Pts',(-0.609410108094966,-2.37154478120365,
-0.00207776223488519));
#88259=CARTESIAN_POINT('Ctrl Pts',(-0.595302208056545,-2.37342552465464,
-0.21243206319483));
#88260=CARTESIAN_POINT('Ctrl Pts',(-0.52834657335484,-2.25138912390084,
-1.20869219511272));
#88261=CARTESIAN_POINT('Ctrl Pts',(-0.408543203989851,-0.847344309994932,
-2.66988130255231));
#88262=CARTESIAN_POINT('Ctrl Pts',(-0.302847734663285,0.896356686121819,
-2.33280287161008));
#88263=CARTESIAN_POINT('Ctrl Pts',(-0.250000000000001,1.50502666328431,
-1.8330555925294));
#88264=CARTESIAN_POINT('Origin',(-17.306589891905,0.,0.));
#88265=CARTESIAN_POINT('',(-1.80658989190501,-2.37456828978886,0.00139247008960864));
#88266=CARTESIAN_POINT('',(-1.60941010809497,-2.36824184279273,0.000929362709871234));
#88267=CARTESIAN_POINT('',(-17.306589891905,-2.37175,-2.3095687792789E-13));
#88268=CARTESIAN_POINT('Ctrl Pts',(-1.80658989190501,-2.37456828978886,
0.00139247008960867));
#88269=CARTESIAN_POINT('Ctrl Pts',(-1.759307012231,-2.36966877518737,-0.700852566888605));
#88270=CARTESIAN_POINT('Ctrl Pts',(-1.6591763978937,-1.66841196255505,-2.19649738938181));
#88271=CARTESIAN_POINT('Ctrl Pts',(-1.50619804889313,0.872419133718849,
-2.66267225518167));
#88272=CARTESIAN_POINT('Ctrl Pts',(-1.34765484490327,2.70917798905082,-0.714962360659344));
#88273=CARTESIAN_POINT('Ctrl Pts',(-1.18911164091343,2.07270626924971,1.88546769043105));
#88274=CARTESIAN_POINT('Ctrl Pts',(-1.03056843692357,-0.456148649799437,
2.76457699047157));
#88275=CARTESIAN_POINT('Ctrl Pts',(-0.903061187254099,-2.15483664022398,
1.44180137017275));
#88276=CARTESIAN_POINT('Ctrl Pts',(-0.82840167224791,-2.36971421105125,
0.327197925735182));
#88277=CARTESIAN_POINT('Ctrl Pts',(-0.806589891905004,-2.36840213013048,
0.00107342251797246));
#88278=CARTESIAN_POINT('Ctrl Pts',(-1.60941010809497,-2.36824184279273,
0.0009293627098712));
#88279=CARTESIAN_POINT('Ctrl Pts',(-1.57905528270292,-2.36664329291314,
-0.452987035959174));
#88280=CARTESIAN_POINT('Ctrl Pts',(-1.49585272264758,-2.02246849688374,
-1.69942388568812));
#88281=CARTESIAN_POINT('Ctrl Pts',(-1.35980242792896,-0.0068319532377577,
-2.80194755688051));
#88282=CARTESIAN_POINT('Ctrl Pts',(-1.20125922393911,2.34801894891291,-1.52873260592859));
#88283=CARTESIAN_POINT('Ctrl Pts',(-1.04271601994925,2.55978575511233,1.14007459203818));
#88284=CARTESIAN_POINT('Ctrl Pts',(-0.884172815959405,0.433672104903693,
2.76814622563851));
#88285=CARTESIAN_POINT('Ctrl Pts',(-0.739737512007974,-1.86225432289822,
1.94894705441156));
#88286=CARTESIAN_POINT('Ctrl Pts',(-0.648149942719829,-2.36638032086125,
0.575548306111478));
#88287=CARTESIAN_POINT('Ctrl Pts',(-0.609410108094966,-2.37154478120365,
-0.00207776223488519));
#88288=CARTESIAN_POINT('Origin',(-17.306589891905,0.,0.));
#88289=CARTESIAN_POINT('',(-2.80658989190501,-2.37248282482123,-0.00208852864143664));
#88290=CARTESIAN_POINT('',(-2.60941010809497,-2.3743301036074,0.00152562654522952));
#88291=CARTESIAN_POINT('',(-17.306589891905,-2.37175,-2.3095687792789E-13));
#88292=CARTESIAN_POINT('Ctrl Pts',(-2.80658989190501,-2.37248282482123,
-0.00208852864143679));
#88293=CARTESIAN_POINT('Ctrl Pts',(-2.79590782154065,-2.37394016434114,
-0.161101375930807));
#88294=CARTESIAN_POINT('Ctrl Pts',(-2.73237801651301,-2.28695745611499,
-1.10521789855147));
#88295=CARTESIAN_POINT('Ctrl Pts',(-2.61600047682208,-1.02181166468338,
-2.60898948164979));
#88296=CARTESIAN_POINT('Ctrl Pts',(-2.45745727283223,1.63456682052989,-2.27576730983566));
#88297=CARTESIAN_POINT('Ctrl Pts',(-2.29891406884238,2.79869174091825,0.135081770570203));
#88298=CARTESIAN_POINT('Ctrl Pts',(-2.14037086485253,1.40779530021379,2.42261014084723));
#88299=CARTESIAN_POINT('Ctrl Pts',(-1.98182766086268,-1.26832916552041,
2.49845337495562));
#88300=CARTESIAN_POINT('Ctrl Pts',(-1.87056733654684,-2.33376337820802,
0.951001110586071));
#88301=CARTESIAN_POINT('Ctrl Pts',(-1.81215474689428,-2.37514492743155,
0.0840416620310201));
#88302=CARTESIAN_POINT('Ctrl Pts',(-1.80658989190501,-2.37456828978886,
0.00139247008960867));
#88303=CARTESIAN_POINT('Ctrl Pts',(-2.60941010809497,-2.3743301036074,0.00152562654522945));
#88304=CARTESIAN_POINT('Ctrl Pts',(-2.56280835734929,-2.36914719074238,
-0.690785681266458));
#88305=CARTESIAN_POINT('Ctrl Pts',(-2.46335887194031,-1.68518474265676,
-2.17711636459373));
#88306=CARTESIAN_POINT('Ctrl Pts',(-2.31106165186806,0.838152943427643,
-2.67365418881957));
#88307=CARTESIAN_POINT('Ctrl Pts',(-2.15251844787821,2.69979292454605,-0.749683767780105));
#88308=CARTESIAN_POINT('Ctrl Pts',(-1.99397524388836,2.09670858668745,1.85869814963478));
#88309=CARTESIAN_POINT('Ctrl Pts',(-1.83543203989851,-0.420553593951653,
2.77021160836216));
#88310=CARTESIAN_POINT('Ctrl Pts',(-1.70724366130071,-2.14539904246319,
1.46238996746531));
#88311=CARTESIAN_POINT('Ctrl Pts',(-1.6319030173662,-2.36942636739278,0.337281169716417));
#88312=CARTESIAN_POINT('Ctrl Pts',(-1.60941010809497,-2.36824184279273,
0.0009293627098712));
#88313=CARTESIAN_POINT('Origin',(-17.306589891905,0.,0.));
#88314=CARTESIAN_POINT('',(-3.80658989190501,-2.36789197928635,0.000123222714106244));
#88315=CARTESIAN_POINT('',(-3.60941010809497,-2.37278677064178,-0.00203906005744159));
#88316=CARTESIAN_POINT('',(-17.306589891905,-2.37175,-2.3095687792789E-13));
#88317=CARTESIAN_POINT('Ctrl Pts',(-3.80658989190501,-2.36789197928635,
0.000123222714106461));
#88318=CARTESIAN_POINT('Ctrl Pts',(-3.77966089618702,-2.36770476616414,
-0.402711191484291));
#88319=CARTESIAN_POINT('Ctrl Pts',(-3.69988416580574,-2.07903988532791,
-1.59635363341212));
#88320=CARTESIAN_POINT('Ctrl Pts',(-3.56725970076119,-0.187703149434983,
-2.79565599393456));
#88321=CARTESIAN_POINT('Ctrl Pts',(-3.40871649677134,2.24461739453909,-1.67708606749907));
#88322=CARTESIAN_POINT('Ctrl Pts',(-3.25017329278149,2.6277487863971,0.972553944787357));
#88323=CARTESIAN_POINT('Ctrl Pts',(-3.09163008879163,0.611917125250802,
2.73431570350978));
#88324=CARTESIAN_POINT('Ctrl Pts',(-2.94376895516614,-1.78909631603478,
2.0493130260116));
#88325=CARTESIAN_POINT('Ctrl Pts',(-2.84875555620393,-2.36673022379259,
0.625587765309121));
#88326=CARTESIAN_POINT('Ctrl Pts',(-2.80658989190501,-2.37248282482123,
-0.00208852864143679));
#88327=CARTESIAN_POINT('Ctrl Pts',(-3.60941010809497,-2.37278677064178,
-0.0020390600574414));
#88328=CARTESIAN_POINT('Ctrl Pts',(-3.59940916665894,-2.37413802781993,
-0.15086348359909));
#88329=CARTESIAN_POINT('Ctrl Pts',(-3.53656049055962,-2.29366732089097,
-1.08466088751338));
#88330=CARTESIAN_POINT('Ctrl Pts',(-3.42086407979702,-1.05522311535154,
-2.59565560789489));
#88331=CARTESIAN_POINT('Ctrl Pts',(-3.26232087580717,1.60521408013114,-2.29656519618435));
#88332=CARTESIAN_POINT('Ctrl Pts',(-3.10377767181731,2.80019550906176,0.0991393121454807));
#88333=CARTESIAN_POINT('Ctrl Pts',(-2.94523446782747,1.43878146837926,2.40433608377855));
#88334=CARTESIAN_POINT('Ctrl Pts',(-2.78669126383761,-1.23614652569664,
2.51453101646264));
#88335=CARTESIAN_POINT('Ctrl Pts',(-2.67474981059345,-2.32800632564574,
0.971495952065517));
#88336=CARTESIAN_POINT('Ctrl Pts',(-2.61565609201257,-2.37502476399855,
0.0943153871308459));
#88337=CARTESIAN_POINT('Ctrl Pts',(-2.60941010809497,-2.3743301036074,0.00152562654522945));
#88338=CARTESIAN_POINT('Origin',(-17.306589891905,0.,0.));
#88339=CARTESIAN_POINT('',(-4.80658989190501,-2.37293245461563,0.00201017445689671));
#88340=CARTESIAN_POINT('',(-4.60941010809497,-2.36788667271892,-4.29541209298612E-5));
#88341=CARTESIAN_POINT('',(-17.306589891905,-2.37175,-2.3095687792789E-13));
#88342=CARTESIAN_POINT('Ctrl Pts',(-4.80658989190501,-2.37293245461563,
0.00201017445689676));
#88343=CARTESIAN_POINT('Ctrl Pts',(-4.76341397083339,-2.36713986096666,
-0.640390818759947));
#88344=CARTESIAN_POINT('Ctrl Pts',(-4.66739031509848,-1.76624041701385,
-2.07864193942938));
#88345=CARTESIAN_POINT('Ctrl Pts',(-4.51851892470029,0.663872292187274,
-2.72216797540702));
#88346=CARTESIAN_POINT('Ctrl Pts',(-4.35997572071044,2.64579147695974,-0.922340700408471));
#88347=CARTESIAN_POINT('Ctrl Pts',(-4.20143251672059,2.21227577950313,1.71952341690803));
#88348=CARTESIAN_POINT('Ctrl Pts',(-4.04288931273074,-0.24090327052083,
2.79157491766907));
#88349=CARTESIAN_POINT('Ctrl Pts',(-3.91127510445888,-2.09482974284144,
1.56588393431461));
#88350=CARTESIAN_POINT('Ctrl Pts',(-3.8325086308503,-2.36807216900053,0.387845072022191));
#88351=CARTESIAN_POINT('Ctrl Pts',(-3.80658989190501,-2.36789197928635,
0.000123222714106461));
#88352=CARTESIAN_POINT('Ctrl Pts',(-4.60941010809497,-2.36788667271892,
-4.29541209298265E-5));
#88353=CARTESIAN_POINT('Ctrl Pts',(-4.58316224130531,-2.36795027473895,
-0.392690372317799));
#88354=CARTESIAN_POINT('Ctrl Pts',(-4.50406663985236,-2.08972978198754,
-1.57581348531183));
#88355=CARTESIAN_POINT('Ctrl Pts',(-4.37212330373612,-0.223580041071285,
-2.79301553794379));
#88356=CARTESIAN_POINT('Ctrl Pts',(-4.21358009974628,2.22290076086175,-1.70576552913832));
#88357=CARTESIAN_POINT('Ctrl Pts',(-4.05503689575642,2.64001829300782,0.938737043143364));
#88358=CARTESIAN_POINT('Ctrl Pts',(-3.89649369176657,0.646971487662433,
2.7262339822803));
#88359=CARTESIAN_POINT('Ctrl Pts',(-3.74795142921276,-1.77373833013654,
2.06910028661809));
#88360=CARTESIAN_POINT('Ctrl Pts',(-3.65225690132222,-2.36699761196315,
0.63556584378477));
#88361=CARTESIAN_POINT('Ctrl Pts',(-3.60941010809497,-2.37278677064178,
-0.0020390600574414));
#88362=CARTESIAN_POINT('Origin',(-17.306589891905,0.,0.));
#88363=CARTESIAN_POINT('',(-5.80658989190502,-2.37420921644579,-0.00158594309364022));
#88364=CARTESIAN_POINT('',(-5.60941010809497,-2.37263003492395,0.00206636748989852));
#88365=CARTESIAN_POINT('',(-17.306589891905,-2.37175,-2.3095687792789E-13));
#88366=CARTESIAN_POINT('Ctrl Pts',(-5.80658989190502,-2.37420921644579,
-0.00158594309364031));
#88367=CARTESIAN_POINT('Ctrl Pts',(-5.80001478014305,-2.37496212800069,
-0.0992782592791646));
#88368=CARTESIAN_POINT('Ctrl Pts',(-5.74059193371779,-2.32517322677813,
-0.981403206808898));
#88369=CARTESIAN_POINT('Ctrl Pts',(-5.62832135262924,-1.2205227666753,-2.52215167718616));
#88370=CARTESIAN_POINT('Ctrl Pts',(-5.4697781486394,1.45366996224847,-2.39536396974682));
#88371=CARTESIAN_POINT('Ctrl Pts',(-5.31123494464955,2.8007569218186,-0.0817653447559351));
#88372=CARTESIAN_POINT('Ctrl Pts',(-5.15269174065969,1.59093566559739,2.30647970175859));
#88373=CARTESIAN_POINT('Ctrl Pts',(-4.99414853666984,-1.07130598541964,
2.58905936438303));
#88374=CARTESIAN_POINT('Ctrl Pts',(-4.87878125375162,-2.29685610505972,
1.07473064721425));
#88375=CARTESIAN_POINT('Ctrl Pts',(-4.81626170549667,-2.37423005023362,
0.145914056604193));
#88376=CARTESIAN_POINT('Ctrl Pts',(-4.80658989190501,-2.37293245461563,
0.00201017445689676));
#88377=CARTESIAN_POINT('Ctrl Pts',(-5.60941010809497,-2.37263003492395,
0.00206636748989856));
#88378=CARTESIAN_POINT('Ctrl Pts',(-5.56691531595168,-2.36685493862076,
-0.630408109289954));
#88379=CARTESIAN_POINT('Ctrl Pts',(-5.4715727891451,-1.78170188936919,-2.05888119862122));
#88380=CARTESIAN_POINT('Ctrl Pts',(-5.32338252767523,0.628868639624235,
-2.73046663851582));
#88381=CARTESIAN_POINT('Ctrl Pts',(-5.16483932368538,2.63373164752747,-0.956232941728888));
#88382=CARTESIAN_POINT('Ctrl Pts',(-5.00629611969553,2.23416961039886,1.6909790010008));
#88383=CARTESIAN_POINT('Ctrl Pts',(-4.84775291570567,-0.205043418049532,
2.79443751524972));
#88384=CARTESIAN_POINT('Ctrl Pts',(-4.71545757850549,-2.08422822423836,
1.58643001607205));
#88385=CARTESIAN_POINT('Ctrl Pts',(-4.63600997596859,-2.36782221775416,
0.397870123107349));
#88386=CARTESIAN_POINT('Ctrl Pts',(-4.60941010809497,-2.36788667271892,
-4.29541209298265E-5));
#88387=CARTESIAN_POINT('Origin',(-17.306589891905,0.,0.));
#88388=CARTESIAN_POINT('',(-6.80658989190501,-2.36818083915218,-0.0008555996482021));
#88389=CARTESIAN_POINT('',(-6.60941010809497,-2.37445554261321,-0.00145817468174603));
#88390=CARTESIAN_POINT('',(-17.306589891905,-2.37175,-2.3095687792789E-13));
#88391=CARTESIAN_POINT('Ctrl Pts',(-6.80658989190501,-2.36818083915218,
-0.00085559964820188));
#88392=CARTESIAN_POINT('Ctrl Pts',(-6.78376785478941,-2.36929017234292,
-0.342149481798462));
#88393=CARTESIAN_POINT('Ctrl Pts',(-6.70809808301052,-2.14074935415041,
-1.47234264798851));
#88394=CARTESIAN_POINT('Ctrl Pts',(-6.57958057656835,-0.403348751247113,
-2.77276661325373));
#88395=CARTESIAN_POINT('Ctrl Pts',(-6.42103737257851,2.10819389270592,-1.84565528132004));
#88396=CARTESIAN_POINT('Ctrl Pts',(-6.26249416858865,2.69509315088937,0.766418824623061));
#88397=CARTESIAN_POINT('Ctrl Pts',(-6.1039509645988,0.821548317644948,2.6788025810951));
#88398=CARTESIAN_POINT('Ctrl Pts',(-5.95198287237092,-1.69321188063458,
2.16772687694675));
#88399=CARTESIAN_POINT('Ctrl Pts',(-5.85286251480633,-2.36891057001675,
0.685927801289234));
#88400=CARTESIAN_POINT('Ctrl Pts',(-5.80658989190502,-2.37420921644579,
-0.00158594309364031));
#88401=CARTESIAN_POINT('Ctrl Pts',(-6.60941010809497,-2.37445554261321,
-0.00145817468174572));
#88402=CARTESIAN_POINT('Ctrl Pts',(-6.60351612526133,-2.37508875977735,
-0.0890065105479783));
#88403=CARTESIAN_POINT('Ctrl Pts',(-6.5447744077644,-2.33100010852313,-0.960902990558076));
#88404=CARTESIAN_POINT('Ctrl Pts',(-6.43318495560419,-1.2528030468829,-2.50627379902584));
#88405=CARTESIAN_POINT('Ctrl Pts',(-6.27464175161433,1.42279687533745,-2.41382950547303));
#88406=CARTESIAN_POINT('Ctrl Pts',(-6.11609854762448,2.79947614093066,-0.117716465815816));
#88407=CARTESIAN_POINT('Ctrl Pts',(-5.95755534363463,1.62041646007026,2.285864021742));
#88408=CARTESIAN_POINT('Ctrl Pts',(-5.79901213964478,-1.0379776562294,2.60259989532173));
#88409=CARTESIAN_POINT('Ctrl Pts',(-5.68296372779822,-2.2902184224173,1.09528349834256));
#88410=CARTESIAN_POINT('Ctrl Pts',(-5.61976305061496,-2.37403701298076,
0.156155176334485));
#88411=CARTESIAN_POINT('Ctrl Pts',(-5.60941010809497,-2.37263003492395,
0.00206636748989856));
#88412=CARTESIAN_POINT('Origin',(-17.306589891905,0.,0.));
#88413=CARTESIAN_POINT('',(-7.80658989190501,-2.37109816127964,0.00213708253619841));
#88414=CARTESIAN_POINT('',(-7.60941010809498,-2.36830089438249,-0.00100592404030236));
#88415=CARTESIAN_POINT('',(-17.306589891905,-2.37175,-2.3095687792789E-13));
#88416=CARTESIAN_POINT('Ctrl Pts',(-7.80658989190501,-2.37109816127964,
0.0021370825361984));
#88417=CARTESIAN_POINT('Ctrl Pts',(-7.76752092943578,-2.36593601989977,
-0.580311471015131));
#88418=CARTESIAN_POINT('Ctrl Pts',(-7.67560423230326,-1.85624009305816,
-1.9587052675019));
#88419=CARTESIAN_POINT('Ctrl Pts',(-7.53083980050746,0.451359570691226,
-2.76535701938333));
#88420=CARTESIAN_POINT('Ctrl Pts',(-7.37229659651761,2.56653624207177,-1.1241959904035));
#88421=CARTESIAN_POINT('Ctrl Pts',(-7.21375339252775,2.33863288664257,1.54328258210251));
#88422=CARTESIAN_POINT('Ctrl Pts',(-7.05521018853791,-0.0242896112824878,
2.80184491388995));
#88423=CARTESIAN_POINT('Ctrl Pts',(-6.91948902166366,-2.02809044884209,
1.68954352771679));
#88424=CARTESIAN_POINT('Ctrl Pts',(-6.83661558945269,-2.36672135055807,
0.448165967901147));
#88425=CARTESIAN_POINT('Ctrl Pts',(-6.80658989190501,-2.36818083915218,
-0.00085559964820188));
#88426=CARTESIAN_POINT('Ctrl Pts',(-7.60941010809498,-2.36830089438249,
-0.00100592404030229));
#88427=CARTESIAN_POINT('Ctrl Pts',(-7.5872691999077,-2.36956993952812,-0.332071764583063));
#88428=CARTESIAN_POINT('Ctrl Pts',(-7.51228055705713,-2.15035683272869,
-1.45174667900709));
#88429=CARTESIAN_POINT('Ctrl Pts',(-7.38444417954329,-0.438913988766854,
-2.76735945269628));
#88430=CARTESIAN_POINT('Ctrl Pts',(-7.22590097555344,2.08432431928549,-1.87256934771392));
#88431=CARTESIAN_POINT('Ctrl Pts',(-7.06735777156358,2.70471060372122,0.731754316748925));
#88432=CARTESIAN_POINT('Ctrl Pts',(-6.90881456757374,0.855872690191172,
2.66803406427797));
#88433=CARTESIAN_POINT('Ctrl Pts',(-6.75616534641753,-1.67654134756637,
2.18714080723266));
#88434=CARTESIAN_POINT('Ctrl Pts',(-6.65636385992461,-2.36941108924122,
0.695985803589395));
#88435=CARTESIAN_POINT('Ctrl Pts',(-6.60941010809497,-2.37445554261321,
-0.00145817468174572));
#88436=CARTESIAN_POINT('Origin',(-17.306589891905,0.,0.));
#88437=CARTESIAN_POINT('',(-8.80658989190501,-2.37538658813648,-0.000666706255725389));
#88438=CARTESIAN_POINT('',(-8.60941010809498,-2.37080369071248,0.00210958135937009));
#88439=CARTESIAN_POINT('',(-17.306589891905,-2.37175,-2.3095687792789E-13));
#88440=CARTESIAN_POINT('Ctrl Pts',(-8.80658989190501,-2.37538658813648,
-0.000666706255725148));
#88441=CARTESIAN_POINT('Ctrl Pts',(-8.80412173874543,-2.37552348369093,
-0.0372902868490661));
#88442=CARTESIAN_POINT('Ctrl Pts',(-8.74880585092257,-2.35817895798474,
-0.857960161496038));
#88443=CARTESIAN_POINT('Ctrl Pts',(-8.64064222843641,-1.41192306630101,
-2.42020622293936));
#88444=CARTESIAN_POINT('Ctrl Pts',(-8.48209902444656,1.26406585736851,-2.50061240797977));
#88445=CARTESIAN_POINT('Ctrl Pts',(-8.32355582045671,2.78604518069765,-0.298122722747819));
#88446=CARTESIAN_POINT('Ctrl Pts',(-8.16501261646686,1.76454714739586,2.17653354472756));
#88447=CARTESIAN_POINT('Ctrl Pts',(-8.00646941247701,-0.867867228973001,
2.66415678584837));
#88448=CARTESIAN_POINT('Ctrl Pts',(-7.88699517095639,-2.25452734930914,
1.19877087178493));
#88449=CARTESIAN_POINT('Ctrl Pts',(-7.82036866409906,-2.37291873611991,
0.207554002436673));
#88450=CARTESIAN_POINT('Ctrl Pts',(-7.80658989190501,-2.37109816127964,
0.0021370825361984));
#88451=CARTESIAN_POINT('Ctrl Pts',(-8.60941010809498,-2.37080369071248,
0.00210958135936995));
#88452=CARTESIAN_POINT('Ctrl Pts',(-8.57102227455407,-2.36584710075431,
-0.570365230392202));
#88453=CARTESIAN_POINT('Ctrl Pts',(-8.47978670634988,-1.87042622880759,
-1.93864657712568));
#88454=CARTESIAN_POINT('Ctrl Pts',(-8.33570340348239,0.415818959741428,
-2.77092374898376));
#88455=CARTESIAN_POINT('Ctrl Pts',(-8.17716019949255,2.55189140603955,-1.15705405307796));
#88456=CARTESIAN_POINT('Ctrl Pts',(-8.0186169955027,2.35825360470366,1.51313045236188));
#88457=CARTESIAN_POINT('Ctrl Pts',(-7.86007379151283,0.0116842262656824,
2.80192564298541));
#88458=CARTESIAN_POINT('Ctrl Pts',(-7.72367149571027,-2.01635883652552,
1.70998943732583));
#88459=CARTESIAN_POINT('Ctrl Pts',(-7.64011693457098,-2.36654087854452,
0.458143322760719));
#88460=CARTESIAN_POINT('Ctrl Pts',(-7.60941010809498,-2.36830089438249,
-0.00100592404030229));
#88461=CARTESIAN_POINT('Origin',(-17.306589891905,0.,0.));
#88462=CARTESIAN_POINT('',(-9.80658989190502,-2.36918623645893,-0.00165592778327176));
#88463=CARTESIAN_POINT('',(-9.60941010809498,-2.3754933284252,-0.000487244657051689));
#88464=CARTESIAN_POINT('',(-17.306589891905,-2.37175,-2.3095687792789E-13));
#88465=CARTESIAN_POINT('Ctrl Pts',(-9.80658989190502,-2.36918623645893,
-0.00165592778327162));
#88466=CARTESIAN_POINT('Ctrl Pts',(-9.7878748133918,-2.37099294971461,-0.281234334838761));
#88467=CARTESIAN_POINT('Ctrl Pts',(-9.7163120002153,-2.19606353177059,-1.34810002136817));
#88468=CARTESIAN_POINT('Ctrl Pts',(-9.59190145237552,-0.616578301017466,
-2.733268392497));
#88469=CARTESIAN_POINT('Ctrl Pts',(-9.43335824838566,1.95914233809709,-2.00316904074074));
#88470=CARTESIAN_POINT('Ctrl Pts',(-9.27481504439582,2.74629392962736,0.555692863728672));
#88471=CARTESIAN_POINT('Ctrl Pts',(-9.11627184040596,1.02625846150236,2.60724346329648));
#88472=CARTESIAN_POINT('Ctrl Pts',(-8.9601967895757,-1.58932149542791,2.28366798664447));
#88473=CARTESIAN_POINT('Ctrl Pts',(-8.85696947340871,-2.37259229609025,
0.746888467253723));
#88474=CARTESIAN_POINT('Ctrl Pts',(-8.80658989190501,-2.37538658813648,
-0.000666706255725148));
#88475=CARTESIAN_POINT('Ctrl Pts',(-9.60941010809498,-2.3754933284252,-0.000487244657051797));
#88476=CARTESIAN_POINT('Ctrl Pts',(-9.60762308386372,-2.37556787913775,
-0.0270007296449992));
#88477=CARTESIAN_POINT('Ctrl Pts',(-9.55298832496918,-2.36316749088712,
-0.837527098122419));
#88478=CARTESIAN_POINT('Ctrl Pts',(-9.44550583141135,-1.4428787190723,-2.40187943744293));
#88479=CARTESIAN_POINT('Ctrl Pts',(-9.2869626274215,1.23185716520365,-2.51663500621346));
#88480=CARTESIAN_POINT('Ctrl Pts',(-9.12841942343165,2.78198788226743,-0.333867118596373));
#88481=CARTESIAN_POINT('Ctrl Pts',(-8.96987621944179,1.79234529127704,2.15369965101908));
#88482=CARTESIAN_POINT('Ctrl Pts',(-8.81133301545195,-0.833591533278391,
2.67507924847269));
#88483=CARTESIAN_POINT('Ctrl Pts',(-8.691177645003,-2.24696283819461,1.21936495983762));
#88484=CARTESIAN_POINT('Ctrl Pts',(-8.62387000921735,-2.37267073540056,
0.217748975652233));
#88485=CARTESIAN_POINT('Ctrl Pts',(-8.60941010809498,-2.37080369071248,
0.00210958135936995));
#88486=CARTESIAN_POINT('Origin',(-17.306589891905,0.,0.));
#88487=CARTESIAN_POINT('',(-10.806589891905,-2.36946338337721,0.00177935167763374));
#88488=CARTESIAN_POINT('',(-10.609410108095,-2.36941210437275,-0.00175842403990767));
#88489=CARTESIAN_POINT('',(-17.306589891905,-2.37175,-2.3095687792789E-13));
#88490=CARTESIAN_POINT('Ctrl Pts',(-10.806589891905,-2.36946338337721,0.00177935167763384));
#88491=CARTESIAN_POINT('Ctrl Pts',(-10.7716278880382,-2.36580882662732,
-0.520352810821665));
#88492=CARTESIAN_POINT('Ctrl Pts',(-10.683818149508,-1.93866057672306,-1.837161940075));
#88493=CARTESIAN_POINT('Ctrl Pts',(-10.5431606763146,0.236143210481572,
-2.79198160648));
#88494=CARTESIAN_POINT('Ctrl Pts',(-10.3846174723248,2.47190748456146,-1.31931735926746));
#88495=CARTESIAN_POINT('Ctrl Pts',(-10.2260742683349,2.45098160937866,1.35779750227409));
#88496=CARTESIAN_POINT('Ctrl Pts',(-10.0675310643451,0.192469542788204,
2.79533189117441));
#88497=CARTESIAN_POINT('Ctrl Pts',(-9.92770293886843,-1.9544090201471,1.81246152264369));
#88498=CARTESIAN_POINT('Ctrl Pts',(-9.84072254805508,-2.36589114355968,
0.508240604484572));
#88499=CARTESIAN_POINT('Ctrl Pts',(-9.80658989190502,-2.36918623645893,
-0.00165592778327162));
#88500=CARTESIAN_POINT('Ctrl Pts',(-10.609410108095,-2.36941210437275,-0.00175842403990777));
#88501=CARTESIAN_POINT('Ctrl Pts',(-10.5913761585101,-2.3712723507284,-0.271096991132142));
#88502=CARTESIAN_POINT('Ctrl Pts',(-10.5204944742619,-2.2046407678535,-1.32748836904326));
#88503=CARTESIAN_POINT('Ctrl Pts',(-10.3967650553504,-0.651618847034371,
-2.72512691597345));
#88504=CARTESIAN_POINT('Ctrl Pts',(-10.2382218513606,1.93326279954282,-2.02815649737983));
#88505=CARTESIAN_POINT('Ctrl Pts',(-10.0796786473708,2.75320172762965,0.520388390472216));
#88506=CARTESIAN_POINT('Ctrl Pts',(-9.9211354433809,1.05964722747713,2.59385265257382));
#88507=CARTESIAN_POINT('Ctrl Pts',(-9.76437926362231,-1.57130311251203,
2.30261886074424));
#88508=CARTESIAN_POINT('Ctrl Pts',(-9.660470818527,-2.37336318811748,0.757083557032393));
#88509=CARTESIAN_POINT('Ctrl Pts',(-9.60941010809498,-2.3754933284252,-0.000487244657051797));
#88510=CARTESIAN_POINT('Origin',(-17.306589891905,0.,0.));
#88511=CARTESIAN_POINT('',(-11.806589891905,-2.37551264984338,0.00044757161090019));
#88512=CARTESIAN_POINT('',(-11.609410108095,-2.36923398858465,0.00167909690344512));
#88513=CARTESIAN_POINT('',(-17.306589891905,-2.37175,-2.3095687792789E-13));
#88514=CARTESIAN_POINT('Ctrl Pts',(-11.806589891905,-2.37551264984338,0.000447571610900214));
#88515=CARTESIAN_POINT('Ctrl Pts',(-11.7553809626845,-2.37353748313963,
-0.759305924460025));
#88516=CARTESIAN_POINT('Ctrl Pts',(-11.6513242988008,-1.56735232559126,
-2.30673160249233));
#88517=CARTESIAN_POINT('Ctrl Pts',(-11.4944199002537,1.06689001235037,-2.59088220714646));
#88518=CARTESIAN_POINT('Ctrl Pts',(-11.3358766962639,2.75464506089428,-0.512694348708331));
#88519=CARTESIAN_POINT('Ctrl Pts',(-11.177333492274,1.92758901194037,2.03354997649873));
#88520=CARTESIAN_POINT('Ctrl Pts',(-11.0187902882842,-0.659229957733515,
2.7232959387495));
#88521=CARTESIAN_POINT('Ctrl Pts',(-10.8952090881612,-2.20648540280323,
1.32300329267972));
#88522=CARTESIAN_POINT('Ctrl Pts',(-10.8244756227015,-2.37133296781115,
0.268889764861912));
#88523=CARTESIAN_POINT('Ctrl Pts',(-10.806589891905,-2.36946338337721,0.00177935167763384));
#88524=CARTESIAN_POINT('Ctrl Pts',(-11.609410108095,-2.36923398858465,0.00167909690344501));
#88525=CARTESIAN_POINT('Ctrl Pts',(-11.5751292331565,-2.36587390366334,
-0.510405547231816));
#88526=CARTESIAN_POINT('Ctrl Pts',(-11.4880006235547,-1.95161611255133,
-1.81687917165628));
#88527=CARTESIAN_POINT('Ctrl Pts',(-11.3480242792896,0.200278529009738,
-2.79478305799562));
#88528=CARTESIAN_POINT('Ctrl Pts',(-11.1894810752997,2.45476536426573,-1.35094442384648));
#88529=CARTESIAN_POINT('Ctrl Pts',(-11.0309378713099,2.46821168687189,1.3262182696089));
#88530=CARTESIAN_POINT('Ctrl Pts',(-10.87239466732,0.228341882252721,2.79263026819601));
#88531=CARTESIAN_POINT('Ctrl Pts',(-10.731885412915,-1.94149674627528,1.83275085496228));
#88532=CARTESIAN_POINT('Ctrl Pts',(-10.6442238931734,-2.36582097662153,
0.518188409787725));
#88533=CARTESIAN_POINT('Ctrl Pts',(-10.609410108095,-2.36941210437275,-0.00175842403990777));
#88534=CARTESIAN_POINT('Origin',(-17.306589891905,0.,0.));
#88535=CARTESIAN_POINT('',(-12.806589891905,-2.37074071993608,-0.00210182595080978));
#88536=CARTESIAN_POINT('',(-12.609410108095,-2.3754122575152,0.00062808862859861));
#88537=CARTESIAN_POINT('',(-17.306589891905,-2.37175,-2.3095687792789E-13));
#88538=CARTESIAN_POINT('Ctrl Pts',(-12.806589891905,-2.37074071993608,-0.00210182595080953));
#88539=CARTESIAN_POINT('Ctrl Pts',(-12.7919817719942,-2.37261602100814,
-0.219966362853848));
#88540=CARTESIAN_POINT('Ctrl Pts',(-12.7245259174201,-2.24529599511548,
-1.22384721227819));
#88541=CARTESIAN_POINT('Ctrl Pts',(-12.6042223281827,-0.826114542781323,
-2.67739786594892));
#88542=CARTESIAN_POINT('Ctrl Pts',(-12.4456791241928,1.79835553752813,-2.1486838716176));
#88543=CARTESIAN_POINT('Ctrl Pts',(-12.287135920203,2.78104444218098,0.341638325206172));
#88544=CARTESIAN_POINT('Ctrl Pts',(-12.1285927162131,1.22482132733881,2.52006697848072));
#88545=CARTESIAN_POINT('Ctrl Pts',(-11.9700495122233,-1.4495836885253,2.39783903872389));
#88546=CARTESIAN_POINT('Ctrl Pts',(-11.8627152374539,-2.36423530914187,
0.833082325119274));
#88547=CARTESIAN_POINT('Ctrl Pts',(-11.8082286973478,-2.37557585979512,
0.024761459511004));
#88548=CARTESIAN_POINT('Ctrl Pts',(-11.806589891905,-2.37551264984338,0.000447571610900214));
#88549=CARTESIAN_POINT('Ctrl Pts',(-12.609410108095,-2.3754122575152,0.000628088628598614));
#88550=CARTESIAN_POINT('Ctrl Pts',(-12.5588823078028,-2.37275587159386,
-0.749104589840911));
#88551=CARTESIAN_POINT('Ctrl Pts',(-12.4555067728474,-1.58541971420767,
-2.28779889543668));
#88552=CARTESIAN_POINT('Ctrl Pts',(-12.2992835032286,1.03353864319095,-2.60436589634899));
#88553=CARTESIAN_POINT('Ctrl Pts',(-12.1407402992388,2.74783554884452,-0.548017908917588));
#88554=CARTESIAN_POINT('Ctrl Pts',(-11.9821970952489,1.95353799427501,2.00863464286302));
#88555=CARTESIAN_POINT('Ctrl Pts',(-11.8236538912591,-0.624212206359067,
2.73153490815486));
#88556=CARTESIAN_POINT('Ctrl Pts',(-11.6993915622078,-2.19794407502757,
1.34361468192694));
#88557=CARTESIAN_POINT('Ctrl Pts',(-11.6279769678197,-2.37105384369362,
0.279029187060534));
#88558=CARTESIAN_POINT('Ctrl Pts',(-11.609410108095,-2.36923398858465,0.00167909690344501));
#88559=CARTESIAN_POINT('Origin',(-17.306589891905,0.,0.));
#88560=CARTESIAN_POINT('',(-13.806589891905,-2.36832932812376,0.00104049776686726));
#88561=CARTESIAN_POINT('',(-13.609410108095,-2.37103340387255,-0.00213221344230991));
#88562=CARTESIAN_POINT('',(-17.306589891905,-2.37175,-2.3095687792789E-13));
#88563=CARTESIAN_POINT('Ctrl Pts',(-13.806589891905,-2.36832932812376,0.00104049776686699));
#88564=CARTESIAN_POINT('Ctrl Pts',(-13.7757348466406,-2.36650353915635,
-0.460312200200009));
#88565=CARTESIAN_POINT('Ctrl Pts',(-13.6920320667128,-2.01378149179939,
-1.71444028663224));
#88566=CARTESIAN_POINT('Ctrl Pts',(-13.5554815521218,0.0195128928627424,
-2.80187936245463));
#88567=CARTESIAN_POINT('Ctrl Pts',(-13.3969383481319,2.36247174813047,-1.50653754623712));
#88568=CARTESIAN_POINT('Ctrl Pts',(-13.2383951441421,2.54864912756637,1.16418002319016));
#88569=CARTESIAN_POINT('Ctrl Pts',(-13.0798519401522,0.408075729452012,
2.77207444785609));
#88570=CARTESIAN_POINT('Ctrl Pts',(-12.9359168560732,-1.87348586078252,
1.93427633586112));
#88571=CARTESIAN_POINT('Ctrl Pts',(-12.8448295066575,-2.36583175211693,
0.568201266456078));
#88572=CARTESIAN_POINT('Ctrl Pts',(-12.806589891905,-2.37074071993608,-0.00210182595080953));
#88573=CARTESIAN_POINT('Ctrl Pts',(-13.609410108095,-2.37103340387255,-0.00213221344230973));
#88574=CARTESIAN_POINT('Ctrl Pts',(-13.5954831171125,-2.37286529370797,
-0.209773287942694));
#88575=CARTESIAN_POINT('Ctrl Pts',(-13.5287083914667,-2.25289472910887,
-1.2032522754709));
#88576=CARTESIAN_POINT('Ctrl Pts',(-13.4090859311576,-0.860420371114484,
-2.6665705025054));
#88577=CARTESIAN_POINT('Ctrl Pts',(-13.2505427271678,1.77062098199356,-2.17159522099969));
#88578=CARTESIAN_POINT('Ctrl Pts',(-13.0919995231779,2.78520124435443,0.305905452644607));
#88579=CARTESIAN_POINT('Ctrl Pts',(-12.9334563191881,1.25707446924262,2.50413403614118));
#88580=CARTESIAN_POINT('Ctrl Pts',(-12.7749131151982,-1.41867915221937,
2.41625193356046));
#88581=CARTESIAN_POINT('Ctrl Pts',(-12.6668977115005,-2.35927592169033,
0.853512735567485));
#88582=CARTESIAN_POINT('Ctrl Pts',(-12.6117300424661,-2.37553422286826,
0.0350513289019418));
#88583=CARTESIAN_POINT('Ctrl Pts',(-12.609410108095,-2.3754122575152,0.000628088628598614));
#88584=CARTESIAN_POINT('Origin',(-17.306589891905,0.,0.));
#88585=CARTESIAN_POINT('',(-14.806589891905,-2.37447732889499,0.00158904524625122));
#88586=CARTESIAN_POINT('',(-14.609410108095,-2.36819900096358,0.000905669814256771));
#88587=CARTESIAN_POINT('',(-17.306589891905,-2.37175,-2.3095687792789E-13));
#88588=CARTESIAN_POINT('Ctrl Pts',(-14.806589891905,-2.37447732889499,0.00158904524625127));
#88589=CARTESIAN_POINT('Ctrl Pts',(-14.7594879212869,-2.36948883111584,
-0.697977827885181));
#88590=CARTESIAN_POINT('Ctrl Pts',(-14.6595382160056,-1.67293185990106,
-2.19161085343155));
#88591=CARTESIAN_POINT('Ctrl Pts',(-14.5067407760609,0.863349698447385,
-2.66549172608374));
#88592=CARTESIAN_POINT('Ctrl Pts',(-14.348197572071,2.70673094384455,-0.724268682598567));
#88593=CARTESIAN_POINT('Ctrl Pts',(-14.1896543680812,2.07909181188049,1.87842405436525));
#88594=CARTESIAN_POINT('Ctrl Pts',(-14.0311111640913,-0.44664765932035,
2.76610238818825));
#88595=CARTESIAN_POINT('Ctrl Pts',(-13.9034230053659,-2.15242365769109,
1.44726882168644));
#88596=CARTESIAN_POINT('Ctrl Pts',(-13.8285825813038,-2.36963070393844,
0.329880935456426));
#88597=CARTESIAN_POINT('Ctrl Pts',(-13.806589891905,-2.36832932812376,0.00104049776686699));
#88598=CARTESIAN_POINT('Ctrl Pts',(-14.609410108095,-2.36819900096358,0.000905669814256944));
#88599=CARTESIAN_POINT('Ctrl Pts',(-14.5792361917588,-2.36667741525576,
-0.450328646933255));
#88600=CARTESIAN_POINT('Ctrl Pts',(-14.4962145407594,-2.02556427845193,
-1.69402330663087));
#88601=CARTESIAN_POINT('Ctrl Pts',(-14.3603451550967,-0.0164545272929353,
-2.80188230448376));
#88602=CARTESIAN_POINT('Ctrl Pts',(-14.2018019511069,2.34293162102215,-1.53675277767917));
#88603=CARTESIAN_POINT('Ctrl Pts',(-14.043258747117,2.56338713804141,1.13136735389903));
#88604=CARTESIAN_POINT('Ctrl Pts',(-13.8847155431272,0.443630763460945,
2.76660429639169));
#88605=CARTESIAN_POINT('Ctrl Pts',(-13.7400993301198,-1.8593443188828,1.95434500217413));
#88606=CARTESIAN_POINT('Ctrl Pts',(-13.6483308517758,-2.36591395525473,
0.578147119572609));
#88607=CARTESIAN_POINT('Ctrl Pts',(-13.609410108095,-2.37103340387255,-0.00213221344230973));
#88608=CARTESIAN_POINT('Origin',(-0.25,3.51939854619125E-16,0.));
#88609=CARTESIAN_POINT('Ctrl Pts',(-0.25,2.22665730523966,0.827839780511539));
#88610=CARTESIAN_POINT('Ctrl Pts',(-0.25,2.21253493697841,0.887066447970513));
#88611=CARTESIAN_POINT('Ctrl Pts',(-0.249999999999997,2.19601471711402,
0.945593270349512));
#88612=CARTESIAN_POINT('Ctrl Pts',(-0.249999999999997,2.17708701742544,
1.00327396853317));
#88613=CARTESIAN_POINT('Ctrl Pts',(-0.249999999999997,2.15165423815579,
1.08077839269253));
#88614=CARTESIAN_POINT('Ctrl Pts',(-0.250000000000005,2.12187728230406,
1.15675586863499));
#88615=CARTESIAN_POINT('Ctrl Pts',(-0.250000000000004,2.08808045010065,
1.23103089813193));
#88616=CARTESIAN_POINT('Ctrl Pts',(-0.250000000000003,2.06840578169053,
1.27426976051136));
#88617=CARTESIAN_POINT('Ctrl Pts',(-0.25,2.0473677896996,1.31693163959809));
#88618=CARTESIAN_POINT('Ctrl Pts',(-0.250000000000001,2.02502259951598,
1.35898078015481));
#88619=CARTESIAN_POINT('Ctrl Pts',(-0.250000000000001,2.01629265380112,
1.37540877702575));
#88620=CARTESIAN_POINT('Ctrl Pts',(-0.249999999999999,2.00736312468595,
1.39174323478388));
#88621=CARTESIAN_POINT('Ctrl Pts',(-0.249999999999999,1.99823713884684,
1.40798196099185));
#88622=CARTESIAN_POINT('Ctrl Pts',(-0.249999999999999,1.99115494736671,
1.42058397138565));
#88623=CARTESIAN_POINT('Ctrl Pts',(-0.250000000000001,1.98395548148856,
1.43312635989235));
#88624=CARTESIAN_POINT('Ctrl Pts',(-0.250000000000001,1.97664492917627,
1.4456004937163));
#88625=CARTESIAN_POINT('Ctrl Pts',(-0.250000000000002,1.93344420468633,
1.51931470784926));
#88626=CARTESIAN_POINT('Ctrl Pts',(-0.249999999999999,1.88632573736469,
1.59072308909904));
#88627=CARTESIAN_POINT('Ctrl Pts',(-0.249999999999999,1.83564389935666,
1.65963329088958));
#88628=CARTESIAN_POINT('Ctrl Pts',(-0.249999999999999,1.79139338401687,
1.71979906350653));
#88629=CARTESIAN_POINT('Ctrl Pts',(-0.249999999999997,1.74442536456685,
1.77806067486507));
#88630=CARTESIAN_POINT('Ctrl Pts',(-0.249999999999997,1.69494407121667,
1.8342821297957));
#88631=CARTESIAN_POINT('Ctrl Pts',(-0.249999999999997,1.67108524646734,
1.86139091676392));
#88632=CARTESIAN_POINT('Ctrl Pts',(-0.249999999999999,1.64664168508504,
1.88802522921354));
#88633=CARTESIAN_POINT('Ctrl Pts',(-0.25,1.62163414288635,1.91416882292567));
#88634=CARTESIAN_POINT('Ctrl Pts',(-0.25,1.606390797066,1.93010464887667));
#88635=CARTESIAN_POINT('Ctrl Pts',(-0.249999999999998,1.59093334989609,
1.94586244562507));
#88636=CARTESIAN_POINT('Ctrl Pts',(-0.249999999999998,1.57529127421572,
1.96141409772889));
#88637=CARTESIAN_POINT('Ctrl Pts',(-0.249999999999998,1.51243278415657,
2.02390921596938));
#88638=CARTESIAN_POINT('Ctrl Pts',(-0.249999999999999,1.44653991914015,
2.08313958788272));
#88639=CARTESIAN_POINT('Ctrl Pts',(-0.249999999999999,1.37797049065438,
2.13890775763005));
#88640=CARTESIAN_POINT('Ctrl Pts',(-0.249999999999998,1.30477974292812,
2.19843449036313));
#88641=CARTESIAN_POINT('Ctrl Pts',(-0.249999999999999,1.22853932099898,
2.25401777387017));
#88642=CARTESIAN_POINT('Ctrl Pts',(-0.249999999999998,1.14962650113067,
2.30539173571991));
#88643=CARTESIAN_POINT('Ctrl Pts',(-0.249999999999998,1.09044188622944,
2.34392220710722));
#88644=CARTESIAN_POINT('Ctrl Pts',(-0.25,1.02975273329805,2.38008449190169));
#88645=CARTESIAN_POINT('Ctrl Pts',(-0.25,0.967700507001693,2.41375165933649));
#88646=CARTESIAN_POINT('Ctrl Pts',(-0.250000000000001,0.921161337279424,
2.43900203491258));
#88647=CARTESIAN_POINT('Ctrl Pts',(-0.249999999999997,0.873855113607986,
2.46284866395087));
#88648=CARTESIAN_POINT('Ctrl Pts',(-0.249999999999997,0.825837112674175,
2.48523195686642));
#88649=CARTESIAN_POINT('Ctrl Pts',(-0.249999999999997,0.812484513410199,
2.4914561880859));
#88650=CARTESIAN_POINT('Ctrl Pts',(-0.249999999999995,0.799076856063629,
2.49756723169206));
#88651=CARTESIAN_POINT('Ctrl Pts',(-0.249999999999995,0.785615286660712,
2.50356372448443));
#88652=CARTESIAN_POINT('Ctrl Pts',(-0.249999999999995,0.772636490123328,
2.5093451647876));
#88653=CARTESIAN_POINT('Ctrl Pts',(-0.250000000000001,0.759614812827758,
2.51501686886279));
#88654=CARTESIAN_POINT('Ctrl Pts',(-0.250000000000001,0.746556237332744,
2.52057598998014));
#88655=CARTESIAN_POINT('Ctrl Pts',(-0.250000000000002,0.661371947117411,
2.55683950025228));
#88656=CARTESIAN_POINT('Ctrl Pts',(-0.249999999999992,0.574557887090518,
2.58834304940443));
#88657=CARTESIAN_POINT('Ctrl Pts',(-0.249999999999994,0.48646010071724,
2.61485457170675));
#88658=CARTESIAN_POINT('Ctrl Pts',(-0.249999999999995,0.450950611910523,
2.62554054513694));
#88659=CARTESIAN_POINT('Ctrl Pts',(-0.250000000000001,0.415232105718096,
2.6354151139179));
#88660=CARTESIAN_POINT('Ctrl Pts',(-0.250000000000001,0.379325561708904,
2.64446137371408));
#88661=CARTESIAN_POINT('Ctrl Pts',(-0.25,0.2933372621455,2.66612518232464));
#88662=CARTESIAN_POINT('Ctrl Pts',(-0.249999999999999,0.206272069189806,
2.68304215953505));
#88663=CARTESIAN_POINT('Ctrl Pts',(-0.249999999999998,0.11844610394434,
2.69538014091633));
#88664=CARTESIAN_POINT('Ctrl Pts',(-0.249999999999998,0.0288600713565845,
2.70796538036119));
#88665=CARTESIAN_POINT('Ctrl Pts',(-0.249999999999999,-0.0615182634234459,
2.71578635010443));
#88666=CARTESIAN_POINT('Ctrl Pts',(-0.249999999999998,-0.152370710138942,
2.71896997432629));
#88667=CARTESIAN_POINT('Ctrl Pts',(-0.249999999999998,-0.17073330596056,
2.71961343090833));
#88668=CARTESIAN_POINT('Ctrl Pts',(-0.249999999999995,-0.189115303514798,
2.7200672839337));
#88669=CARTESIAN_POINT('Ctrl Pts',(-0.249999999999995,-0.20751411631365,
2.72033232888479));
#88670=CARTESIAN_POINT('Ctrl Pts',(-0.249999999999994,-0.221324751245115,
2.72053127862683));
#88671=CARTESIAN_POINT('Ctrl Pts',(-0.25,-0.235143715204858,2.72062376322601));
#88672=CARTESIAN_POINT('Ctrl Pts',(-0.25,-0.248957210752076,2.72061034785803));
#88673=CARTESIAN_POINT('Ctrl Pts',(-0.250000000000001,-0.341482715415868,
2.72052048908994));
#88674=CARTESIAN_POINT('Ctrl Pts',(-0.249999999999998,-0.433912331818891,
2.71568618768959));
#88675=CARTESIAN_POINT('Ctrl Pts',(-0.249999999999999,-0.525897798319606,
2.70631418714313));
#88676=CARTESIAN_POINT('Ctrl Pts',(-0.249999999999999,-0.619674068827689,
2.69675972933713));
#88677=CARTESIAN_POINT('Ctrl Pts',(-0.25,-0.712989524571036,2.68248921578258));
#88678=CARTESIAN_POINT('Ctrl Pts',(-0.249999999999999,-0.805492806230512,
2.66366898531223));
#88679=CARTESIAN_POINT('Ctrl Pts',(-0.249999999999997,-0.898813914036067,
2.64468236424171));
#88680=CARTESIAN_POINT('Ctrl Pts',(-0.249999999999998,-0.991309340568736,
2.62106517248096));
#88681=CARTESIAN_POINT('Ctrl Pts',(-0.249999999999997,-1.08262302389016,
2.59293522572841));
#88682=CARTESIAN_POINT('Ctrl Pts',(-0.249999999999997,-1.1353317955791,
2.57669784610389));
#88683=CARTESIAN_POINT('Ctrl Pts',(-0.250000000000005,-1.18764683585401,
2.55895587944617));
#88684=CARTESIAN_POINT('Ctrl Pts',(-0.250000000000006,-1.23949850126476,
2.53972416718926));
#88685=CARTESIAN_POINT('Ctrl Pts',(-0.250000000000006,-1.25272255783918,
2.53481938257157));
#88686=CARTESIAN_POINT('Ctrl Pts',(-0.250000000000002,-1.26591860367828,
2.52981684034259));
#88687=CARTESIAN_POINT('Ctrl Pts',(-0.250000000000002,-1.27907848770803,
2.52471944034195));
#88688=CARTESIAN_POINT('Ctrl Pts',(-0.250000000000002,-1.37073515539029,
2.48921679481363));
#88689=CARTESIAN_POINT('Ctrl Pts',(-0.250000000000005,-1.46040274807117,
2.44920963606695));
#88690=CARTESIAN_POINT('Ctrl Pts',(-0.250000000000005,-1.54771241082929,
2.40488333309869));
#88691=CARTESIAN_POINT('Ctrl Pts',(-0.250000000000005,-1.63531255634976,
2.36040955473625));
#88692=CARTESIAN_POINT('Ctrl Pts',(-0.250000000000003,-1.72054002860748,
2.31158770014214));
#88693=CARTESIAN_POINT('Ctrl Pts',(-0.250000000000004,-1.80302121060508,
2.2585523933109));
#88694=CARTESIAN_POINT('Ctrl Pts',(-0.250000000000005,-1.88397085596804,
2.2065018628053));
#88695=CARTESIAN_POINT('Ctrl Pts',(-0.25,-1.96227614017533,2.15039259324176));
#88696=CARTESIAN_POINT('Ctrl Pts',(-0.250000000000001,-2.03756910697441,
2.09030490667818));
#88697=CARTESIAN_POINT('Ctrl Pts',(-0.250000000000001,-2.0994426421019,
2.04092662151587));
#88698=CARTESIAN_POINT('Ctrl Pts',(-0.250000000000001,-2.15928191063436,
1.98886079770323));
#88699=CARTESIAN_POINT('Ctrl Pts',(-0.250000000000001,-2.21686865784453,
1.93412961144453));
#88700=CARTESIAN_POINT('',(-0.25,-3.60291088309151E-16,2.942));
#88701=CARTESIAN_POINT('Origin',(-0.25,0.,0.));
#88702=CARTESIAN_POINT('',(-0.25,-2.89149574471101,-0.555476496098387));
#88703=CARTESIAN_POINT('Origin',(-0.25,0.,0.));
#88704=CARTESIAN_POINT('Ctrl Pts',(-0.25,-2.89371419577505,-0.556479620053392));
#88705=CARTESIAN_POINT('Ctrl Pts',(-0.25,-2.87319648930919,-0.628281513663384));
#88706=CARTESIAN_POINT('Ctrl Pts',(-0.250000000000005,-2.8497945550991,
-0.699127993612092));
#88707=CARTESIAN_POINT('Ctrl Pts',(-0.250000000000004,-2.82345497557192,
-0.768854229344188));
#88708=CARTESIAN_POINT('Ctrl Pts',(-0.250000000000004,-2.78891200574704,
-0.860296511268678));
#88709=CARTESIAN_POINT('Ctrl Pts',(-0.249999999999999,-2.74931759817973,
-0.949813518739235));
#88710=CARTESIAN_POINT('Ctrl Pts',(-0.25,-2.7049917476029,-1.03713570465333));
#88711=CARTESIAN_POINT('Ctrl Pts',(-0.250000000000001,-2.68151631903656,
-1.0833824367748));
#88712=CARTESIAN_POINT('Ctrl Pts',(-0.250000000000004,-2.65671306618578,
-1.12901301630281));
#88713=CARTESIAN_POINT('Ctrl Pts',(-0.250000000000004,-2.63062539793924,
-1.17398328280867));
#88714=CARTESIAN_POINT('Ctrl Pts',(-0.250000000000004,-2.61659733378916,
-1.19816504475953));
#88715=CARTESIAN_POINT('Ctrl Pts',(-0.250000000000005,-2.60219783598583,
-1.22215582354875));
#88716=CARTESIAN_POINT('Ctrl Pts',(-0.250000000000005,-2.58743338226914,
-1.24594836073162));
#88717=CARTESIAN_POINT('Ctrl Pts',(-0.250000000000006,-2.57841221178637,
-1.26048574479356));
#88718=CARTESIAN_POINT('Ctrl Pts',(-0.250000000000002,-2.5692556860291,
-1.27494753731645));
#88719=CARTESIAN_POINT('Ctrl Pts',(-0.250000000000002,-2.55997180439406,
-1.28932244956251));
#88720=CARTESIAN_POINT('Ctrl Pts',(-0.250000000000001,-2.50722268190062,
-1.37099776994114));
#88721=CARTESIAN_POINT('Ctrl Pts',(-0.249999999999998,-2.45031051886283,
-1.44996023242765));
#88722=CARTESIAN_POINT('Ctrl Pts',(-0.249999999999997,-2.38955315391405,
-1.52594513247122));
#88723=CARTESIAN_POINT('Ctrl Pts',(-0.249999999999997,-2.33964731266927,
-1.58835880629945));
#88724=CARTESIAN_POINT('Ctrl Pts',(-0.250000000000005,-2.28714614339243,
-1.64876308353032));
#88725=CARTESIAN_POINT('Ctrl Pts',(-0.250000000000005,-2.23221010314724,
-1.70699014883082));
#88726=CARTESIAN_POINT('Ctrl Pts',(-0.250000000000006,-2.2077967295152,
-1.73286604185723));
#88727=CARTESIAN_POINT('Ctrl Pts',(-0.250000000000001,-2.18290234415457,
-1.75831168687554));
#88728=CARTESIAN_POINT('Ctrl Pts',(-0.250000000000001,-2.15754040351483,
-1.7833109594478));
#88729=CARTESIAN_POINT('Ctrl Pts',(-0.250000000000001,-2.14235758353611,
-1.79827666970062));
#88730=CARTESIAN_POINT('Ctrl Pts',(-0.250000000000002,-2.12700719616793,
-1.81308239326784));
#88731=CARTESIAN_POINT('Ctrl Pts',(-0.250000000000002,-2.11149207982293,
-1.82772451114123));
#88732=CARTESIAN_POINT('Ctrl Pts',(-0.250000000000002,-2.10034093269375,
-1.83824820990432));
#88733=CARTESIAN_POINT('Ctrl Pts',(-0.250000000000001,-2.08910489602872,
-1.8486870996063));
#88734=CARTESIAN_POINT('Ctrl Pts',(-0.250000000000001,-2.07779536845615,
-1.85903064245993));
#88735=CARTESIAN_POINT('Ctrl Pts',(-0.250000000000001,-2.00763237329104,
-1.92320078065298));
#88736=CARTESIAN_POINT('Ctrl Pts',(-0.250000000000004,-1.93454403565031,
-1.98379921146077));
#88737=CARTESIAN_POINT('Ctrl Pts',(-0.250000000000003,-1.85882259425096,
-2.04057766488801));
#88738=CARTESIAN_POINT('Ctrl Pts',(-0.250000000000002,-1.78043266758531,
-2.0993570372573));
#88739=CARTESIAN_POINT('Ctrl Pts',(-0.249999999999999,-1.69921998861886,
-2.15404336229777));
#88740=CARTESIAN_POINT('Ctrl Pts',(-0.249999999999998,-1.61548348714018,
-2.20430748725186));
#88741=CARTESIAN_POINT('Ctrl Pts',(-0.249999999999998,-1.53798869174479,
-2.2508249319774));
#88742=CARTESIAN_POINT('Ctrl Pts',(-0.250000000000001,-1.45833145198356,
-2.29355469232131));
#88743=CARTESIAN_POINT('Ctrl Pts',(-0.250000000000001,-1.37673980248905,
-2.33218716905464));
#88744=CARTESIAN_POINT('Ctrl Pts',(-0.250000000000001,-1.32909704313918,
-2.35474533283119));
#88745=CARTESIAN_POINT('Ctrl Pts',(-0.250000000000003,-1.28079462304566,
-2.37590557784026));
#88746=CARTESIAN_POINT('Ctrl Pts',(-0.250000000000003,-1.23187796096567,
-2.39559798168754));
#88747=CARTESIAN_POINT('Ctrl Pts',(-0.250000000000003,-1.21499175511448,
-2.40239586958362));
#88748=CARTESIAN_POINT('Ctrl Pts',(-0.250000000000002,-1.19802860580916,
-2.40902009027204));
#88749=CARTESIAN_POINT('Ctrl Pts',(-0.250000000000002,-1.18101594114361,
-2.41545826461572));
#88750=CARTESIAN_POINT('Ctrl Pts',(-0.250000000000001,-1.09759886515225,
-2.44702614002095));
#88751=CARTESIAN_POINT('Ctrl Pts',(-0.250000000000005,-1.01287967862669,
-2.4741726092685));
#88752=CARTESIAN_POINT('Ctrl Pts',(-0.250000000000005,-0.927092223399418,
-2.49664604416005));
#88753=CARTESIAN_POINT('Ctrl Pts',(-0.250000000000004,-0.886487901330664,
-2.5072830141682));
#88754=CARTESIAN_POINT('Ctrl Pts',(-0.249999999999998,-0.84564411064597,
-2.51687238559944));
#88755=CARTESIAN_POINT('Ctrl Pts',(-0.249999999999998,-0.804585174478583,
-2.52538339335047));
#88756=CARTESIAN_POINT('Ctrl Pts',(-0.249999999999999,-0.716013041901021,
-2.54374329687598));
#88757=CARTESIAN_POINT('Ctrl Pts',(-0.25,-0.626439022336421,-2.55708831331885));
#88758=CARTESIAN_POINT('Ctrl Pts',(-0.250000000000001,-0.536235855388279,
-2.56552072220656));
#88759=CARTESIAN_POINT('Ctrl Pts',(-0.250000000000002,-0.443708985077977,
-2.57417035647057));
#88760=CARTESIAN_POINT('Ctrl Pts',(-0.25,-0.350519004198512,-2.57765081355158));
#88761=CARTESIAN_POINT('Ctrl Pts',(-0.25,-0.257086776744317,-2.57601949021612));
#88762=CARTESIAN_POINT('Ctrl Pts',(-0.25,-0.243661630645749,-2.57578508764744));
#88763=CARTESIAN_POINT('Ctrl Pts',(-0.250000000000003,-0.230231530774191,
-2.57544506120073));
#88764=CARTESIAN_POINT('Ctrl Pts',(-0.250000000000003,-0.21679777797424,
-2.57499949833529));
#88765=CARTESIAN_POINT('Ctrl Pts',(-0.250000000000003,-0.202668222536943,
-2.57453085749444));
#88766=CARTESIAN_POINT('Ctrl Pts',(-0.250000000000004,-0.188542730400431,
-2.57394570730987));
#88767=CARTESIAN_POINT('Ctrl Pts',(-0.250000000000004,-0.174427630795246,
-2.57324484391326));
#88768=CARTESIAN_POINT('Ctrl Pts',(-0.250000000000003,-0.0858016677984528,
-2.56884425906505));
#88769=CARTESIAN_POINT('Ctrl Pts',(-0.250000000000001,0.00247755739145698,
-2.55988411430444));
#88770=CARTESIAN_POINT('Ctrl Pts',(-0.250000000000002,0.0900618971462069,
-2.54649071805601));
#88771=CARTESIAN_POINT('Ctrl Pts',(-0.250000000000002,0.177515102319017,
-2.53311737490637));
#88772=CARTESIAN_POINT('Ctrl Pts',(-0.250000000000002,0.264276427722839,
-2.51532361020355));
#88773=CARTESIAN_POINT('Ctrl Pts',(-0.250000000000002,0.349981301201772,
-2.49318670047294));
#88774=CARTESIAN_POINT('Ctrl Pts',(-0.250000000000002,0.434317736638152,
-2.47140324776513));
#88775=CARTESIAN_POINT('Ctrl Pts',(-0.250000000000002,0.517631958865446,
-2.44541374332064));
#88776=CARTESIAN_POINT('Ctrl Pts',(-0.250000000000002,0.599546682957301,
-2.41525188469741));
#88777=CARTESIAN_POINT('Ctrl Pts',(-0.250000000000002,0.627537361614373,
-2.40494542390196));
#88778=CARTESIAN_POINT('Ctrl Pts',(-0.249999999999999,0.655364319587099,
-2.39415147439514));
#88779=CARTESIAN_POINT('Ctrl Pts',(-0.249999999999999,0.683011442265382,
-2.38287044100979));
#88780=CARTESIAN_POINT('Ctrl Pts',(-0.249999999999999,0.70026444827292,
-2.37583058593939));
#88781=CARTESIAN_POINT('Ctrl Pts',(-0.250000000000004,0.717447409397925,
-2.3686010365864));
#88782=CARTESIAN_POINT('Ctrl Pts',(-0.250000000000004,0.734556286227355,
-2.36118180434677));
#88783=CARTESIAN_POINT('Ctrl Pts',(-0.250000000000005,0.747119478010523,
-2.35573379987285));
#88784=CARTESIAN_POINT('Ctrl Pts',(-0.249999999999999,0.759634939071271,
-2.35018686706227));
#88785=CARTESIAN_POINT('Ctrl Pts',(-0.249999999999999,0.772097715167772,
-2.34454300922358));
#88786=CARTESIAN_POINT('Ctrl Pts',(-0.249999999999999,0.849775762223969,
-2.30936594663516));
#88787=CARTESIAN_POINT('Ctrl Pts',(-0.249999999999998,0.925455358875783,
-2.27040707536139));
#88788=CARTESIAN_POINT('Ctrl Pts',(-0.249999999999999,0.998809291101006,
-2.22774211242364));
#88789=CARTESIAN_POINT('Ctrl Pts',(-0.25,1.07101111120779,-2.18574725426885));
#88790=CARTESIAN_POINT('Ctrl Pts',(-0.25,1.14096041241647,-2.14016132509184));
#88791=CARTESIAN_POINT('Ctrl Pts',(-0.250000000000002,1.20831094189049,
-2.0910204724465));
#88792=CARTESIAN_POINT('Ctrl Pts',(-0.250000000000003,1.27356246615044,
-2.04341111341719));
#88793=CARTESIAN_POINT('Ctrl Pts',(-0.25,1.33637510283447,-1.99246448542687));
#88794=CARTESIAN_POINT('Ctrl Pts',(-0.250000000000001,1.39639388640012,
-1.93818640597136));
#88795=CARTESIAN_POINT('Ctrl Pts',(-0.250000000000001,1.43371761251259,
-1.90443263671525));
#88796=CARTESIAN_POINT('Ctrl Pts',(-0.250000000000001,1.4699600853265,-1.86939002404756));
#88797=CARTESIAN_POINT('Ctrl Pts',(-0.250000000000001,1.50502666328431,
-1.8330555925294));
#88798=CARTESIAN_POINT('Ctrl Pts',(-15.7872339910054,-1.03908919352511,
2.13201587949043));
#88799=CARTESIAN_POINT('Ctrl Pts',(-15.7343862563421,-1.74702956476549,
1.78698412034994));
#88800=CARTESIAN_POINT('Ctrl Pts',(-15.6286907870155,-2.78011294947163,
0.342389453078488));
#88801=CARTESIAN_POINT('Ctrl Pts',(-15.4701475830257,-1.79667481887822,
-2.15247714088935));
#88802=CARTESIAN_POINT('Ctrl Pts',(-15.3116043790358,0.829372328041529,
-2.67555139502504));
#88803=CARTESIAN_POINT('Ctrl Pts',(-15.153061175046,2.69704440340713,-0.759379027323357));
#88804=CARTESIAN_POINT('Ctrl Pts',(-14.9945179710561,2.10312284761966,1.85179574340887));
#88805=CARTESIAN_POINT('Ctrl Pts',(-14.8359747670663,-0.411142958056525,
2.77149379088676));
#88806=CARTESIAN_POINT('Ctrl Pts',(-14.6774315630764,-2.54988918864703,
1.1614740258459));
#88807=CARTESIAN_POINT('Ctrl Pts',(-14.5188883590866,-2.36084355622959,
-1.50914432504944));
#88808=CARTESIAN_POINT('Ctrl Pts',(-14.3603451550967,-0.0164545272929353,
-2.80188230448376));
#88809=CARTESIAN_POINT('Ctrl Pts',(-14.2018019511069,2.34293162102215,-1.53675277767917));
#88810=CARTESIAN_POINT('Ctrl Pts',(-14.043258747117,2.56338713804141,1.13136735389903));
#88811=CARTESIAN_POINT('Ctrl Pts',(-13.8847155431272,0.443630763460945,
2.76660429639169));
#88812=CARTESIAN_POINT('Ctrl Pts',(-13.7261723391373,-2.08112798018708,
1.87612190650057));
#88813=CARTESIAN_POINT('Ctrl Pts',(-13.5676291351475,-2.70595460958226,
-0.727142408722851));
#88814=CARTESIAN_POINT('Ctrl Pts',(-13.4090859311576,-0.860420371114484,
-2.6665705025054));
#88815=CARTESIAN_POINT('Ctrl Pts',(-13.2505427271678,1.77062098199356,-2.17159522099969));
#88816=CARTESIAN_POINT('Ctrl Pts',(-13.0919995231779,2.78520124435443,0.305905452644607));
#88817=CARTESIAN_POINT('Ctrl Pts',(-12.9334563191881,1.25707446924262,2.50413403614118));
#88818=CARTESIAN_POINT('Ctrl Pts',(-12.7749131151982,-1.41867915221937,
2.41625193356046));
#88819=CARTESIAN_POINT('Ctrl Pts',(-12.6163699112084,-2.79927136767585,
0.122489461091731));
#88820=CARTESIAN_POINT('Ctrl Pts',(-12.4578267072185,-1.6243115612719,-2.28309783734224));
#88821=CARTESIAN_POINT('Ctrl Pts',(-12.2992835032286,1.03353864319095,-2.60436589634899));
#88822=CARTESIAN_POINT('Ctrl Pts',(-12.1407402992388,2.74783554884452,-0.548017908917588));
#88823=CARTESIAN_POINT('Ctrl Pts',(-11.9821970952489,1.95353799427501,2.00863464286302));
#88824=CARTESIAN_POINT('Ctrl Pts',(-11.8236538912591,-0.624212206359067,
2.73153490815486));
#88825=CARTESIAN_POINT('Ctrl Pts',(-11.6651106872692,-2.63209741649849,
0.960722134658545));
#88826=CARTESIAN_POINT('Ctrl Pts',(-11.5065674832794,-2.23704952747652,
-1.68716722370331));
#88827=CARTESIAN_POINT('Ctrl Pts',(-11.3480242792896,0.200278529009738,
-2.79478305799562));
#88828=CARTESIAN_POINT('Ctrl Pts',(-11.1894810752997,2.45476536426573,-1.35094442384648));
#88829=CARTESIAN_POINT('Ctrl Pts',(-11.0309378713099,2.46821168687189,1.3262182696089));
#88830=CARTESIAN_POINT('Ctrl Pts',(-10.87239466732,0.228341882252721,2.79263026819601));
#88831=CARTESIAN_POINT('Ctrl Pts',(-10.7138514633301,-2.21998915305615,
1.70955315514429));
#88832=CARTESIAN_POINT('Ctrl Pts',(-10.5553082593403,-2.64161502869699,
-0.934234376434406));
#88833=CARTESIAN_POINT('Ctrl Pts',(-10.3967650553504,-0.651618847034371,
-2.72512691597345));
#88834=CARTESIAN_POINT('Ctrl Pts',(-10.2382218513606,1.93326279954282,-2.02815649737983));
#88835=CARTESIAN_POINT('Ctrl Pts',(-10.0796786473708,2.75320172762965,0.520388390472216));
#88836=CARTESIAN_POINT('Ctrl Pts',(-9.9211354433809,1.05964722747713,2.59385265257382));
#88837=CARTESIAN_POINT('Ctrl Pts',(-9.76259223939105,-1.60129600986408,
2.29929878849087));
#88838=CARTESIAN_POINT('Ctrl Pts',(-9.6040490354012,-2.80036053447984,-0.0943647544917269));
#88839=CARTESIAN_POINT('Ctrl Pts',(-9.44550583141135,-1.4428787190723,-2.40187943744293));
#88840=CARTESIAN_POINT('Ctrl Pts',(-9.2869626274215,1.23185716520365,-2.51663500621346));
#88841=CARTESIAN_POINT('Ctrl Pts',(-9.12841942343165,2.78198788226743,-0.333867118596373));
#88842=CARTESIAN_POINT('Ctrl Pts',(-8.96987621944179,1.79234529127704,2.15369965101908));
#88843=CARTESIAN_POINT('Ctrl Pts',(-8.81133301545195,-0.833591533278391,
2.67507924847269));
#88844=CARTESIAN_POINT('Ctrl Pts',(-8.65278981146209,-2.69851371088473,
0.754286140751512));
#88845=CARTESIAN_POINT('Ctrl Pts',(-8.49424660747226,-2.09986904910667,
-1.85512096817608));
#88846=CARTESIAN_POINT('Ctrl Pts',(-8.33570340348239,0.415818959741428,
-2.77092374898376));
#88847=CARTESIAN_POINT('Ctrl Pts',(-8.17716019949255,2.55189140603955,-1.15705405307796));
#88848=CARTESIAN_POINT('Ctrl Pts',(-8.0186169955027,2.35825360470366,1.51313045236188));
#88849=CARTESIAN_POINT('Ctrl Pts',(-7.86007379151283,0.0116842262656824,
2.80192564298541));
#88850=CARTESIAN_POINT('Ctrl Pts',(-7.701530587523,-2.34555208792137,1.53274565170167));
#88851=CARTESIAN_POINT('Ctrl Pts',(-7.54298738353314,-2.56145248058093,
-1.13573105077235));
#88852=CARTESIAN_POINT('Ctrl Pts',(-7.38444417954329,-0.438913988766854,
-2.76735945269628));
#88853=CARTESIAN_POINT('Ctrl Pts',(-7.22590097555344,2.08432431928549,-1.87256934771392));
#88854=CARTESIAN_POINT('Ctrl Pts',(-7.06735777156358,2.70471060372122,0.731754316748925));
#88855=CARTESIAN_POINT('Ctrl Pts',(-6.90881456757374,0.855872690191172,
2.66803406427797));
#88856=CARTESIAN_POINT('Ctrl Pts',(-6.75027136358388,-1.77432111187291,
2.16857289984097));
#88857=CARTESIAN_POINT('Ctrl Pts',(-6.59172815959403,-2.78467557941811,
-0.310653741898083));
#88858=CARTESIAN_POINT('Ctrl Pts',(-6.43318495560419,-1.2528030468829,-2.50627379902584));
#88859=CARTESIAN_POINT('Ctrl Pts',(-6.27464175161433,1.42279687533745,-2.41382950547303));
#88860=CARTESIAN_POINT('Ctrl Pts',(-6.11609854762448,2.79947614093066,-0.117716465815816));
#88861=CARTESIAN_POINT('Ctrl Pts',(-5.95755534363463,1.62041646007026,2.285864021742));
#88862=CARTESIAN_POINT('Ctrl Pts',(-5.79901213964478,-1.0379776562294,2.60259989532173));
#88863=CARTESIAN_POINT('Ctrl Pts',(-5.64046893565492,-2.74876593914578,
0.543331981173054));
#88864=CARTESIAN_POINT('Ctrl Pts',(-5.48192573166508,-1.95011037910057,
-2.01196255911331));
#88865=CARTESIAN_POINT('Ctrl Pts',(-5.32338252767523,0.628868639624235,
-2.73046663851582));
#88866=CARTESIAN_POINT('Ctrl Pts',(-5.16483932368538,2.63373164752747,-0.956232941728888));
#88867=CARTESIAN_POINT('Ctrl Pts',(-5.00629611969553,2.23416961039886,1.6909790010008));
#88868=CARTESIAN_POINT('Ctrl Pts',(-4.84775291570567,-0.205043418049532,
2.79443751524972));
#88869=CARTESIAN_POINT('Ctrl Pts',(-4.68920971171582,-2.45706519272027,
1.3467570193484));
#88870=CARTESIAN_POINT('Ctrl Pts',(-4.53066650772597,-2.46594686124215,
-1.33042470912548));
#88871=CARTESIAN_POINT('Ctrl Pts',(-4.37212330373612,-0.223580041071285,
-2.79301553794379));
#88872=CARTESIAN_POINT('Ctrl Pts',(-4.21358009974628,2.22290076086175,-1.70576552913832));
#88873=CARTESIAN_POINT('Ctrl Pts',(-4.05503689575642,2.64001829300782,0.938737043143364));
#88874=CARTESIAN_POINT('Ctrl Pts',(-3.89649369176657,0.646971487662433,
2.7262339822803));
#88875=CARTESIAN_POINT('Ctrl Pts',(-3.73795048777672,-1.93671805526808,
2.02485728470756));
#88876=CARTESIAN_POINT('Ctrl Pts',(-3.57940728378687,-2.75231044083283,
-0.525081917648047));
#88877=CARTESIAN_POINT('Ctrl Pts',(-3.42086407979702,-1.05522311535154,
-2.59565560789489));
#88878=CARTESIAN_POINT('Ctrl Pts',(-3.26232087580717,1.60521408013114,-2.29656519618435));
#88879=CARTESIAN_POINT('Ctrl Pts',(-3.10377767181731,2.80019550906176,0.0991393121454807));
#88880=CARTESIAN_POINT('Ctrl Pts',(-2.94523446782747,1.43878146837926,2.40433608377855));
#88881=CARTESIAN_POINT('Ctrl Pts',(-2.78669126383761,-1.23614652569664,
2.51453101646264));
#88882=CARTESIAN_POINT('Ctrl Pts',(-2.62814805984777,-2.78255266904079,
0.329123235087791));
#88883=CARTESIAN_POINT('Ctrl Pts',(-2.46960485585791,-1.7886713762176,-2.15675245208684));
#88884=CARTESIAN_POINT('Ctrl Pts',(-2.31106165186806,0.838152943427643,
-2.67365418881957));
#88885=CARTESIAN_POINT('Ctrl Pts',(-2.15251844787821,2.69979292454605,-0.749683767780105));
#88886=CARTESIAN_POINT('Ctrl Pts',(-1.99397524388836,2.09670858668745,1.85869814963478));
#88887=CARTESIAN_POINT('Ctrl Pts',(-1.83543203989851,-0.420553593951653,
2.77021160836216));
#88888=CARTESIAN_POINT('Ctrl Pts',(-1.67688883590866,-2.55383998688081,
1.15269966645968));
#88889=CARTESIAN_POINT('Ctrl Pts',(-1.51834563191881,-2.35570945011923,
-1.51714596444729));
#88890=CARTESIAN_POINT('Ctrl Pts',(-1.35980242792896,-0.0068319532377577,
-2.80194755688051));
#88891=CARTESIAN_POINT('Ctrl Pts',(-1.20125922393911,2.34801894891291,-1.52873260592859));
#88892=CARTESIAN_POINT('Ctrl Pts',(-1.04271601994925,2.55978575511233,1.14007459203818));
#88893=CARTESIAN_POINT('Ctrl Pts',(-0.884172815959405,0.433672104903693,
2.76814622563851));
#88894=CARTESIAN_POINT('Ctrl Pts',(-0.725629611969553,-2.08651182541223,
1.86893074466561));
#88895=CARTESIAN_POINT('Ctrl Pts',(-0.567086407979702,-2.70540359932766,
-0.73619943737228));
#88896=CARTESIAN_POINT('Ctrl Pts',(-0.408543203989851,-0.847344309994932,
-2.66988130255231));
#88897=CARTESIAN_POINT('Ctrl Pts',(-0.302847734663285,0.896356686121819,
-2.33280287161008));
#88898=CARTESIAN_POINT('Ctrl Pts',(-0.250000000000001,1.50502666328431,
-1.8330555925294));
#88899=CARTESIAN_POINT('Ctrl Pts',(-15.6774893273369,-1.12236674703449,
2.30288577939267));
#88900=CARTESIAN_POINT('Ctrl Pts',(-15.6246415926736,-1.88704482906504,
1.93020153289759));
#88901=CARTESIAN_POINT('Ctrl Pts',(-15.5189461233471,-3.00292443317721,
0.369830173449262));
#88902=CARTESIAN_POINT('Ctrl Pts',(-15.3604029193572,-1.94066889012877,
-2.32498690366536));
#88903=CARTESIAN_POINT('Ctrl Pts',(-15.2018597153673,0.895842173804579,
-2.88998281809704));
#88904=CARTESIAN_POINT('Ctrl Pts',(-15.0433165113775,2.91319837846674,-0.820239276834098));
#88905=CARTESIAN_POINT('Ctrl Pts',(-14.8847733073877,2.27167712243153,2.00020746789906));
#88906=CARTESIAN_POINT('Ctrl Pts',(-14.7262301033978,-0.444093911548188,
2.99361449420052));
#88907=CARTESIAN_POINT('Ctrl Pts',(-14.567686899408,-2.75424944441119,1.25456008230755));
#88908=CARTESIAN_POINT('Ctrl Pts',(-14.4091436954181,-2.55005279525,-1.63009433402444));
#88909=CARTESIAN_POINT('Ctrl Pts',(-14.2506004914283,-0.0177732714254624,
-3.02643848791117));
#88910=CARTESIAN_POINT('Ctrl Pts',(-14.0920572874384,2.53070531230325,-1.65991545945025));
#88911=CARTESIAN_POINT('Ctrl Pts',(-13.9335140834486,2.76882918371348,1.22204051837825));
#88912=CARTESIAN_POINT('Ctrl Pts',(-13.7749708794587,0.479185444303327,
2.98833313234507));
#88913=CARTESIAN_POINT('Ctrl Pts',(-13.6164276754689,-2.24791948163841,
2.02648324548122));
#88914=CARTESIAN_POINT('Ctrl Pts',(-13.457884471479,-2.92282269097284,-0.785419062188865));
#88915=CARTESIAN_POINT('Ctrl Pts',(-13.2993412674892,-0.92937855482246,
-2.88028215410634));
#88916=CARTESIAN_POINT('Ctrl Pts',(-13.1407980634993,1.91252697475302,-2.34563719770819));
#88917=CARTESIAN_POINT('Ctrl Pts',(-12.9822548595095,3.00842052822964,0.330422171575135));
#88918=CARTESIAN_POINT('Ctrl Pts',(-12.8237116555196,1.35782240024796,2.70482725621207));
#88919=CARTESIAN_POINT('Ctrl Pts',(-12.6651684515298,-1.53237885167518,
2.60990186365609));
#88920=CARTESIAN_POINT('Ctrl Pts',(-12.5066252475399,-3.02361829820073,
0.132306349491674));
#88921=CARTESIAN_POINT('Ctrl Pts',(-12.3480820435501,-1.75449162069573,
-2.4660761644206));
#88922=CARTESIAN_POINT('Ctrl Pts',(-12.1895388395602,1.11637134917872,-2.81309217475004));
#88923=CARTESIAN_POINT('Ctrl Pts',(-12.0309956355704,2.96806016803971,-0.591938672427007));
#88924=CARTESIAN_POINT('Ctrl Pts',(-11.8724524315805,2.11010382699142,2.16961618322949));
#88925=CARTESIAN_POINT('Ctrl Pts',(-11.7139092275907,-0.674239543511815,
2.95045311642237));
#88926=CARTESIAN_POINT('Ctrl Pts',(-11.5553660236008,-2.84304623091236,
1.03771897908273));
#88927=CARTESIAN_POINT('Ctrl Pts',(-11.396822819611,-2.41633732383554,-1.8223848350756));
#88928=CARTESIAN_POINT('Ctrl Pts',(-11.2382796156211,0.216329803549303,
-3.01877027402064));
#88929=CARTESIAN_POINT('Ctrl Pts',(-11.0797364116313,2.65150194400256,-1.45921553978739));
#88930=CARTESIAN_POINT('Ctrl Pts',(-10.9211932076414,2.66602591890011,1.43250771386515));
#88931=CARTESIAN_POINT('Ctrl Pts',(-10.7626500036516,0.246642287488625,
3.01644494940029));
#88932=CARTESIAN_POINT('Ctrl Pts',(-10.6041067996617,-2.39790964981033,
1.84656488160804));
#88933=CARTESIAN_POINT('Ctrl Pts',(-10.4455635956719,-2.85332662985148,
-1.00910836584611));
#88934=CARTESIAN_POINT('Ctrl Pts',(-10.287020391682,-0.703842682812667,
-2.94353155724871));
#88935=CARTESIAN_POINT('Ctrl Pts',(-10.1284771876922,2.08820368165366,-2.19070261208149));
#88936=CARTESIAN_POINT('Ctrl Pts',(-9.96993398370229,2.973856417933,0.562094792870815));
#88937=CARTESIAN_POINT('Ctrl Pts',(-9.81139077971244,1.14457239967333,2.80173634958097));
#88938=CARTESIAN_POINT('Ctrl Pts',(-9.65284757572259,-1.72963149345564,
2.48357553690266));
#88939=CARTESIAN_POINT('Ctrl Pts',(-9.49430437173273,-3.02479475601628,
-0.101927595045291));
#88940=CARTESIAN_POINT('Ctrl Pts',(-9.3357611677429,-1.55851788699347,-2.59437748729385));
#88941=CARTESIAN_POINT('Ctrl Pts',(-9.17721796375303,1.33058406144162,-2.71833011352428));
#88942=CARTESIAN_POINT('Ctrl Pts',(-9.01867475976319,3.004949632011,-0.360624818519741));
#88943=CARTESIAN_POINT('Ctrl Pts',(-8.86013155577333,1.93599237357926,2.32630739157542));
#88944=CARTESIAN_POINT('Ctrl Pts',(-8.70158835178349,-0.900399526230412,
2.88947283147281));
#88945=CARTESIAN_POINT('Ctrl Pts',(-8.54304514779364,-2.91478544323875,
0.814738222092814));
#88946=CARTESIAN_POINT('Ctrl Pts',(-8.38450194380378,-2.26816254901928,
-2.0037991920055));
#88947=CARTESIAN_POINT('Ctrl Pts',(-8.22595873981394,0.449144670263532,
-2.9929987664263));
#88948=CARTESIAN_POINT('Ctrl Pts',(-8.06741553582408,2.75641212903509,-1.24978587188514));
#88949=CARTESIAN_POINT('Ctrl Pts',(-7.90887233183423,2.54725527268193,1.63439992855164));
#88950=CARTESIAN_POINT('Ctrl Pts',(-7.75032912784439,0.0126206557696573,
3.02648529976662));
#88951=CARTESIAN_POINT('Ctrl Pts',(-7.59178592385452,-2.53353579589187,
1.65558718332501));
#88952=CARTESIAN_POINT('Ctrl Pts',(-7.43324271986469,-2.76673947359612,
-1.226753942688));
#88953=CARTESIAN_POINT('Ctrl Pts',(-7.27469951587482,-0.474090644835783,
-2.98914881047008));
#88954=CARTESIAN_POINT('Ctrl Pts',(-7.11615631188499,2.25137199056513,-2.02264596772502));
#88955=CARTESIAN_POINT('Ctrl Pts',(-6.95761310789512,2.92147898456125,0.790400590474505));
#88956=CARTESIAN_POINT('Ctrl Pts',(-6.79906990390528,0.924466401105285,
2.88186301268518));
#88957=CARTESIAN_POINT('Ctrl Pts',(-6.64052669991542,-1.91652365065164,
2.34237265334709));
#88958=CARTESIAN_POINT('Ctrl Pts',(-6.48198349592558,-3.00785273400343,
-0.335551011328845));
#88959=CARTESIAN_POINT('Ctrl Pts',(-6.32344029193572,-1.35320864577052,
-2.70713850987851));
#88960=CARTESIAN_POINT('Ctrl Pts',(-6.16489708794587,1.53682658872223,-2.6072852906522));
#88961=CARTESIAN_POINT('Ctrl Pts',(-6.00635388395602,3.02383948295879,-0.1271508236573));
#88962=CARTESIAN_POINT('Ctrl Pts',(-5.84781067996617,1.75028434754508,2.4690640440038));
#88963=CARTESIAN_POINT('Ctrl Pts',(-5.68926747597632,-1.12116612584954,
2.81118463799518));
#88964=CARTESIAN_POINT('Ctrl Pts',(-5.53072427198646,-2.96906512424789,
0.586877192130376));
#88965=CARTESIAN_POINT('Ctrl Pts',(-5.37218106799662,-2.10640150642318,
-2.17321081452728));
#88966=CARTESIAN_POINT('Ctrl Pts',(-5.21363786400676,0.679269165501129,
-2.94929923057003));
#88967=CARTESIAN_POINT('Ctrl Pts',(-5.05509466001692,2.8448114369941,-1.0328700008654));
#88968=CARTESIAN_POINT('Ctrl Pts',(-4.89655145602706,2.41322659649633,1.82650210634784));
#88969=CARTESIAN_POINT('Ctrl Pts',(-4.73800825203721,-0.221476573475216,
3.01839703783448));
#88970=CARTESIAN_POINT('Ctrl Pts',(-4.57946504804736,-2.65398609165546,
1.45469253676291));
#88971=CARTESIAN_POINT('Ctrl Pts',(-4.42092184405751,-2.66357957936498,
-1.43705127746513));
#88972=CARTESIAN_POINT('Ctrl Pts',(-4.26237864006766,-0.241498809690948,
-3.01686109649935));
#88973=CARTESIAN_POINT('Ctrl Pts',(-4.10383543607781,2.40105460772325,-1.84247369722676));
#88974=CARTESIAN_POINT('Ctrl Pts',(-3.94529223208796,2.85160192416453,1.01397189769554));
#88975=CARTESIAN_POINT('Ctrl Pts',(-3.78674902809811,0.698822861941575,
2.94472734911847));
#88976=CARTESIAN_POINT('Ctrl Pts',(-3.62820582410825,-2.09193585801802,
2.18713898480308));
#88977=CARTESIAN_POINT('Ctrl Pts',(-3.46966262011841,-2.97289369917019,
-0.567164481653337));
#88978=CARTESIAN_POINT('Ctrl Pts',(-3.31111941612855,-1.13979371814545,
-2.80368380232263));
#88979=CARTESIAN_POINT('Ctrl Pts',(-3.15257621213871,1.73386357652194,-2.48062286149818));
#88980=CARTESIAN_POINT('Ctrl Pts',(-2.99403300814886,3.02461650467576,0.107084808473903));
#88981=CARTESIAN_POINT('Ctrl Pts',(-2.835489804159,1.55409226312905,2.5970310209592));
#88982=CARTESIAN_POINT('Ctrl Pts',(-2.67694660016915,-1.33521719169972,
2.7160575000209));
#88983=CARTESIAN_POINT('Ctrl Pts',(-2.5184033961793,-3.00555968348449,0.355500737608286));
#88984=CARTESIAN_POINT('Ctrl Pts',(-2.35986019218945,-1.93202401348097,
-2.32960485865055));
#88985=CARTESIAN_POINT('Ctrl Pts',(-2.2013169881996,0.905326509499033,-2.88793356075652));
#88986=CARTESIAN_POINT('Ctrl Pts',(-2.04277378420975,2.91616717917131,-0.809766993046504));
#88987=CARTESIAN_POINT('Ctrl Pts',(-1.8842305802199,2.26474879209958,2.00766306581188));
#88988=CARTESIAN_POINT('Ctrl Pts',(-1.72568737623005,-0.454258760593834,
2.99222955146585));
#88989=CARTESIAN_POINT('Ctrl Pts',(-1.5671441722402,-2.75851687841923,1.24508250399859));
#88990=CARTESIAN_POINT('Ctrl Pts',(-1.40860096825035,-2.5445072174402,-1.63873726288739));
#88991=CARTESIAN_POINT('Ctrl Pts',(-1.25005776426049,-0.00737949848690254,
-3.02650896994557));
#88992=CARTESIAN_POINT('Ctrl Pts',(-1.09151456027065,2.53620036286428,-1.6512525129636));
#88993=CARTESIAN_POINT('Ctrl Pts',(-0.932971356280792,2.7649391688157,1.23144559602393));
#88994=CARTESIAN_POINT('Ctrl Pts',(-0.774428152290943,0.468428651451106,
2.98999863914054));
#88995=CARTESIAN_POINT('Ctrl Pts',(-0.615884948301092,-2.25373481384429,
2.01871574971051));
#88996=CARTESIAN_POINT('Ctrl Pts',(-0.457341744311241,-2.9222275201339,
-0.795201964221146));
#88997=CARTESIAN_POINT('Ctrl Pts',(-0.298798540321389,-0.915254515929336,
-2.88385829742676));
#88998=CARTESIAN_POINT('Ctrl Pts',(-0.193103070994823,0.968194977153174,
-2.51976479670557));
#88999=CARTESIAN_POINT('Ctrl Pts',(-0.14025533633154,1.62564666324746,-1.97996539213447));
#89000=CARTESIAN_POINT('Ctrl Pts',(-15.5677446636685,-1.20564430054386,
2.47375567929492));
#89001=CARTESIAN_POINT('Ctrl Pts',(-15.5148969290052,-2.0270600933646,2.07341894544524));
#89002=CARTESIAN_POINT('Ctrl Pts',(-15.4092014596786,-3.2257359168828,0.397270893820039));
#89003=CARTESIAN_POINT('Ctrl Pts',(-15.2506582556888,-2.08466296137931,
-2.49749666644138));
#89004=CARTESIAN_POINT('Ctrl Pts',(-15.0921150516989,0.962312019567628,
-3.10441424116905));
#89005=CARTESIAN_POINT('Ctrl Pts',(-14.9335718477091,3.12935235352635,-0.881099526344837));
#89006=CARTESIAN_POINT('Ctrl Pts',(-14.7750286437192,2.44023139724341,2.14861919238924));
#89007=CARTESIAN_POINT('Ctrl Pts',(-14.6164854397294,-0.477044865039856,
3.21573519751427));
#89008=CARTESIAN_POINT('Ctrl Pts',(-14.4579422357395,-2.95860970017535,
1.3476461387692));
#89009=CARTESIAN_POINT('Ctrl Pts',(-14.2993990317497,-2.73926203427042,
-1.75104434299943));
#89010=CARTESIAN_POINT('Ctrl Pts',(-14.1408558277598,-0.0190920155579868,
-3.25099467133857));
#89011=CARTESIAN_POINT('Ctrl Pts',(-13.98231262377,2.71847900358434,-1.78307814122133));
#89012=CARTESIAN_POINT('Ctrl Pts',(-13.8237694197801,2.97427122938555,1.31271368285747));
#89013=CARTESIAN_POINT('Ctrl Pts',(-13.6652262157903,0.514740125145709,
3.21006196829846));
#89014=CARTESIAN_POINT('Ctrl Pts',(-13.5066830118004,-2.41471098308974,
2.17684458446186));
#89015=CARTESIAN_POINT('Ctrl Pts',(-13.3481398078105,-3.13969077236341,
-0.843695715654877));
#89016=CARTESIAN_POINT('Ctrl Pts',(-13.1895966038207,-0.998336738530438,
-3.0939938057073));
#89017=CARTESIAN_POINT('Ctrl Pts',(-13.0310533998308,2.05443296751247,-2.51967917441669));
#89018=CARTESIAN_POINT('Ctrl Pts',(-12.872510195841,3.23163981210485,0.354938890505661));
#89019=CARTESIAN_POINT('Ctrl Pts',(-12.7139669918511,1.4585703312533,2.90552047628297));
#89020=CARTESIAN_POINT('Ctrl Pts',(-12.5554237878613,-1.64607855113099,
2.80355179375173));
#89021=CARTESIAN_POINT('Ctrl Pts',(-12.3968805838714,-3.24796522872561,
0.14212323789162));
#89022=CARTESIAN_POINT('Ctrl Pts',(-12.2383373798816,-1.88467168011957,
-2.64905449149896));
#89023=CARTESIAN_POINT('Ctrl Pts',(-12.0797941758917,1.19920405516649,-3.02181845315109));
#89024=CARTESIAN_POINT('Ctrl Pts',(-11.9212509719019,3.18828478723489,-0.635859435936428));
#89025=CARTESIAN_POINT('Ctrl Pts',(-11.7627077679121,2.26666965970783,2.33059772359595));
#89026=CARTESIAN_POINT('Ctrl Pts',(-11.6041645639222,-0.724266880664566,
3.16937132468987));
#89027=CARTESIAN_POINT('Ctrl Pts',(-11.4456213599323,-3.05399504532621,
1.11471582350691));
#89028=CARTESIAN_POINT('Ctrl Pts',(-11.2870781559425,-2.59562512019457,
-1.95760244644789));
#89029=CARTESIAN_POINT('Ctrl Pts',(-11.1285349519526,0.232381078088869,
-3.24275749004566));
#89030=CARTESIAN_POINT('Ctrl Pts',(-10.9699917479628,2.84823852373938,-1.5674866557283));
#89031=CARTESIAN_POINT('Ctrl Pts',(-10.8114485439729,2.86384015092833,1.53879715812141));
#89032=CARTESIAN_POINT('Ctrl Pts',(-10.6529053399831,0.26494269272453,3.24025963060457));
#89033=CARTESIAN_POINT('Ctrl Pts',(-10.4943621359932,-2.57583014656451,
1.98357660807178));
#89034=CARTESIAN_POINT('Ctrl Pts',(-10.3358189320034,-3.06503823100597,
-1.0839823552578));
#89035=CARTESIAN_POINT('Ctrl Pts',(-10.1772757280135,-0.756066518590962,
-3.16193619852398));
#89036=CARTESIAN_POINT('Ctrl Pts',(-10.0187325240237,2.24314456376451,-2.35324872678314));
#89037=CARTESIAN_POINT('Ctrl Pts',(-9.86018932003384,3.19451110823633,0.603801195269414));
#89038=CARTESIAN_POINT('Ctrl Pts',(-9.70164611604398,1.22949757186952,3.00962004658812));
#89039=CARTESIAN_POINT('Ctrl Pts',(-9.54310291205413,-1.85796697704721,
2.66785228531445));
#89040=CARTESIAN_POINT('Ctrl Pts',(-9.38455970806428,-3.24922897755272,
-0.109490435598857));
#89041=CARTESIAN_POINT('Ctrl Pts',(-9.22601650407443,-1.67415705491464,
-2.78687553714476));
#89042=CARTESIAN_POINT('Ctrl Pts',(-9.06747330008458,1.4293109576796,-2.9200252208351));
#89043=CARTESIAN_POINT('Ctrl Pts',(-8.90893009609472,3.22791138175458,-0.387382518443105));
#89044=CARTESIAN_POINT('Ctrl Pts',(-8.75038689210488,2.07963945588148,2.49891513213177));
#89045=CARTESIAN_POINT('Ctrl Pts',(-8.59184368811503,-0.96720751918243,
3.10386641447293));
#89046=CARTESIAN_POINT('Ctrl Pts',(-8.43330048412516,-3.13105717559277,
0.875190303434115));
#89047=CARTESIAN_POINT('Ctrl Pts',(-8.27475728013534,-2.43645604893188,
-2.15247741583492));
#89048=CARTESIAN_POINT('Ctrl Pts',(-8.11621407614546,0.482470380785634,
-3.21507378386883));
#89049=CARTESIAN_POINT('Ctrl Pts',(-7.95767087215563,2.96093285203063,-1.34251769069233));
#89050=CARTESIAN_POINT('Ctrl Pts',(-7.79912766816575,2.73625694066019,1.75566940474141));
#89051=CARTESIAN_POINT('Ctrl Pts',(-7.64058446417593,0.0135570852736332,
3.25104495654781));
#89052=CARTESIAN_POINT('Ctrl Pts',(-7.48204126018606,-2.72151950386236,
1.77842871494836));
#89053=CARTESIAN_POINT('Ctrl Pts',(-7.32349805619623,-2.97202646661131,
-1.31777683460364));
#89054=CARTESIAN_POINT('Ctrl Pts',(-7.16495485220635,-0.509267300904713,
-3.21093816824387));
#89055=CARTESIAN_POINT('Ctrl Pts',(-7.00641164821653,2.41841966184476,-2.17272258773612));
#89056=CARTESIAN_POINT('Ctrl Pts',(-6.84786844422665,3.13824736540129,0.849046864200083));
#89057=CARTESIAN_POINT('Ctrl Pts',(-6.68932524023682,0.993060112019402,
3.0956919610924));
#89058=CARTESIAN_POINT('Ctrl Pts',(-6.53078203624696,-2.05872618943038,
2.51617240685321));
#89059=CARTESIAN_POINT('Ctrl Pts',(-6.37223883225711,-3.23102988858874,
-0.360448280759603));
#89060=CARTESIAN_POINT('Ctrl Pts',(-6.21369562826727,-1.45361424465813,
-2.90800322073118));
#89061=CARTESIAN_POINT('Ctrl Pts',(-6.0551524242774,1.65085630210701,-2.80074107583137));
#89062=CARTESIAN_POINT('Ctrl Pts',(-5.89660922028756,3.24820282498693,-0.136585181498785));
#89063=CARTESIAN_POINT('Ctrl Pts',(-5.73806601629771,1.88015223501989,2.6522640662656));
#89064=CARTESIAN_POINT('Ctrl Pts',(-5.57952281230785,-1.20435459546967,
3.01976938066863));
#89065=CARTESIAN_POINT('Ctrl Pts',(-5.42097960831801,-3.18936430935001,
0.630422403087696));
#89066=CARTESIAN_POINT('Ctrl Pts',(-5.26243640432815,-2.26269263374579,
-2.33445906994125));
#89067=CARTESIAN_POINT('Ctrl Pts',(-5.10389320033831,0.729669691378021,
-3.16813182262423));
#89068=CARTESIAN_POINT('Ctrl Pts',(-4.94534999634845,3.05589122646074,-1.1095070600019));
#89069=CARTESIAN_POINT('Ctrl Pts',(-4.78680679235861,2.5922835825938,1.96202521169489));
#89070=CARTESIAN_POINT('Ctrl Pts',(-4.62826358836875,-0.237909728900899,
3.24235656041923));
#89071=CARTESIAN_POINT('Ctrl Pts',(-4.46972038437891,-2.85090699059066,
1.56262805417741));
#89072=CARTESIAN_POINT('Ctrl Pts',(-4.31117718038905,-2.8612122974878,-1.54367784580477));
#89073=CARTESIAN_POINT('Ctrl Pts',(-4.1526339763992,-0.259417578310609,
-3.24070665505491));
#89074=CARTESIAN_POINT('Ctrl Pts',(-3.99409077240935,2.57920845458475,-1.9791818653152));
#89075=CARTESIAN_POINT('Ctrl Pts',(-3.8355475684195,3.06318555532124,1.08920675224771));
#89076=CARTESIAN_POINT('Ctrl Pts',(-3.67700436442965,0.750674236220715,
3.16322071595664));
#89077=CARTESIAN_POINT('Ctrl Pts',(-3.5184611604398,-2.24715366076796,2.34942068489859));
#89078=CARTESIAN_POINT('Ctrl Pts',(-3.35991795644995,-3.19347695750756,
-0.609247045658628));
#89079=CARTESIAN_POINT('Ctrl Pts',(-3.2013747524601,-1.22436432093936,-3.01171199675037));
#89080=CARTESIAN_POINT('Ctrl Pts',(-3.04283154847024,1.86251307291274,-2.66468052681201));
#89081=CARTESIAN_POINT('Ctrl Pts',(-2.88428834448039,3.24903750028975,0.115030304802324));
#89082=CARTESIAN_POINT('Ctrl Pts',(-2.72574514049054,1.66940305787883,2.78972595813986));
#89083=CARTESIAN_POINT('Ctrl Pts',(-2.56720193650069,-1.43428785770279,
2.91758398357915));
#89084=CARTESIAN_POINT('Ctrl Pts',(-2.40865873251084,-3.22856669792818,
0.381878240128784));
#89085=CARTESIAN_POINT('Ctrl Pts',(-2.25011552852099,-2.07537665074434,
-2.50245726521425));
#89086=CARTESIAN_POINT('Ctrl Pts',(-2.09157232453114,0.972500075570423,
-3.10221293269348));
#89087=CARTESIAN_POINT('Ctrl Pts',(-1.93302912054129,3.13254143379656,-0.869850218312904));
#89088=CARTESIAN_POINT('Ctrl Pts',(-1.77448591655143,2.43278899751171,2.15662798198898));
#89089=CARTESIAN_POINT('Ctrl Pts',(-1.61594271256159,-0.487963927236016,
3.21424749456954));
#89090=CARTESIAN_POINT('Ctrl Pts',(-1.45739950857173,-2.96319376995764,
1.33746534153751));
#89091=CARTESIAN_POINT('Ctrl Pts',(-1.29885630458188,-2.73330498476118,
-1.7603285613275));
#89092=CARTESIAN_POINT('Ctrl Pts',(-1.14031310059203,-0.00792704373605107,
-3.25107038301062));
#89093=CARTESIAN_POINT('Ctrl Pts',(-0.981769896602184,2.72438177681566,
-1.77377241999862));
#89094=CARTESIAN_POINT('Ctrl Pts',(-0.823226692612331,2.97009258251906,
1.32281660000969));
#89095=CARTESIAN_POINT('Ctrl Pts',(-0.664683488622481,0.50318519799852,
3.21185105264258));
#89096=CARTESIAN_POINT('Ctrl Pts',(-0.506140284632631,-2.42095780227635,
2.1685007547554));
#89097=CARTESIAN_POINT('Ctrl Pts',(-0.347597080642779,-3.13905144094015,
-0.854204491070011));
#89098=CARTESIAN_POINT('Ctrl Pts',(-0.189053876652928,-0.983164721863736,
-3.09783529230121));
#89099=CARTESIAN_POINT('Ctrl Pts',(-0.0833584073263618,1.04003326818453,
-2.70672672180107));
#89100=CARTESIAN_POINT('Ctrl Pts',(-0.0305106726630785,1.7462666632106,
-2.12687519173954));
#89101=CARTESIAN_POINT('Ctrl Pts',(-15.458,-1.28892185405323,2.64462557919717));
#89102=CARTESIAN_POINT('Ctrl Pts',(-15.4051522653367,-2.16707535766416,
2.21663635799288));
#89103=CARTESIAN_POINT('Ctrl Pts',(-15.2994567960101,-3.44854740058839,
0.424711614190816));
#89104=CARTESIAN_POINT('Ctrl Pts',(-15.1409135920203,-2.22865703262986,
-2.6700064292174));
#89105=CARTESIAN_POINT('Ctrl Pts',(-14.9823703880304,1.02878186533068,-3.31884566424105));
#89106=CARTESIAN_POINT('Ctrl Pts',(-14.8238271840406,3.34550632858596,-0.941959775855578));
#89107=CARTESIAN_POINT('Ctrl Pts',(-14.6652839800507,2.60878567205529,2.29703091687943));
#89108=CARTESIAN_POINT('Ctrl Pts',(-14.5067407760609,-0.509995818531524,
3.43785590082803));
#89109=CARTESIAN_POINT('Ctrl Pts',(-14.348197572071,-3.1629699559395,1.44073219523085));
#89110=CARTESIAN_POINT('Ctrl Pts',(-14.1896543680812,-2.92847127329083,
-1.87199435197442));
#89111=CARTESIAN_POINT('Ctrl Pts',(-14.0311111640913,-0.0204107596905135,
-3.47555085476599));
#89112=CARTESIAN_POINT('Ctrl Pts',(-13.8725679601015,2.90625269486543,-1.90624082299241));
#89113=CARTESIAN_POINT('Ctrl Pts',(-13.7140247561117,3.17971327505761,1.40338684733669));
#89114=CARTESIAN_POINT('Ctrl Pts',(-13.5554815521218,0.550294805988092,
3.43179080425185));
#89115=CARTESIAN_POINT('Ctrl Pts',(-13.3969383481319,-2.58150248454107,
2.32720592344252));
#89116=CARTESIAN_POINT('Ctrl Pts',(-13.2383951441421,-3.35655885375399,
-0.901972369120892));
#89117=CARTESIAN_POINT('Ctrl Pts',(-13.0798519401522,-1.06729492223842,
-3.30770545730824));
#89118=CARTESIAN_POINT('Ctrl Pts',(-12.9213087361624,2.19633896027193,-2.6937211511252));
#89119=CARTESIAN_POINT('Ctrl Pts',(-12.7627655321725,3.45485909598007,0.379455609436187));
#89120=CARTESIAN_POINT('Ctrl Pts',(-12.6042223281827,1.55931826225864,3.10621369635386));
#89121=CARTESIAN_POINT('Ctrl Pts',(-12.4456791241928,-1.7597782505868,2.99720172384735));
#89122=CARTESIAN_POINT('Ctrl Pts',(-12.287135920203,-3.47231215925049,0.151940126291566));
#89123=CARTESIAN_POINT('Ctrl Pts',(-12.1285927162131,-2.0148517395434,-2.83203281857732));
#89124=CARTESIAN_POINT('Ctrl Pts',(-11.9700495122233,1.28203676115426,-3.23054473155214));
#89125=CARTESIAN_POINT('Ctrl Pts',(-11.8115063082334,3.40850940643008,-0.679780199445849));
#89126=CARTESIAN_POINT('Ctrl Pts',(-11.6529631042436,2.42323549242424,2.49157926396243));
#89127=CARTESIAN_POINT('Ctrl Pts',(-11.4944199002537,-0.774294217817315,
3.38828953295737));
#89128=CARTESIAN_POINT('Ctrl Pts',(-11.3358766962639,-3.26494385974007,
1.1917126679311));
#89129=CARTESIAN_POINT('Ctrl Pts',(-11.177333492274,-2.7749129165536,-2.09282005782018));
#89130=CARTESIAN_POINT('Ctrl Pts',(-11.0187902882842,0.248432352628435,
-3.46674470607068));
#89131=CARTESIAN_POINT('Ctrl Pts',(-10.8602470842943,3.04497510347621,-1.67575777166922));
#89132=CARTESIAN_POINT('Ctrl Pts',(-10.7017038803045,3.06165438295654,1.64508660237767));
#89133=CARTESIAN_POINT('Ctrl Pts',(-10.5431606763146,0.283243097960434,
3.46407431180885));
#89134=CARTESIAN_POINT('Ctrl Pts',(-10.3846174723248,-2.75375064331868,
2.12058833453552));
#89135=CARTESIAN_POINT('Ctrl Pts',(-10.2260742683349,-3.27674983216047,
-1.15885634466949));
#89136=CARTESIAN_POINT('Ctrl Pts',(-10.0675310643451,-0.808290354369253,
-3.38034083979924));
#89137=CARTESIAN_POINT('Ctrl Pts',(-9.90898786035523,2.39808544587535,-2.51579484148479));
#89138=CARTESIAN_POINT('Ctrl Pts',(-9.75044465636536,3.41516579853967,0.645507597668011));
#89139=CARTESIAN_POINT('Ctrl Pts',(-9.59190145237552,1.31442274406572,3.21750374359528));
#89140=CARTESIAN_POINT('Ctrl Pts',(-9.43335824838566,-1.98630246063877,
2.85212903372624));
#89141=CARTESIAN_POINT('Ctrl Pts',(-9.27481504439582,-3.47366319908915,
-0.11705327615242));
#89142=CARTESIAN_POINT('Ctrl Pts',(-9.11627184040597,-1.78979622283581,
-2.97937358699568));
#89143=CARTESIAN_POINT('Ctrl Pts',(-8.95772863641611,1.52803785391757,-3.12172032814591));
#89144=CARTESIAN_POINT('Ctrl Pts',(-8.79918543242626,3.45087313149815,-0.414140218366475));
#89145=CARTESIAN_POINT('Ctrl Pts',(-8.64064222843643,2.22328653818369,2.67152287268811));
#89146=CARTESIAN_POINT('Ctrl Pts',(-8.48209902444655,-1.03401551213445,
3.31825999747305));
#89147=CARTESIAN_POINT('Ctrl Pts',(-8.32355582045672,-3.3473289079468,0.935642384775419));
#89148=CARTESIAN_POINT('Ctrl Pts',(-8.16501261646686,-2.60474954884449,
-2.30115563966434));
#89149=CARTESIAN_POINT('Ctrl Pts',(-8.00646941247702,0.515796091307738,
-3.43714880131137));
#89150=CARTESIAN_POINT('Ctrl Pts',(-7.84792620848715,3.16545357502616,-1.43524950949952));
#89151=CARTESIAN_POINT('Ctrl Pts',(-7.68938300449731,2.92525860863845,1.87693888093117));
#89152=CARTESIAN_POINT('Ctrl Pts',(-7.53083980050746,0.0144935147776107,
3.47560461332901));
#89153=CARTESIAN_POINT('Ctrl Pts',(-7.37229659651761,-2.90950321183286,
1.9012702465717));
#89154=CARTESIAN_POINT('Ctrl Pts',(-7.21375339252776,-3.1773134596265,-1.40879972651929));
#89155=CARTESIAN_POINT('Ctrl Pts',(-7.0552101885379,-0.544443956973644,
-3.43272752601767));
#89156=CARTESIAN_POINT('Ctrl Pts',(-6.89666698454805,2.5854673331244,-2.32279920774723));
#89157=CARTESIAN_POINT('Ctrl Pts',(-6.7381237805582,3.35501574624132,0.907693137925664));
#89158=CARTESIAN_POINT('Ctrl Pts',(-6.57958057656835,1.06165382293352,3.30952090949962));
#89159=CARTESIAN_POINT('Ctrl Pts',(-6.42103737257851,-2.20092872820912,
2.68997216035933));
#89160=CARTESIAN_POINT('Ctrl Pts',(-6.26249416858865,-3.45420704317407,
-0.385345550190368));
#89161=CARTESIAN_POINT('Ctrl Pts',(-6.1039509645988,-1.55401984354575,-3.10886793158384));
#89162=CARTESIAN_POINT('Ctrl Pts',(-5.94540776060894,1.76488601549179,-2.99419686101054));
#89163=CARTESIAN_POINT('Ctrl Pts',(-5.7868645566191,3.47256616701507,-0.146019539340268));
#89164=CARTESIAN_POINT('Ctrl Pts',(-5.62832135262924,2.01002012249471,2.8354640885274));
#89165=CARTESIAN_POINT('Ctrl Pts',(-5.4697781486394,-1.2875430650898,3.22835412334209));
#89166=CARTESIAN_POINT('Ctrl Pts',(-5.31123494464955,-3.40966349445213,
0.673967614045017));
#89167=CARTESIAN_POINT('Ctrl Pts',(-5.15269174065969,-2.4189837610684,-2.49570732535522));
#89168=CARTESIAN_POINT('Ctrl Pts',(-4.99414853666985,0.780070217254916,
-3.38696441467844));
#89169=CARTESIAN_POINT('Ctrl Pts',(-4.83560533267999,3.26697101592738,-1.18614411913841));
#89170=CARTESIAN_POINT('Ctrl Pts',(-4.67706212869014,2.77134056869127,2.09754831704194));
#89171=CARTESIAN_POINT('Ctrl Pts',(-4.51851892470029,-0.254342884326582,
3.46631608300398));
#89172=CARTESIAN_POINT('Ctrl Pts',(-4.35997572071044,-3.04782788952586,
1.67056357159192));
#89173=CARTESIAN_POINT('Ctrl Pts',(-4.20143251672059,-3.05884501561062,
-1.65030441414442));
#89174=CARTESIAN_POINT('Ctrl Pts',(-4.04288931273074,-0.277336346930273,
-3.46455221361046));
#89175=CARTESIAN_POINT('Ctrl Pts',(-3.88434610874088,2.75736230144626,-2.11589003340364));
#89176=CARTESIAN_POINT('Ctrl Pts',(-3.72580290475104,3.27476918647795,1.16444160679989));
#89177=CARTESIAN_POINT('Ctrl Pts',(-3.56725970076118,0.802525610499856,
3.38171408279482));
#89178=CARTESIAN_POINT('Ctrl Pts',(-3.40871649677134,-2.4023714635179,2.5117023849941));
#89179=CARTESIAN_POINT('Ctrl Pts',(-3.25017329278148,-3.41406021584493,
-0.651329609663918));
#89180=CARTESIAN_POINT('Ctrl Pts',(-3.09163008879163,-1.30893492373327,
-3.21974019117812));
#89181=CARTESIAN_POINT('Ctrl Pts',(-2.93308688480178,1.99116256930354,-2.84873819212584));
#89182=CARTESIAN_POINT('Ctrl Pts',(-2.77454368081193,3.47345849590375,0.122975801130747));
#89183=CARTESIAN_POINT('Ctrl Pts',(-2.61600047682208,1.78471385262861,2.98242089532051));
#89184=CARTESIAN_POINT('Ctrl Pts',(-2.45745727283223,-1.53335852370586,
3.11911046713741));
#89185=CARTESIAN_POINT('Ctrl Pts',(-2.29891406884238,-3.45157371237187,
0.408255742649282));
#89186=CARTESIAN_POINT('Ctrl Pts',(-2.14037086485253,-2.21872928800771,
-2.67530967177796));
#89187=CARTESIAN_POINT('Ctrl Pts',(-1.98182766086268,1.03967364164181,-3.31649230463043));
#89188=CARTESIAN_POINT('Ctrl Pts',(-1.82328445687283,3.34891568842182,-0.929933443579305));
#89189=CARTESIAN_POINT('Ctrl Pts',(-1.66474125288297,2.60082920292383,2.30559289816608));
#89190=CARTESIAN_POINT('Ctrl Pts',(-1.50619804889312,-0.521669093878197,
3.43626543767323));
#89191=CARTESIAN_POINT('Ctrl Pts',(-1.34765484490327,-3.16787066149606,
1.42984817907643));
#89192=CARTESIAN_POINT('Ctrl Pts',(-1.18911164091342,-2.92210275208215,
-1.8819198597676));
#89193=CARTESIAN_POINT('Ctrl Pts',(-1.03056843692357,-0.00847458898519691,
-3.47563179607567));
#89194=CARTESIAN_POINT('Ctrl Pts',(-0.872025232933723,2.91256319076703,
-1.89629232703364));
#89195=CARTESIAN_POINT('Ctrl Pts',(-0.713482028943869,3.17524599622243,
1.41418760399544));
#89196=CARTESIAN_POINT('Ctrl Pts',(-0.554938824954021,0.537941744545933,
3.43370346614461));
#89197=CARTESIAN_POINT('Ctrl Pts',(-0.396395620964168,-2.58818079070841,
2.3182857598003));
#89198=CARTESIAN_POINT('Ctrl Pts',(-0.237852416974318,-3.35587536174639,
-0.913207017918879));
#89199=CARTESIAN_POINT('Ctrl Pts',(-0.0793092129844665,-1.05107492779814,
-3.31181228717566));
#89200=CARTESIAN_POINT('Ctrl Pts',(0.0263862563420996,1.11187155921588,
-2.89368864689656));
#89201=CARTESIAN_POINT('Ctrl Pts',(0.079233991005383,1.86688666317375,-2.27378499134461));
#89202=CARTESIAN_POINT('Ctrl Pts',(-0.2801761170896,-2.94174543957041,-0.0025773274983063));
#89203=CARTESIAN_POINT('Ctrl Pts',(-0.270117411393067,-2.94340878728205,
-0.188616707269291));
#89204=CARTESIAN_POINT('Ctrl Pts',(-0.260058705696534,-2.92767190815943,
-0.374380454857518));
#89205=CARTESIAN_POINT('Ctrl Pts',(-0.25,-2.89371419577505,-0.556479620053392));
#89206=CARTESIAN_POINT('',(-15.458,-1.37702479013096,-1.93106208855769));
#89207=CARTESIAN_POINT('Ctrl Pts',(-15.458,-1.37998566170037,-1.93363955138647));
#89208=CARTESIAN_POINT('Ctrl Pts',(-15.458,-1.43347830229574,-1.9045572974682));
#89209=CARTESIAN_POINT('Ctrl Pts',(-15.458,-1.48566986876101,-1.8733427436734));
#89210=CARTESIAN_POINT('Ctrl Pts',(-15.458,-1.53641663480976,-1.84002474984019));
#89211=CARTESIAN_POINT('Ctrl Pts',(-15.458,-1.60460402297775,-1.79525604524328));
#89212=CARTESIAN_POINT('Ctrl Pts',(-15.458,-1.67018419084743,-1.74669183548175));
#89213=CARTESIAN_POINT('Ctrl Pts',(-15.458,-1.73307230563806,-1.69469097346931));
#89214=CARTESIAN_POINT('Ctrl Pts',(-15.458,-1.76968235674676,-1.66441889070279));
#89215=CARTESIAN_POINT('Ctrl Pts',(-15.458,-1.80537978873803,-1.63298117771037));
#89216=CARTESIAN_POINT('Ctrl Pts',(-15.458,-1.84014472377397,-1.60044134393351));
#89217=CARTESIAN_POINT('Ctrl Pts',(-15.458,-1.85372686908611,-1.58772851273353));
#89218=CARTESIAN_POINT('Ctrl Pts',(-15.458,-1.86716665434422,-1.57484740618035));
#89219=CARTESIAN_POINT('Ctrl Pts',(-15.458,-1.88046277856858,-1.56180161460873));
#89220=CARTESIAN_POINT('Ctrl Pts',(-15.458,-1.89078117069646,-1.55167749191079));
#89221=CARTESIAN_POINT('Ctrl Pts',(-15.458,-1.90101141569677,-1.54145570679727));
#89222=CARTESIAN_POINT('Ctrl Pts',(-15.458,-1.91114679361931,-1.53114448488591));
#89223=CARTESIAN_POINT('Ctrl Pts',(-15.458,-1.97104061151735,-1.47021153771948));
#89224=CARTESIAN_POINT('Ctrl Pts',(-15.458,-2.02768651729067,-1.40609792454873));
#89225=CARTESIAN_POINT('Ctrl Pts',(-15.458,-2.08099125696457,-1.33919592441725));
#89226=CARTESIAN_POINT('Ctrl Pts',(-15.458,-2.12753187286875,-1.28078347722422));
#89227=CARTESIAN_POINT('Ctrl Pts',(-15.458,-2.17152540896558,-1.22024428012911));
#89228=CARTESIAN_POINT('Ctrl Pts',(-15.458,-2.21289384890174,-1.15781096868051));
#89229=CARTESIAN_POINT('Ctrl Pts',(-15.458,-2.23284077791439,-1.12770703356929));
#89230=CARTESIAN_POINT('Ctrl Pts',(-15.458,-2.25217713735731,-1.09716236855975));
#89231=CARTESIAN_POINT('Ctrl Pts',(-15.458,-2.27089265932552,-1.06620124816656));
#89232=CARTESIAN_POINT('Ctrl Pts',(-15.458,-2.28230086503392,-1.04732863371274));
#89233=CARTESIAN_POINT('Ctrl Pts',(-15.458,-2.2934813528384,-1.02829576315832));
#89234=CARTESIAN_POINT('Ctrl Pts',(-15.458,-2.3044146678338,-1.00913842369171));
#89235=CARTESIAN_POINT('Ctrl Pts',(-15.458,-2.34835022708968,-0.932154597315731));
#89236=CARTESIAN_POINT('Ctrl Pts',(-15.458,-2.38834257191954,-0.853093023880235));
#89237=CARTESIAN_POINT('Ctrl Pts',(-15.458,-2.4242944129843,-0.772350635534902));
#89238=CARTESIAN_POINT('Ctrl Pts',(-15.458,-2.46266928377817,-0.686166489505774));
#89239=CARTESIAN_POINT('Ctrl Pts',(-15.458,-2.49644173827623,-0.598066862910968));
#89240=CARTESIAN_POINT('Ctrl Pts',(-15.458,-2.52545351592011,-0.508485325700583));
#89241=CARTESIAN_POINT('Ctrl Pts',(-15.458,-2.54721234915301,-0.441299172792795));
#89242=CARTESIAN_POINT('Ctrl Pts',(-15.458,-2.5662925310425,-0.373278292061055));
#89243=CARTESIAN_POINT('Ctrl Pts',(-15.458,-2.58260842417879,-0.304592361318692));
#89244=CARTESIAN_POINT('Ctrl Pts',(-15.458,-2.59484534403102,-0.25307791326192));
#89245=CARTESIAN_POINT('Ctrl Pts',(-15.458,-2.60552703202891,-0.20118912404049));
#89246=CARTESIAN_POINT('Ctrl Pts',(-15.458,-2.61461037966331,-0.148994900882582));
#89247=CARTESIAN_POINT('Ctrl Pts',(-15.458,-2.6171362359893,-0.134480966807842));
#89248=CARTESIAN_POINT('Ctrl Pts',(-15.458,-2.6195384609721,-0.119943404900011));
#89249=CARTESIAN_POINT('Ctrl Pts',(-15.458,-2.62181603752144,-0.105383677115885));
#89250=CARTESIAN_POINT('Ctrl Pts',(-15.458,-2.62401192290557,-0.0913461715719244));
#89251=CARTESIAN_POINT('Ctrl Pts',(-15.458,-2.626090686319,-0.0772958939545234));
#89252=CARTESIAN_POINT('Ctrl Pts',(-15.458,-2.62805114010171,-0.0632393621128043));
#89253=CARTESIAN_POINT('Ctrl Pts',(-15.458,-2.64083969310654,0.0284550731791334));
#89254=CARTESIAN_POINT('Ctrl Pts',(-15.458,-2.64860794987797,0.120481249385476));
#89255=CARTESIAN_POINT('Ctrl Pts',(-15.458,-2.65122213956709,0.212444566688069));
#89256=CARTESIAN_POINT('Ctrl Pts',(-15.458,-2.65227583835989,0.24951212793885));
#89257=CARTESIAN_POINT('Ctrl Pts',(-15.458,-2.65249170062149,0.286569819973956));
#89258=CARTESIAN_POINT('Ctrl Pts',(-15.458,-2.6518588794726,0.323592979930078));
#89259=CARTESIAN_POINT('Ctrl Pts',(-15.458,-2.65034341185433,0.412255313889691));
#89260=CARTESIAN_POINT('Ctrl Pts',(-15.458,-2.64396453755206,0.500719073352961));
#89261=CARTESIAN_POINT('Ctrl Pts',(-15.458,-2.63296674054628,0.588722862793259));
#89262=CARTESIAN_POINT('Ctrl Pts',(-15.458,-2.62174854388975,0.67849027857141));
#89263=CARTESIAN_POINT('Ctrl Pts',(-15.458,-2.60572434059568,0.767779835098673));
#89264=CARTESIAN_POINT('Ctrl Pts',(-15.458,-2.58509965927721,0.85631746801127));
#89265=CARTESIAN_POINT('Ctrl Pts',(-15.458,-2.58093104674581,0.874212488077799));
#89266=CARTESIAN_POINT('Ctrl Pts',(-15.458,-2.57657432765316,0.892076780351709));
#89267=CARTESIAN_POINT('Ctrl Pts',(-15.458,-2.5720309446835,0.909908055300652));
#89268=CARTESIAN_POINT('Ctrl Pts',(-15.458,-2.56862062286144,0.923292440125721));
#89269=CARTESIAN_POINT('Ctrl Pts',(-15.458,-2.56510534954551,0.936657094581119));
#89270=CARTESIAN_POINT('Ctrl Pts',(-15.458,-2.56148926917185,0.949988846813725));
#89271=CARTESIAN_POINT('Ctrl Pts',(-15.458,-2.53726799609416,1.03928775006344));
#89272=CARTESIAN_POINT('Ctrl Pts',(-15.458,-2.50849153567128,1.12725652713466));
#89273=CARTESIAN_POINT('Ctrl Pts',(-15.458,-2.47545031643021,1.21361290371913));
#89274=CARTESIAN_POINT('Ctrl Pts',(-15.458,-2.44176584027502,1.30165049357576));
#89275=CARTESIAN_POINT('Ctrl Pts',(-15.458,-2.40364877016699,1.38801307200986));
#89276=CARTESIAN_POINT('Ctrl Pts',(-15.458,-2.36135133676212,1.4724048350925));
#89277=CARTESIAN_POINT('Ctrl Pts',(-15.458,-2.31867994269378,1.55754272381856));
#89278=CARTESIAN_POINT('Ctrl Pts',(-15.458,-2.27175365245138,1.64067566687927));
#89279=CARTESIAN_POINT('Ctrl Pts',(-15.458,-2.22077908013504,1.72149066351755));
#89280=CARTESIAN_POINT('Ctrl Pts',(-15.458,-2.19135516133176,1.76813929225768));
#89281=CARTESIAN_POINT('Ctrl Pts',(-15.458,-2.16058144437314,1.81401536176244));
#89282=CARTESIAN_POINT('Ctrl Pts',(-15.458,-2.12849042302997,1.859055511539));
#89283=CARTESIAN_POINT('Ctrl Pts',(-15.458,-2.12030608087635,1.87054233810272));
#89284=CARTESIAN_POINT('Ctrl Pts',(-15.458,-2.11203467242689,1.88197662493571));
#89285=CARTESIAN_POINT('Ctrl Pts',(-15.458,-2.10368112338145,1.89335125942451));
#89286=CARTESIAN_POINT('Ctrl Pts',(-15.458,-2.04549963217281,1.97257425708832));
#89287=CARTESIAN_POINT('Ctrl Pts',(-15.458,-1.983488402854,2.04870207909741));
#89288=CARTESIAN_POINT('Ctrl Pts',(-15.458,-1.91792260118989,2.12142699555156));
#89289=CARTESIAN_POINT('Ctrl Pts',(-15.458,-1.85213864268311,2.1943938893438));
#89290=CARTESIAN_POINT('Ctrl Pts',(-15.458,-1.78277602527643,2.26393609626659));
#89291=CARTESIAN_POINT('Ctrl Pts',(-15.458,-1.71006216878643,2.32972805253332));
#89292=CARTESIAN_POINT('Ctrl Pts',(-15.458,-1.63869844345376,2.3942984016079));
#89293=CARTESIAN_POINT('Ctrl Pts',(-15.458,-1.5641062449556,2.4552572514107));
#89294=CARTESIAN_POINT('Ctrl Pts',(-15.458,-1.48645909468778,2.51227033795963));
#89295=CARTESIAN_POINT('Ctrl Pts',(-15.458,-1.42265110390908,2.55912190286874));
#89296=CARTESIAN_POINT('Ctrl Pts',(-15.458,-1.35677924409571,2.60330862048415));
#89297=CARTESIAN_POINT('Ctrl Pts',(-15.458,-1.28892185405323,2.64462557919717));
#89298=CARTESIAN_POINT('Ctrl Pts',(-15.458,-1.37998566170039,-1.93363955138645));
#89299=CARTESIAN_POINT('Ctrl Pts',(-15.4092014596786,-0.787929274296016,
-2.35116721332258));
#89300=CARTESIAN_POINT('Ctrl Pts',(-15.3075551846939,0.877072683589833,
-2.62661234173148));
#89301=CARTESIAN_POINT('Ctrl Pts',(-15.153061175046,2.69704440340713,-0.759379027323357));
#89302=CARTESIAN_POINT('Ctrl Pts',(-14.9945179710561,2.10312284761966,1.85179574340887));
#89303=CARTESIAN_POINT('Ctrl Pts',(-14.8359747670663,-0.411142958056525,
2.77149379088676));
#89304=CARTESIAN_POINT('Ctrl Pts',(-14.7076054794126,-2.14284336011571,
1.46789272098577));
#89305=CARTESIAN_POINT('Ctrl Pts',(-14.6320839264221,-2.36934237783001,
0.339980147483457));
#89306=CARTESIAN_POINT('Ctrl Pts',(-14.609410108095,-2.36819900096358,0.000905669814256944));
#89307=CARTESIAN_POINT('Origin',(-15.458,-3.51939854619125E-16,0.));
#89308=CARTESIAN_POINT('',(-15.458,-2.942,-3.60291088309151E-16));
#89309=CARTESIAN_POINT('Origin',(-15.458,0.,0.));
#89310=CARTESIAN_POINT('Origin',(-15.458,0.,0.));
#89311=CARTESIAN_POINT('',(-15.458,1.37702479013102,-1.93106208855765));
#89312=CARTESIAN_POINT('Ctrl Pts',(-15.458,1.29201644558798,2.64838508500724));
#89313=CARTESIAN_POINT('Ctrl Pts',(-15.458,1.35598079841149,2.60984876276284));
#89314=CARTESIAN_POINT('Ctrl Pts',(-15.458,1.41827048161202,2.56877727889907));
#89315=CARTESIAN_POINT('Ctrl Pts',(-15.458,1.478712436698,2.52516206076636));
#89316=CARTESIAN_POINT('Ctrl Pts',(-15.458,1.55797887552663,2.46796300068971));
#89317=CARTESIAN_POINT('Ctrl Pts',(-15.458,1.6340690562504,2.40638958112882));
#89318=CARTESIAN_POINT('Ctrl Pts',(-15.458,1.7068062328737,2.34082102500523));
#89319=CARTESIAN_POINT('Ctrl Pts',(-15.458,1.74532859254324,2.30609524076032));
#89320=CARTESIAN_POINT('Ctrl Pts',(-15.458,1.78290977621518,2.27024832065862));
#89321=CARTESIAN_POINT('Ctrl Pts',(-15.458,1.81951847534658,2.23333368924381));
#89322=CARTESIAN_POINT('Ctrl Pts',(-15.458,1.83920400820175,2.21348364794776));
#89323=CARTESIAN_POINT('Ctrl Pts',(-15.458,1.85860828312012,2.19332484796848));
#89324=CARTESIAN_POINT('Ctrl Pts',(-15.458,1.87772598262537,2.17286543604939));
#89325=CARTESIAN_POINT('Ctrl Pts',(-15.458,1.88940700821849,2.16036461636752));
#89326=CARTESIAN_POINT('Ctrl Pts',(-15.458,1.90097975254709,2.14775284477581));
#89327=CARTESIAN_POINT('Ctrl Pts',(-15.458,1.91243540428845,2.13504078826461));
#89328=CARTESIAN_POINT('Ctrl Pts',(-15.458,1.97752404706709,2.06281351356038));
#89329=CARTESIAN_POINT('Ctrl Pts',(-15.458,2.0389078481352,1.98727494961689));
#89330=CARTESIAN_POINT('Ctrl Pts',(-15.458,2.09641417399276,1.90880097474144));
#89331=CARTESIAN_POINT('Ctrl Pts',(-15.458,2.14364962250154,1.84434278958995));
#89332=CARTESIAN_POINT('Ctrl Pts',(-15.458,2.18826826557574,1.77790325975163));
#89333=CARTESIAN_POINT('Ctrl Pts',(-15.458,2.23014995231654,1.70968105891695));
#89334=CARTESIAN_POINT('Ctrl Pts',(-15.458,2.24876201198549,1.67936337661968));
#89335=CARTESIAN_POINT('Ctrl Pts',(-15.458,2.26683325063596,1.64869356154499));
#89336=CARTESIAN_POINT('Ctrl Pts',(-15.458,2.28435161214332,1.61768881004261));
#89337=CARTESIAN_POINT('Ctrl Pts',(-15.458,2.29483893867365,1.59912788738667));
#89338=CARTESIAN_POINT('Ctrl Pts',(-15.458,2.30512810739652,1.58044692881486));
#89339=CARTESIAN_POINT('Ctrl Pts',(-15.458,2.31521636496224,1.56164961846106));
#89340=CARTESIAN_POINT('Ctrl Pts',(-15.458,2.32246704729265,1.54813952267358));
#89341=CARTESIAN_POINT('Ctrl Pts',(-15.458,2.32961371405895,1.53456959807542));
#89342=CARTESIAN_POINT('Ctrl Pts',(-15.458,2.33664916559811,1.52095359722892));
#89343=CARTESIAN_POINT('Ctrl Pts',(-15.458,2.38029635675402,1.43648137985685));
#89344=CARTESIAN_POINT('Ctrl Pts',(-15.458,2.41973243650582,1.35011673909372));
#89345=CARTESIAN_POINT('Ctrl Pts',(-15.458,2.4547939593135,1.26220655296561));
#89346=CARTESIAN_POINT('Ctrl Pts',(-15.458,2.49109107187097,1.17119835750465));
#89347=CARTESIAN_POINT('Ctrl Pts',(-15.458,2.52270054445843,1.0785327617823));
#89348=CARTESIAN_POINT('Ctrl Pts',(-15.458,2.54938259447905,0.98458420023318));
#89349=CARTESIAN_POINT('Ctrl Pts',(-15.458,2.57407579027275,0.897638473683871));
#89350=CARTESIAN_POINT('Ctrl Pts',(-15.458,2.59454836746826,0.809593140210348));
#89351=CARTESIAN_POINT('Ctrl Pts',(-15.458,2.61056092669808,0.720749094404554));
#89352=CARTESIAN_POINT('Ctrl Pts',(-15.458,2.61991094011146,0.668871502068452));
#89353=CARTESIAN_POINT('Ctrl Pts',(-15.458,2.62773935904613,0.61672171671261));
#89354=CARTESIAN_POINT('Ctrl Pts',(-15.458,2.63399052891176,0.564361823102604));
#89355=CARTESIAN_POINT('Ctrl Pts',(-15.458,2.63614843132954,0.546287199720975));
#89356=CARTESIAN_POINT('Ctrl Pts',(-15.458,2.63811861239107,0.528183596397594));
#89357=CARTESIAN_POINT('Ctrl Pts',(-15.458,2.63989627603494,0.510080720039946));
#89358=CARTESIAN_POINT('Ctrl Pts',(-15.458,2.64861266483537,0.421317185226454));
#89359=CARTESIAN_POINT('Ctrl Pts',(-15.458,2.65272106695796,0.332449891189197));
#89360=CARTESIAN_POINT('Ctrl Pts',(-15.458,2.65203956213944,0.24377021736768));
#89361=CARTESIAN_POINT('Ctrl Pts',(-15.458,2.65171699761295,0.201797048259159));
#89362=CARTESIAN_POINT('Ctrl Pts',(-15.458,2.65032064204942,0.159865954417084));
#89363=CARTESIAN_POINT('Ctrl Pts',(-15.458,2.64782714013714,0.118008441338152));
#89364=CARTESIAN_POINT('Ctrl Pts',(-15.458,2.64244816134619,0.02771347345198));
#89365=CARTESIAN_POINT('Ctrl Pts',(-15.458,2.63196657542956,-0.0622406233293999));
#89366=CARTESIAN_POINT('Ctrl Pts',(-15.458,2.6165783453312,-0.151520688076739));
#89367=CARTESIAN_POINT('Ctrl Pts',(-15.458,2.60079370843378,-0.243100642054985));
#89368=CARTESIAN_POINT('Ctrl Pts',(-15.458,2.57984588485276,-0.333972428620849));
#89369=CARTESIAN_POINT('Ctrl Pts',(-15.458,2.55390006101663,-0.423744721287635));
#89370=CARTESIAN_POINT('Ctrl Pts',(-15.458,2.55017192951763,-0.436644019230246));
#89371=CARTESIAN_POINT('Ctrl Pts',(-15.458,2.54634053796955,-0.449520548422734));
#89372=CARTESIAN_POINT('Ctrl Pts',(-15.458,2.54240631011605,-0.46237307584355));
#89373=CARTESIAN_POINT('Ctrl Pts',(-15.458,2.53826834072496,-0.475891196055698));
#89374=CARTESIAN_POINT('Ctrl Pts',(-15.458,2.53401895642664,-0.489375003499241));
#89375=CARTESIAN_POINT('Ctrl Pts',(-15.458,2.52966057660384,-0.50281859601556));
#89376=CARTESIAN_POINT('Ctrl Pts',(-15.458,2.50229503013095,-0.587228691217232));
#89377=CARTESIAN_POINT('Ctrl Pts',(-15.458,2.47061821529643,-0.67011473702423));
#89378=CARTESIAN_POINT('Ctrl Pts',(-15.458,2.43484287744197,-0.751173581138594));
#89379=CARTESIAN_POINT('Ctrl Pts',(-15.458,2.39912112064777,-0.832111022659138));
#89380=CARTESIAN_POINT('Ctrl Pts',(-15.458,2.35931244647116,-0.911227512394363));
#89381=CARTESIAN_POINT('Ctrl Pts',(-15.458,2.31558654972163,-0.988191253045081));
#89382=CARTESIAN_POINT('Ctrl Pts',(-15.458,2.27255883690487,-1.06392609157778));
#89383=CARTESIAN_POINT('Ctrl Pts',(-15.458,2.22573732113999,-1.13757699578186));
#89384=CARTESIAN_POINT('Ctrl Pts',(-15.458,2.17525294284896,-1.20878852905993));
#89385=CARTESIAN_POINT('Ctrl Pts',(-15.458,2.15800223012227,-1.23312179303172));
#89386=CARTESIAN_POINT('Ctrl Pts',(-15.458,2.14032361321456,-1.25716984887907));
#89387=CARTESIAN_POINT('Ctrl Pts',(-15.458,2.12222168617203,-1.28091724550889));
#89388=CARTESIAN_POINT('Ctrl Pts',(-15.458,2.11092470998078,-1.29573742314528));
#89389=CARTESIAN_POINT('Ctrl Pts',(-15.458,2.09946286113177,-1.31044048926918));
#89390=CARTESIAN_POINT('Ctrl Pts',(-15.458,2.08783720440675,-1.3250225466833));
#89391=CARTESIAN_POINT('Ctrl Pts',(-15.458,2.07930116483031,-1.33572929832211));
#89392=CARTESIAN_POINT('Ctrl Pts',(-15.458,2.07068208018384,-1.34636417148749));
#89393=CARTESIAN_POINT('Ctrl Pts',(-15.458,2.06198317460606,-1.35692290862301));
#89394=CARTESIAN_POINT('Ctrl Pts',(-15.458,2.00776228997665,-1.42273625294983));
#89395=CARTESIAN_POINT('Ctrl Pts',(-15.458,1.95041179714208,-1.48563387608283));
#89396=CARTESIAN_POINT('Ctrl Pts',(-15.458,1.8900901408264,-1.54531963924066));
#89397=CARTESIAN_POINT('Ctrl Pts',(-15.458,1.83071592658384,-1.60406794798104));
#89398=CARTESIAN_POINT('Ctrl Pts',(-15.458,1.7684625100101,-1.65970501421417));
#89399=CARTESIAN_POINT('Ctrl Pts',(-15.458,1.70345510229972,-1.7119059984751));
#89400=CARTESIAN_POINT('Ctrl Pts',(-15.458,1.64047369118742,-1.76248010634987));
#89401=CARTESIAN_POINT('Ctrl Pts',(-15.458,1.57490670552085,-1.80982925665588));
#89402=CARTESIAN_POINT('Ctrl Pts',(-15.458,1.50685234912452,-1.8536122879539));
#89403=CARTESIAN_POINT('Ctrl Pts',(-15.458,1.46453142187118,-1.88083961887897));
#89404=CARTESIAN_POINT('Ctrl Pts',(-15.458,1.42124829763283,-1.90668693330214));
#89405=CARTESIAN_POINT('Ctrl Pts',(-15.458,1.37702479013106,-1.93106208855762));
#89406=CARTESIAN_POINT('Origin',(-15.458,0.,0.));
#89407=CARTESIAN_POINT('Origin',(-17.306589891905,0.,0.));
#89408=CARTESIAN_POINT('Ctrl Pts',(-15.458,1.37702479013101,-1.93106208855765));
#89409=CARTESIAN_POINT('Ctrl Pts',(-15.4051522653367,2.01823803108889,-1.47381810153559));
#89410=CARTESIAN_POINT('Ctrl Pts',(-15.2994567960102,2.79847537909562,0.121597510273868));
#89411=CARTESIAN_POINT('Ctrl Pts',(-15.1409135920203,1.4163960290961,2.41971406834469));
#89412=CARTESIAN_POINT('Ctrl Pts',(-14.9823703880305,-1.25998309782399,
2.5017761501444));
#89413=CARTESIAN_POINT('Ctrl Pts',(-14.8709291546587,-2.33223647147471,
0.956512055862881));
#89414=CARTESIAN_POINT('Ctrl Pts',(-14.8123356559502,-2.37508585399071,
0.0869261581971881));
#89415=CARTESIAN_POINT('Ctrl Pts',(-14.806589891905,-2.37447732889499,0.00158904524625127));
#89416=CARTESIAN_POINT('Ctrl Pts',(-15.7872339910054,1.70810875200393,-2.39535560853239));
#89417=CARTESIAN_POINT('Ctrl Pts',(-15.7343862563421,2.50349163590743,-1.82817449339847));
#89418=CARTESIAN_POINT('Ctrl Pts',(-15.6286907870155,3.4713247877303,0.150833719922236));
#89419=CARTESIAN_POINT('Ctrl Pts',(-15.4701475830257,1.75694618640281,3.00149627451039));
#89420=CARTESIAN_POINT('Ctrl Pts',(-15.3116043790358,-1.56292622485423,
3.10328889373875));
#89421=CARTESIAN_POINT('Ctrl Pts',(-15.153061175046,-3.45515176952641,0.376332500485629));
#89422=CARTESIAN_POINT('Ctrl Pts',(-14.9945179710561,-2.19346697899567,
-2.69644503550222));
#89423=CARTESIAN_POINT('Ctrl Pts',(-14.8359747670663,1.07092856027493,-3.30636730605605));
#89424=CARTESIAN_POINT('Ctrl Pts',(-14.6774315630764,3.35752184538448,-0.898407700729471));
#89425=CARTESIAN_POINT('Ctrl Pts',(-14.5188883590866,2.57897675157689,2.33006158656791));
#89426=CARTESIAN_POINT('Ctrl Pts',(-14.3603451550967,-0.554037067026588,
3.43116822011167));
#89427=CARTESIAN_POINT('Ctrl Pts',(-14.2018019511069,-3.1812348231794,1.39993047848449));
#89428=CARTESIAN_POINT('Ctrl Pts',(-14.043258747117,-2.90418145753586,-1.90939854479434));
#89429=CARTESIAN_POINT('Ctrl Pts',(-13.8847155431272,0.0242044611793096,
-3.4755472053722));
#89430=CARTESIAN_POINT('Ctrl Pts',(-13.7261723391373,2.93049093833658,-1.86876081417929));
#89431=CARTESIAN_POINT('Ctrl Pts',(-13.5676291351475,3.16143174166768,1.44408880709405));
#89432=CARTESIAN_POINT('Ctrl Pts',(-13.4090859311576,0.506191123030663,
3.43857616763681));
#89433=CARTESIAN_POINT('Ctrl Pts',(-13.2505427271678,-2.61116860653983,
2.29386979327385));
#89434=CARTESIAN_POINT('Ctrl Pts',(-13.0919995231779,-3.3447020505759,-0.944990889370293));
#89435=CARTESIAN_POINT('Ctrl Pts',(-12.9334563191881,-1.02474079682209,
-3.32113609006922));
#89436=CARTESIAN_POINT('Ctrl Pts',(-12.7749131151982,2.23074185365558,-2.66530112798528));
#89437=CARTESIAN_POINT('Ctrl Pts',(-12.6163699112084,3.44970285607524,0.42377988943034));
#89438=CARTESIAN_POINT('Ctrl Pts',(-12.4578267072185,1.51931035945226,3.12597746418898));
#89439=CARTESIAN_POINT('Ctrl Pts',(-12.2992835032287,-1.79811329678141,
2.9743617379259));
#89440=CARTESIAN_POINT('Ctrl Pts',(-12.1407402992388,-3.47397691061775,
0.10734791350577));
#89441=CARTESIAN_POINT('Ctrl Pts',(-11.982197095249,-1.97832640971397,-2.85766753731015));
#89442=CARTESIAN_POINT('Ctrl Pts',(-11.8236538912591,1.32340694269406,-3.21381910126486));
#89443=CARTESIAN_POINT('Ctrl Pts',(-11.6651106872693,3.41695615859637,-0.63596364452411));
#89444=CARTESIAN_POINT('Ctrl Pts',(-11.5065674832794,2.39104748524451,2.52248509786409));
#89445=CARTESIAN_POINT('Ctrl Pts',(-11.3480242792896,-0.817731436977695,
3.37806963288756));
#89446=CARTESIAN_POINT('Ctrl Pts',(-11.1894810752997,-3.27997494478484,
1.1496971377047));
#89447=CARTESIAN_POINT('Ctrl Pts',(-11.0309378713099,-2.74781546864746,
-2.12827378338047));
#89448=CARTESIAN_POINT('Ctrl Pts',(-10.87239466732,0.292920132913095,-3.46326968958119));
#89449=CARTESIAN_POINT('Ctrl Pts',(-10.7138514633302,3.06623877709696,-1.63652647663751));
#89450=CARTESIAN_POINT('Ctrl Pts',(-10.5553082593403,3.04028160421297,1.68425856506386));
#89451=CARTESIAN_POINT('Ctrl Pts',(-10.3967650553505,0.238745818439147,
3.46742549755881));
#89452=CARTESIAN_POINT('Ctrl Pts',(-10.2382218513606,-2.7807493125031,2.08505932959628));
#89453=CARTESIAN_POINT('Ctrl Pts',(-10.0796786473708,-3.26160186872235,
-1.20082987840549));
#89454=CARTESIAN_POINT('Ctrl Pts',(-9.92113544338089,-0.764824859953005,
-3.39043980635655));
#89455=CARTESIAN_POINT('Ctrl Pts',(-9.76259223939106,2.43018731260948,-2.48479954373748));
#89456=CARTESIAN_POINT('Ctrl Pts',(-9.60404903540119,3.40659712910876,0.689300476479223));
#89457=CARTESIAN_POINT('Ctrl Pts',(-9.44550583141137,1.27300617423425,3.2341141642324));
#89458=CARTESIAN_POINT('Ctrl Pts',(-9.2869626274215,-2.02275630659,2.82639276659792));
#89459=CARTESIAN_POINT('Ctrl Pts',(-9.12841942343164,-3.47187433977975,
-0.161640699409721));
#89460=CARTESIAN_POINT('Ctrl Pts',(-8.96987621944181,-1.75139777002538,
-3.00210675993993));
#89461=CARTESIAN_POINT('Ctrl Pts',(-8.81133301545194,1.56799061974407,-3.10184534806643));
#89462=CARTESIAN_POINT('Ctrl Pts',(-8.6527898114621,3.45590594354905,-0.369801644492143));
#89463=CARTESIAN_POINT('Ctrl Pts',(-8.49424660747225,2.18880476763518,2.69984681715543));
#89464=CARTESIAN_POINT('Ctrl Pts',(-8.3357034034824,-1.07653225999301,3.30471140042836));
#89465=CARTESIAN_POINT('Ctrl Pts',(-8.17716019949254,-3.35906561812389,
0.892590230769289));
#89466=CARTESIAN_POINT('Ctrl Pts',(-8.0186169955027,-2.57499137120645,-2.33440754478286));
#89467=CARTESIAN_POINT('Ctrl Pts',(-7.86007379151284,0.559881883408217,
-3.43024363909593));
#89468=CARTESIAN_POINT('Ctrl Pts',(-7.701530587523,3.18361953164334,-1.39449124223347));
#89469=CARTESIAN_POINT('Ctrl Pts',(-7.54298738353313,2.90092039738697,1.91434061623083));
#89470=CARTESIAN_POINT('Ctrl Pts',(-7.38444417954331,-0.0301296664458408,
3.47550447419172));
#89471=CARTESIAN_POINT('Ctrl Pts',(-7.22590097555343,-2.93367331189794,
1.86375965349199));
#89472=CARTESIAN_POINT('Ctrl Pts',(-7.0673577715636,-3.15896475517418,-1.44947605102469));
#89473=CARTESIAN_POINT('Ctrl Pts',(-6.90881456757374,-0.50032761723165,
-3.43943475332242));
#89474=CARTESIAN_POINT('Ctrl Pts',(-6.75027136358389,2.61507597020796,-2.2894140772188));
#89475=CARTESIAN_POINT('Ctrl Pts',(-6.59172815959404,3.34308592807698,0.950692181739598));
#89476=CARTESIAN_POINT('Ctrl Pts',(-6.43318495560419,1.01907669463965,3.32287854688806));
#89477=CARTESIAN_POINT('Ctrl Pts',(-6.27464175161433,-2.23528302824535,
2.66149374047064));
#89478=CARTESIAN_POINT('Ctrl Pts',(-6.11609854762449,-3.44897528191934,
-0.429661089276792));
#89479=CARTESIAN_POINT('Ctrl Pts',(-5.95755534363462,-1.5139782774571,-3.12856339592352));
#89480=CARTESIAN_POINT('Ctrl Pts',(-5.79901213964479,1.8031820507789,-2.97129157752513));
#89481=CARTESIAN_POINT('Ctrl Pts',(-5.64046893565492,3.4741548915317,-0.10142453642758));
#89482=CARTESIAN_POINT('Ctrl Pts',(-5.48192573166509,1.97345113447355,2.86103648469429));
#89483=CARTESIAN_POINT('Ctrl Pts',(-5.32338252767522,-1.32888466706206,
3.21155798461682));
#89484=CARTESIAN_POINT('Ctrl Pts',(-5.16483932368538,-3.41803552688201,
0.630136718506388));
#89485=CARTESIAN_POINT('Ctrl Pts',(-5.00629611969552,-2.38674310488516,
-2.52655823167527));
#89486=CARTESIAN_POINT('Ctrl Pts',(-4.84775291570568,0.823489947766338,
-3.37667046849267));
#89487=CARTESIAN_POINT('Ctrl Pts',(-4.68920971171582,3.28193044174787,-1.14410302122984));
#89488=CARTESIAN_POINT('Ctrl Pts',(-4.53066650772598,2.74418271036083,2.13295578899264));
#89489=CARTESIAN_POINT('Ctrl Pts',(-4.37212330373612,-0.298824674553444,
3.46276521883943));
#89490=CARTESIAN_POINT('Ctrl Pts',(-4.21358009974627,-3.06902464253253,
1.63129607832356));
#89491=CARTESIAN_POINT('Ctrl Pts',(-4.05503689575642,-3.03740547736332,
-1.68943987855481));
#89492=CARTESIAN_POINT('Ctrl Pts',(-3.89649369176657,-0.232833420739063,
-3.46782752573225));
#89493=CARTESIAN_POINT('Ctrl Pts',(-3.73795048777672,2.78430035827296,-2.08031504609778));
#89494=CARTESIAN_POINT('Ctrl Pts',(-3.57940728378687,3.2595496698979,1.2063892507913));
#89495=CARTESIAN_POINT('Ctrl Pts',(-3.42086407979702,0.759042977753982,
3.39173892683704));
#89496=CARTESIAN_POINT('Ctrl Pts',(-3.26232087580717,-2.43442046921783,
2.48065239393666));
#89497=CARTESIAN_POINT('Ctrl Pts',(-3.10377767181732,-3.40541682692287,
-0.695107807712134));
#89498=CARTESIAN_POINT('Ctrl Pts',(-2.94523446782747,-1.26749021503053,
-3.2362799852487));
#89499=CARTESIAN_POINT('Ctrl Pts',(-2.78669126383761,2.02757271466167,-2.82293978097886));
#89500=CARTESIAN_POINT('Ctrl Pts',(-2.62814805984777,3.47159317035164,0.167560058613843));
#89501=CARTESIAN_POINT('Ctrl Pts',(-2.46960485585791,1.74627754747723,3.00508866211552));
#89502=CARTESIAN_POINT('Ctrl Pts',(-2.31106165186806,-1.57327897331545,
3.09916720949489));
#89503=CARTESIAN_POINT('Ctrl Pts',(-2.15251844787821,-3.45652780504244,
0.363909007418006));
#89504=CARTESIAN_POINT('Ctrl Pts',(-1.99397524388836,-2.18420522486996,
-2.70357546164494));
#89505=CARTESIAN_POINT('Ctrl Pts',(-1.83543203989851,1.08217859867216,-3.30286993770192));
#89506=CARTESIAN_POINT('Ctrl Pts',(-1.67688883590866,3.36055724413934,-0.886863819989433));
#89507=CARTESIAN_POINT('Ctrl Pts',(-1.51834563191881,2.57105590561094,2.33879875418911));
#89508=CARTESIAN_POINT('Ctrl Pts',(-1.35980242792896,-0.565822421296421,
3.42927606449558));
#89509=CARTESIAN_POINT('Ctrl Pts',(-1.20125922393911,-3.18581540308026,
1.38907629785603));
#89510=CARTESIAN_POINT('Ctrl Pts',(-1.04271601994926,-2.89799076133817,
-1.91931309708123));
#89511=CARTESIAN_POINT('Ctrl Pts',(-0.884172815959405,0.0367029694702862,
-3.47539246609865));
#89512=CARTESIAN_POINT('Ctrl Pts',(-0.725629611969554,2.9356051105282,-1.85886066647829));
#89513=CARTESIAN_POINT('Ctrl Pts',(-0.567086407979703,3.15889968948113,
1.45505757261049));
#89514=CARTESIAN_POINT('Ctrl Pts',(-0.408543203989852,0.489518686277904,
3.43994448338358));
#89515=CARTESIAN_POINT('Ctrl Pts',(-0.302847734663285,-1.57463683943972,
2.67024552677286));
#89516=CARTESIAN_POINT('Ctrl Pts',(-0.250000000000001,-2.21686865784453,
1.93412961144453));
#89517=CARTESIAN_POINT('Ctrl Pts',(-15.6774893273369,1.59774743137963,-2.24059110187414));
#89518=CARTESIAN_POINT('Ctrl Pts',(-15.6246415926736,2.34174043430125,-1.71005569611084));
#89519=CARTESIAN_POINT('Ctrl Pts',(-15.5189461233471,3.24704165151874,0.141088316706114));
#89520=CARTESIAN_POINT('Ctrl Pts',(-15.3604029193572,1.64342946730058,2.80756887245516));
#89521=CARTESIAN_POINT('Ctrl Pts',(-15.2018597153674,-1.46194518251082,
2.90278464587397));
#89522=CARTESIAN_POINT('Ctrl Pts',(-15.0433165113775,-3.2319135759424,0.352017566381606));
#89523=CARTESIAN_POINT('Ctrl Pts',(-14.8847733073876,-2.0517465456428,-2.52222706796369));
#89524=CARTESIAN_POINT('Ctrl Pts',(-14.7262301033978,1.00173560633241,-3.09274211273195));
#89525=CARTESIAN_POINT('Ctrl Pts',(-14.567686899408,3.14059154487117,-0.840361361352499));
#89526=CARTESIAN_POINT('Ctrl Pts',(-14.4091436954181,2.41234843834475,2.17951574250036));
#89527=CARTESIAN_POINT('Ctrl Pts',(-14.2506004914283,-0.518240597791176,
3.20947960947053));
#89528=CARTESIAN_POINT('Ctrl Pts',(-14.0920572874384,-2.97569446991427,
1.30948063083483));
#89529=CARTESIAN_POINT('Ctrl Pts',(-13.9335140834486,-2.71654158940082,
-1.78603184185203));
#89530=CARTESIAN_POINT('Ctrl Pts',(-13.7749708794587,0.0226406050737881,
-3.25099125773301));
#89531=CARTESIAN_POINT('Ctrl Pts',(-13.6164276754689,2.74115120826787,-1.74801972486523));
#89532=CARTESIAN_POINT('Ctrl Pts',(-13.457884471479,2.95717087030058,1.35078587912609));
#89533=CARTESIAN_POINT('Ctrl Pts',(-13.2993412674892,0.473485991837778,
3.2164089277099));
#89534=CARTESIAN_POINT('Ctrl Pts',(-13.1407980634993,-2.44246036975315,
2.14566230974626));
#89535=CARTESIAN_POINT('Ctrl Pts',(-12.9822548595095,-3.12860004011352,
-0.883934798880462));
#89536=CARTESIAN_POINT('Ctrl Pts',(-12.8237116555196,-0.95853204547517,
-3.10655668202912));
#89537=CARTESIAN_POINT('Ctrl Pts',(-12.6651684515298,2.0866130816131,-2.49309537586272));
#89538=CARTESIAN_POINT('Ctrl Pts',(-12.5066252475399,3.22681671811049,0.396399368022285));
#89539=CARTESIAN_POINT('Ctrl Pts',(-12.3480820435501,1.42114734874778,2.92400730228622));
#89540=CARTESIAN_POINT('Ctrl Pts',(-12.1895388395602,-1.68193676069604,
2.78218750485857));
#89541=CARTESIAN_POINT('Ctrl Pts',(-12.0309956355704,-3.24952242010339,
0.100412138785985));
#89542=CARTESIAN_POINT('Ctrl Pts',(-11.8724524315805,-1.85050626070654,
-2.67303294483893));
#89543=CARTESIAN_POINT('Ctrl Pts',(-11.7139092275906,1.23790129924616,-3.00617346989206));
#89544=CARTESIAN_POINT('Ctrl Pts',(-11.5553660236008,3.19618579269568,-0.594873879252186));
#89545=CARTESIAN_POINT('Ctrl Pts',(-11.3968228196109,2.23656132747646,2.35950672407564));
#89546=CARTESIAN_POINT('Ctrl Pts',(-11.2382796156211,-0.764897610562968,
3.15981173484154));
#89547=CARTESIAN_POINT('Ctrl Pts',(-11.0797364116312,-3.06805496832172,
1.07541492687576));
#89548=CARTESIAN_POINT('Ctrl Pts',(-10.9211932076414,-2.57027844496784,
-1.99076549820343));
#89549=CARTESIAN_POINT('Ctrl Pts',(-10.7626500036515,0.273994492102586,
-3.23950699521412));
#89550=CARTESIAN_POINT('Ctrl Pts',(-10.6041067996617,2.8681283462518,-1.53079010418083));
#89551=CARTESIAN_POINT('Ctrl Pts',(-10.4455635956718,2.84384827260153,1.57543821080061));
#89552=CARTESIAN_POINT('Ctrl Pts',(-10.287020391682,0.223320393222169,3.24339429543067));
#89553=CARTESIAN_POINT('Ctrl Pts',(-10.1284771876921,-2.60108442518668,
1.95034314075622));
#89554=CARTESIAN_POINT('Ctrl Pts',(-9.9699339837023,-3.05086898115845,-1.12324396880199));
#89555=CARTESIAN_POINT('Ctrl Pts',(-9.81139077971244,-0.715409340307828,
-3.17138266840337));
#89556=CARTESIAN_POINT('Ctrl Pts',(-9.65284757572259,2.27317232110535,-2.32425604273857));
#89557=CARTESIAN_POINT('Ctrl Pts',(-9.49430437173274,3.18649606261496,0.644764605562371));
#89558=CARTESIAN_POINT('Ctrl Pts',(-9.33576116774289,1.19075693665695,3.02515726392043));
#89559=CARTESIAN_POINT('Ctrl Pts',(-9.17721796375304,-1.89206553117273,
2.64377884464544));
#89560=CARTESIAN_POINT('Ctrl Pts',(-9.01867475976319,-3.24755569687704,
-0.151197054628592));
#89561=CARTESIAN_POINT('Ctrl Pts',(-8.86013155577334,-1.63823953545058,
-2.80813991427307));
#89562=CARTESIAN_POINT('Ctrl Pts',(-8.70158835178349,1.46668236561888,-2.90143436803755));
#89563=CARTESIAN_POINT('Ctrl Pts',(-8.54304514779364,3.23261902259859,-0.345908670577368));
#89564=CARTESIAN_POINT('Ctrl Pts',(-8.38450194380379,2.04738556088874,2.52540905967947));
#89565=CARTESIAN_POINT('Ctrl Pts',(-8.22595873981393,-1.00697724965301,
3.09119319556836));
#89566=CARTESIAN_POINT('Ctrl Pts',(-8.06741553582409,-3.14203557407958,
0.834919759536982));
#89567=CARTESIAN_POINT('Ctrl Pts',(-7.90887233183423,-2.40862055436636,
-2.18358090730129));
#89568=CARTESIAN_POINT('Ctrl Pts',(-7.75032912784438,0.52370777916922,-3.20861476585839));
#89569=CARTESIAN_POINT('Ctrl Pts',(-7.59178592385453,2.97792510178615,-1.30439282495681));
#89570=CARTESIAN_POINT('Ctrl Pts',(-7.43324271986468,2.71349122713884,1.79065460485472));
#89571=CARTESIAN_POINT('Ctrl Pts',(-7.27469951587483,-0.0281829813913912,
3.25095128742446));
#89572=CARTESIAN_POINT('Ctrl Pts',(-7.11615631188498,-2.74412796790182,
1.74334169038255));
#89573=CARTESIAN_POINT('Ctrl Pts',(-6.95761310789512,-2.95486327640258,
-1.35582505192015));
#89574=CARTESIAN_POINT('Ctrl Pts',(-6.79906990390528,-0.468001328570138,
-3.21721203996619));
#89575=CARTESIAN_POINT('Ctrl Pts',(-6.64052669991542,2.44611527770728,-2.14149447858588));
#89576=CARTESIAN_POINT('Ctrl Pts',(-6.48198349592558,3.12708833568111,0.889267729367418));
#89577=CARTESIAN_POINT('Ctrl Pts',(-6.32344029193572,0.953233902308082,
3.10818655829041));
#89578=CARTESIAN_POINT('Ctrl Pts',(-6.16489708794588,-2.09086084981154,
2.48953398457857));
#89579=CARTESIAN_POINT('Ctrl Pts',(-6.00635388395601,-3.22613615269721,
-0.40190058212067));
#89580=CARTESIAN_POINT('Ctrl Pts',(-5.84781067996618,-1.41615977386316,
-2.9264261563444));
#89581=CARTESIAN_POINT('Ctrl Pts',(-5.68926747597632,1.68667802126876,-2.77931570826569));
#89582=CARTESIAN_POINT('Ctrl Pts',(-5.53072427198647,3.24968890162733,-0.0948714725370323));
#89583=CARTESIAN_POINT('Ctrl Pts',(-5.37218106799661,1.8459459781815,2.67618422371572));
#89584=CARTESIAN_POINT('Ctrl Pts',(-5.21363786400677,-1.24302510651458,
3.00405844453889));
#89585=CARTESIAN_POINT('Ctrl Pts',(-5.05509466001691,-3.19719542273467,
0.589423432337293));
#89586=CARTESIAN_POINT('Ctrl Pts',(-4.89655145602707,-2.23253505417579,
-2.36331669172368));
#89587=CARTESIAN_POINT('Ctrl Pts',(-4.73800825203721,0.770284062573315,
-3.15850297079745));
#89588=CARTESIAN_POINT('Ctrl Pts',(-4.57946504804737,3.06988412015183,-1.07018224762271));
#89589=CARTESIAN_POINT('Ctrl Pts',(-4.42092184405751,2.56688040007493,1.99514499829777));
#89590=CARTESIAN_POINT('Ctrl Pts',(-4.26237864006767,-0.279517539875905,
3.23903511844931));
#89591=CARTESIAN_POINT('Ctrl Pts',(-4.10383543607781,-2.87073421624609,
1.52589764317013));
#89592=CARTESIAN_POINT('Ctrl Pts',(-3.94529223208797,-2.841157973005,-1.58028475837061));
#89593=CARTESIAN_POINT('Ctrl Pts',(-3.78674902809811,-0.217789996971037,
-3.24377034846635));
#89594=CARTESIAN_POINT('Ctrl Pts',(-3.62820582410826,2.60440603702834,-1.94590538656487));
#89595=CARTESIAN_POINT('Ctrl Pts',(-3.46966262011841,3.04894937539763,1.12844414878998));
#89596=CARTESIAN_POINT('Ctrl Pts',(-3.31111941612856,0.710001026919591,
3.17259785239462));
#89597=CARTESIAN_POINT('Ctrl Pts',(-3.1525762121387,-2.27713197243884,2.32037684129191));
#89598=CARTESIAN_POINT('Ctrl Pts',(-2.99403300814886,-3.18539202003948,
-0.650196723716245));
#89599=CARTESIAN_POINT('Ctrl Pts',(-2.835489804159,-1.18559736491481,-3.02718315071573));
#89600=CARTESIAN_POINT('Ctrl Pts',(-2.67694660016915,1.89657074995108,-2.64054895726446));
#89601=CARTESIAN_POINT('Ctrl Pts',(-2.5184033961793,3.24729269387384,0.156733962599296));
#89602=CARTESIAN_POINT('Ctrl Pts',(-2.35986019218945,1.63345013172275,2.81092915502609));
#89603=CARTESIAN_POINT('Ctrl Pts',(-2.2013169881996,-1.47162903738377,2.89892926464846));
#89604=CARTESIAN_POINT('Ctrl Pts',(-2.04277378420975,-3.2332007054701,0.340396758213354));
#89605=CARTESIAN_POINT('Ctrl Pts',(-1.8842305802199,-2.04308319569681,-2.52889679554445));
#89606=CARTESIAN_POINT('Ctrl Pts',(-1.72568737623005,1.01225877702106,-3.08947071019517));
#89607=CARTESIAN_POINT('Ctrl Pts',(-1.5671441722402,3.1434308257765,-0.829563333546072));
#89608=CARTESIAN_POINT('Ctrl Pts',(-1.40860096825035,2.4049393601572,2.18768839960309));
#89609=CARTESIAN_POINT('Ctrl Pts',(-1.2500577642605,-0.529264497464093,
3.20770970648758));
#89610=CARTESIAN_POINT('Ctrl Pts',(-1.09151456027064,-2.97997909743711,
1.29932774144854));
#89611=CARTESIAN_POINT('Ctrl Pts',(-0.932971356280794,-2.71075087558549,
-1.79530581251172));
#89612=CARTESIAN_POINT('Ctrl Pts',(-0.774428152290943,0.0343315817136276,
-3.25084651620144));
#89613=CARTESIAN_POINT('Ctrl Pts',(-0.615884948301093,2.74593495255419,
-1.73875922810764));
#89614=CARTESIAN_POINT('Ctrl Pts',(-0.457341744311242,2.95480241461973,
1.36104595004296));
#89615=CARTESIAN_POINT('Ctrl Pts',(-0.29879854032139,0.457890765266106,
3.21768883624451));
#89616=CARTESIAN_POINT('Ctrl Pts',(-0.193103070994824,-1.47289917144852,
2.4977203158458));
#89617=CARTESIAN_POINT('Ctrl Pts',(-0.14025533633154,-2.07363623634716,
1.8091650282895));
#89618=CARTESIAN_POINT('Ctrl Pts',(-15.5677446636685,1.48738611075532,-2.0858265952159));
#89619=CARTESIAN_POINT('Ctrl Pts',(-15.5148969290052,2.17998923269507,-1.59193689882322));
#89620=CARTESIAN_POINT('Ctrl Pts',(-15.4092014596786,3.02275851530718,0.131342913489991));
#89621=CARTESIAN_POINT('Ctrl Pts',(-15.2506582556888,1.52991274819834,2.61364147039993));
#89622=CARTESIAN_POINT('Ctrl Pts',(-15.0921150516989,-1.3609641401674,2.70228039800918));
#89623=CARTESIAN_POINT('Ctrl Pts',(-14.9335718477091,-3.0086753823584,0.327702632277589));
#89624=CARTESIAN_POINT('Ctrl Pts',(-14.7750286437192,-1.91002611228993,
-2.34800910042517));
#89625=CARTESIAN_POINT('Ctrl Pts',(-14.6164854397294,0.932542652389897,
-2.87911691940785));
#89626=CARTESIAN_POINT('Ctrl Pts',(-14.4579422357395,2.92366124435786,-0.782315021975532));
#89627=CARTESIAN_POINT('Ctrl Pts',(-14.2993990317497,2.24572012511262,2.0289698984328));
#89628=CARTESIAN_POINT('Ctrl Pts',(-14.1408558277598,-0.482444128555762,
2.98779099882939));
#89629=CARTESIAN_POINT('Ctrl Pts',(-13.98231262377,-2.77015411664915,1.21903078318517));
#89630=CARTESIAN_POINT('Ctrl Pts',(-13.8237694197801,-2.52890172126577,
-1.66266513890972));
#89631=CARTESIAN_POINT('Ctrl Pts',(-13.6652262157903,0.0210767489682646,
-3.02643531009382));
#89632=CARTESIAN_POINT('Ctrl Pts',(-13.5066830118004,2.55181147819917,-1.62727863555117));
#89633=CARTESIAN_POINT('Ctrl Pts',(-13.3481398078105,2.75290999893348,1.25748295115812));
#89634=CARTESIAN_POINT('Ctrl Pts',(-13.1895966038207,0.440780860644896,
2.994241687783));
#89635=CARTESIAN_POINT('Ctrl Pts',(-13.0310533998308,-2.27375213296647,
1.99745482621866));
#89636=CARTESIAN_POINT('Ctrl Pts',(-12.872510195841,-2.91249802965114,-0.822878708390627));
#89637=CARTESIAN_POINT('Ctrl Pts',(-12.7139669918512,-0.892323294128247,
-2.89197727398902));
#89638=CARTESIAN_POINT('Ctrl Pts',(-12.5554237878613,1.94248430957061,-2.32088962374017));
#89639=CARTESIAN_POINT('Ctrl Pts',(-12.3968805838714,3.00393058014573,0.36901884661423));
#89640=CARTESIAN_POINT('Ctrl Pts',(-12.2383373798816,1.32298433804329,2.72203714038347));
#89641=CARTESIAN_POINT('Ctrl Pts',(-12.0797941758917,-1.56576022461067,
2.59001327179123));
#89642=CARTESIAN_POINT('Ctrl Pts',(-11.9212509719019,-3.02506792958903,
0.0934763640662002));
#89643=CARTESIAN_POINT('Ctrl Pts',(-11.7627077679121,-1.72268611169912,
-2.4883983523677));
#89644=CARTESIAN_POINT('Ctrl Pts',(-11.6041645639222,1.15239565579826,-2.79852783851926));
#89645=CARTESIAN_POINT('Ctrl Pts',(-11.4456213599324,2.97541542679498,-0.55378411398026));
#89646=CARTESIAN_POINT('Ctrl Pts',(-11.2870781559425,2.08207516970842,2.19652835028719));
#89647=CARTESIAN_POINT('Ctrl Pts',(-11.1285349519526,-0.712063784148243,
2.94155383679551));
#89648=CARTESIAN_POINT('Ctrl Pts',(-10.9699917479628,-2.8561349918586,1.00113271604682));
#89649=CARTESIAN_POINT('Ctrl Pts',(-10.811448543973,-2.39274142128822,-1.85325721302638));
#89650=CARTESIAN_POINT('Ctrl Pts',(-10.6529053399831,0.25506885129208,-3.01574430084707));
#89651=CARTESIAN_POINT('Ctrl Pts',(-10.4943621359933,2.67001791540662,-1.42505373172415));
#89652=CARTESIAN_POINT('Ctrl Pts',(-10.3358189320034,2.6474149409901,1.46661785653735));
#89653=CARTESIAN_POINT('Ctrl Pts',(-10.1772757280135,0.207894968005185,
3.01936309330255));
#89654=CARTESIAN_POINT('Ctrl Pts',(-10.0187325240237,-2.42141953787024,
1.81562695191615));
#89655=CARTESIAN_POINT('Ctrl Pts',(-9.86018932003382,-2.84013609359455,
-1.04565805919847));
#89656=CARTESIAN_POINT('Ctrl Pts',(-9.70164611604399,-0.665993820662647,
-2.95232553045019));
#89657=CARTESIAN_POINT('Ctrl Pts',(-9.54310291205412,2.11615732960122,-2.16371254173965));
#89658=CARTESIAN_POINT('Ctrl Pts',(-9.38455970806428,2.96639499612116,0.600228734645521));
#89659=CARTESIAN_POINT('Ctrl Pts',(-9.22601650407443,1.10850769907965,2.81620036360846));
#89660=CARTESIAN_POINT('Ctrl Pts',(-9.06747330008458,-1.76137475575546,
2.46116492269297));
#89661=CARTESIAN_POINT('Ctrl Pts',(-8.90893009609472,-3.02323705397431,
-0.140753409847466));
#89662=CARTESIAN_POINT('Ctrl Pts',(-8.75038689210489,-1.52508130087579,
-2.61417306860622));
#89663=CARTESIAN_POINT('Ctrl Pts',(-8.59184368811502,1.36537411149369,-2.70102338800866));
#89664=CARTESIAN_POINT('Ctrl Pts',(-8.43330048412517,3.00933210164812,-0.322015696662593));
#89665=CARTESIAN_POINT('Ctrl Pts',(-8.27475728013533,1.9059663541423,2.35097130220351));
#89666=CARTESIAN_POINT('Ctrl Pts',(-8.11621407614547,-0.937422239313005,
2.87767499070837));
#89667=CARTESIAN_POINT('Ctrl Pts',(-7.95767087215562,-2.92500553003527,
0.777249288304674));
#89668=CARTESIAN_POINT('Ctrl Pts',(-7.79912766816577,-2.24224973752628,
-2.03275426981972));
#89669=CARTESIAN_POINT('Ctrl Pts',(-7.64058446417592,0.487533674930223,
-2.98698589262086));
#89670=CARTESIAN_POINT('Ctrl Pts',(-7.48204126018606,2.77223067192896,-1.21429440768016));
#89671=CARTESIAN_POINT('Ctrl Pts',(-7.32349805619622,2.5260620568907,1.66696859347862));
#89672=CARTESIAN_POINT('Ctrl Pts',(-7.16495485220636,-0.0262362963369388,
3.0263981006572));
#89673=CARTESIAN_POINT('Ctrl Pts',(-7.00641164821652,-2.55458262390571,
1.62292372727311));
#89674=CARTESIAN_POINT('Ctrl Pts',(-6.84786844422666,-2.75076179763098,
-1.26217405281561));
#89675=CARTESIAN_POINT('Ctrl Pts',(-6.68932524023683,-0.435675039908627,
-2.99498932660997));
#89676=CARTESIAN_POINT('Ctrl Pts',(-6.53078203624695,2.27715458520661,-1.99357487995296));
#89677=CARTESIAN_POINT('Ctrl Pts',(-6.37223883225713,2.91109074328524,0.827843276995237));
#89678=CARTESIAN_POINT('Ctrl Pts',(-6.21369562826725,0.887391109976515,
2.89349456969276));
#89679=CARTESIAN_POINT('Ctrl Pts',(-6.05515242427742,-1.94643867137773,
2.31757422868649));
#89680=CARTESIAN_POINT('Ctrl Pts',(-5.89660922028755,-3.00329702347508,
-0.374140074964546));
#89681=CARTESIAN_POINT('Ctrl Pts',(-5.73806601629772,-1.31834127026923,
-2.72428891676528));
#89682=CARTESIAN_POINT('Ctrl Pts',(-5.57952281230786,1.57017399175861,-2.58733983900626));
#89683=CARTESIAN_POINT('Ctrl Pts',(-5.42097960831801,3.02522291172297,-0.0883184086464839));
#89684=CARTESIAN_POINT('Ctrl Pts',(-5.26243640432816,1.71844082188944,2.49133196273716));
#89685=CARTESIAN_POINT('Ctrl Pts',(-5.10389320033831,-1.15716554596711,
2.79655890446096));
#89686=CARTESIAN_POINT('Ctrl Pts',(-4.94534999634845,-2.97635531858733,
0.548710146168202));
#89687=CARTESIAN_POINT('Ctrl Pts',(-4.78680679235861,-2.07832700346642,
-2.20007515177209));
#89688=CARTESIAN_POINT('Ctrl Pts',(-4.62826358836875,0.717078177380293,
-2.94033547310223));
#89689=CARTESIAN_POINT('Ctrl Pts',(-4.4697203843789,2.85783779855579,-0.996261474015594));
#89690=CARTESIAN_POINT('Ctrl Pts',(-4.31117718038905,2.38957808978902,1.8573342076029));
#89691=CARTESIAN_POINT('Ctrl Pts',(-4.1526339763992,-0.260210405198368,
3.01530501805919));
#89692=CARTESIAN_POINT('Ctrl Pts',(-3.99409077240935,-2.67244378995965,
1.42049920801671));
#89693=CARTESIAN_POINT('Ctrl Pts',(-3.8355475684195,-2.64491046864669,-1.47112963818641));
#89694=CARTESIAN_POINT('Ctrl Pts',(-3.67700436442965,-0.202746573203009,
-3.01971317120046));
#89695=CARTESIAN_POINT('Ctrl Pts',(-3.5184611604398,2.42451171578371,-1.81149572703197));
#89696=CARTESIAN_POINT('Ctrl Pts',(-3.35991795644994,2.83834908089737,1.05049904678867));
#89697=CARTESIAN_POINT('Ctrl Pts',(-3.2013747524601,0.660959076085197,2.9534567779522));
#89698=CARTESIAN_POINT('Ctrl Pts',(-3.04283154847024,-2.11984347565985,
2.16010128864717));
#89699=CARTESIAN_POINT('Ctrl Pts',(-2.8842883444804,-2.96536721315609,-0.605285639720359));
#89700=CARTESIAN_POINT('Ctrl Pts',(-2.72574514049054,-1.1037045147991,-2.81808631618276));
#89701=CARTESIAN_POINT('Ctrl Pts',(-2.56720193650069,1.76556878524048,-2.45815813355006));
#89702=CARTESIAN_POINT('Ctrl Pts',(-2.40865873251084,3.02299221739605,0.145907866584748));
#89703=CARTESIAN_POINT('Ctrl Pts',(-2.25011552852099,1.52062271596827,2.61676964793666));
#89704=CARTESIAN_POINT('Ctrl Pts',(-2.09157232453114,-1.36997910145209,
2.69869131980204));
#89705=CARTESIAN_POINT('Ctrl Pts',(-1.93302912054129,-3.00987360589777,
0.316884509008699));
#89706=CARTESIAN_POINT('Ctrl Pts',(-1.77448591655144,-1.90196116652366,
-2.35421812944396));
#89707=CARTESIAN_POINT('Ctrl Pts',(-1.61594271256159,0.942338955369951,
-2.87607148268842));
#89708=CARTESIAN_POINT('Ctrl Pts',(-1.45739950857174,2.92630440741367,-0.772262847102708));
#89709=CARTESIAN_POINT('Ctrl Pts',(-1.29885630458189,2.23882281470346,2.03657804501707));
#89710=CARTESIAN_POINT('Ctrl Pts',(-1.14031310059203,-0.492706573631765,
2.98614334847957));
#89711=CARTESIAN_POINT('Ctrl Pts',(-0.981769896602184,-2.77414279179396,
1.20957918504104));
#89712=CARTESIAN_POINT('Ctrl Pts',(-0.823226692612332,-2.52351098983281,
-1.67129852794222));
#89713=CARTESIAN_POINT('Ctrl Pts',(-0.664683488622482,0.031960193956968,
-3.02630056630424));
#89714=CARTESIAN_POINT('Ctrl Pts',(-0.506140284632631,2.55626479458018,
-1.61865778973699));
#89715=CARTESIAN_POINT('Ctrl Pts',(-0.34759708064278,2.75070513975834,1.26703432747543));
#89716=CARTESIAN_POINT('Ctrl Pts',(-0.189053876652929,0.426262844254307,
2.99543318910543));
#89717=CARTESIAN_POINT('Ctrl Pts',(-0.0833584073263626,-1.37116150345731,
2.32519510491873));
#89718=CARTESIAN_POINT('Ctrl Pts',(-0.0305106726630785,-1.9304038148498,
1.68420044513446));
#89719=CARTESIAN_POINT('Ctrl Pts',(-15.458,1.37702479013101,-1.93106208855765));
#89720=CARTESIAN_POINT('Ctrl Pts',(-15.4051522653367,2.01823803108889,-1.47381810153559));
#89721=CARTESIAN_POINT('Ctrl Pts',(-15.2994567960102,2.79847537909562,0.121597510273868));
#89722=CARTESIAN_POINT('Ctrl Pts',(-15.1409135920203,1.4163960290961,2.41971406834469));
#89723=CARTESIAN_POINT('Ctrl Pts',(-14.9823703880305,-1.25998309782399,
2.5017761501444));
#89724=CARTESIAN_POINT('Ctrl Pts',(-14.8238271840406,-2.78543718877439,
0.30338769817357));
#89725=CARTESIAN_POINT('Ctrl Pts',(-14.6652839800508,-1.76830567893707,
-2.17379113288664));
#89726=CARTESIAN_POINT('Ctrl Pts',(-14.5067407760609,0.863349698447385,
-2.66549172608374));
#89727=CARTESIAN_POINT('Ctrl Pts',(-14.348197572071,2.70673094384455,-0.724268682598567));
#89728=CARTESIAN_POINT('Ctrl Pts',(-14.1896543680812,2.07909181188049,1.87842405436525));
#89729=CARTESIAN_POINT('Ctrl Pts',(-14.0311111640913,-0.44664765932035,
2.76610238818825));
#89730=CARTESIAN_POINT('Ctrl Pts',(-13.8725679601015,-2.56461376338402,
1.12858093553551));
#89731=CARTESIAN_POINT('Ctrl Pts',(-13.7140247561116,-2.34126185313073,
-1.53929843596741));
#89732=CARTESIAN_POINT('Ctrl Pts',(-13.5554815521218,0.0195128928627424,
-2.80187936245463));
#89733=CARTESIAN_POINT('Ctrl Pts',(-13.3969383481319,2.36247174813047,-1.50653754623712));
#89734=CARTESIAN_POINT('Ctrl Pts',(-13.2383951441421,2.54864912756637,1.16418002319016));
#89735=CARTESIAN_POINT('Ctrl Pts',(-13.0798519401522,0.408075729452012,
2.77207444785609));
#89736=CARTESIAN_POINT('Ctrl Pts',(-12.9213087361624,-2.10504389617979,
1.84924734269107));
#89737=CARTESIAN_POINT('Ctrl Pts',(-12.7627655321725,-2.69639601918876,
-0.761822617900794));
#89738=CARTESIAN_POINT('Ctrl Pts',(-12.6042223281827,-0.826114542781323,
-2.67739786594892));
#89739=CARTESIAN_POINT('Ctrl Pts',(-12.4456791241928,1.79835553752813,-2.1486838716176));
#89740=CARTESIAN_POINT('Ctrl Pts',(-12.287135920203,2.78104444218098,0.341638325206172));
#89741=CARTESIAN_POINT('Ctrl Pts',(-12.1285927162131,1.22482132733881,2.52006697848072));
#89742=CARTESIAN_POINT('Ctrl Pts',(-11.9700495122233,-1.4495836885253,2.39783903872389));
#89743=CARTESIAN_POINT('Ctrl Pts',(-11.8115063082334,-2.80061343907466,
0.0865405893464179));
#89744=CARTESIAN_POINT('Ctrl Pts',(-11.6529631042436,-1.5948659626917,-2.30376375989648));
#89745=CARTESIAN_POINT('Ctrl Pts',(-11.4944199002537,1.06689001235037,-2.59088220714646));
#89746=CARTESIAN_POINT('Ctrl Pts',(-11.3358766962639,2.75464506089428,-0.512694348708331));
#89747=CARTESIAN_POINT('Ctrl Pts',(-11.177333492274,1.92758901194037,2.03354997649873));
#89748=CARTESIAN_POINT('Ctrl Pts',(-11.0187902882842,-0.659229957733515,
2.7232959387495));
#89749=CARTESIAN_POINT('Ctrl Pts',(-10.8602470842943,-2.64421501539548,
0.926850505217873));
#89750=CARTESIAN_POINT('Ctrl Pts',(-10.7017038803045,-2.2152043976086,-1.71574892784934));
#89751=CARTESIAN_POINT('Ctrl Pts',(-10.5431606763146,0.236143210481572,
-2.79198160648));
#89752=CARTESIAN_POINT('Ctrl Pts',(-10.3846174723248,2.47190748456146,-1.31931735926746));
#89753=CARTESIAN_POINT('Ctrl Pts',(-10.2260742683349,2.45098160937866,1.35779750227409));
#89754=CARTESIAN_POINT('Ctrl Pts',(-10.0675310643451,0.192469542788204,
2.79533189117441));
#89755=CARTESIAN_POINT('Ctrl Pts',(-9.90898786035522,-2.24175465055382,
1.68091076307609));
#89756=CARTESIAN_POINT('Ctrl Pts',(-9.75044465636537,-2.62940320603065,
-0.968072149594963));
#89757=CARTESIAN_POINT('Ctrl Pts',(-9.59190145237552,-0.616578301017466,
-2.733268392497));
#89758=CARTESIAN_POINT('Ctrl Pts',(-9.43335824838566,1.95914233809709,-2.00316904074074));
#89759=CARTESIAN_POINT('Ctrl Pts',(-9.27481504439582,2.74629392962736,0.555692863728672));
#89760=CARTESIAN_POINT('Ctrl Pts',(-9.11627184040596,1.02625846150236,2.60724346329648));
#89761=CARTESIAN_POINT('Ctrl Pts',(-8.95772863641611,-1.63068398033819,
2.27855100074049));
#89762=CARTESIAN_POINT('Ctrl Pts',(-8.79918543242627,-2.79891841107159,
-0.130309765066336));
#89763=CARTESIAN_POINT('Ctrl Pts',(-8.64064222843641,-1.41192306630101,
-2.42020622293936));
#89764=CARTESIAN_POINT('Ctrl Pts',(-8.48209902444656,1.26406585736851,-2.50061240797977));
#89765=CARTESIAN_POINT('Ctrl Pts',(-8.32355582045671,2.78604518069765,-0.298122722747819));
#89766=CARTESIAN_POINT('Ctrl Pts',(-8.16501261646686,1.76454714739586,2.17653354472756));
#89767=CARTESIAN_POINT('Ctrl Pts',(-8.00646941247701,-0.867867228973001,
2.66415678584837));
#89768=CARTESIAN_POINT('Ctrl Pts',(-7.84792620848716,-2.70797548599095,
0.719578817072367));
#89769=CARTESIAN_POINT('Ctrl Pts',(-7.68938300449731,-2.0758789206862,-1.88192763233816));
#89770=CARTESIAN_POINT('Ctrl Pts',(-7.53083980050746,0.451359570691226,
-2.76535701938333));
#89771=CARTESIAN_POINT('Ctrl Pts',(-7.37229659651761,2.56653624207177,-1.1241959904035));
#89772=CARTESIAN_POINT('Ctrl Pts',(-7.21375339252775,2.33863288664257,1.54328258210251));
#89773=CARTESIAN_POINT('Ctrl Pts',(-7.05521018853791,-0.0242896112824878,
2.80184491388995));
#89774=CARTESIAN_POINT('Ctrl Pts',(-6.89666698454806,-2.36503727990959,
1.50250576416366));
#89775=CARTESIAN_POINT('Ctrl Pts',(-6.7381237805582,-2.54666031885938,-1.16852305371107));
#89776=CARTESIAN_POINT('Ctrl Pts',(-6.57958057656835,-0.403348751247113,
-2.77276661325373));
#89777=CARTESIAN_POINT('Ctrl Pts',(-6.42103737257851,2.10819389270592,-1.84565528132004));
#89778=CARTESIAN_POINT('Ctrl Pts',(-6.26249416858865,2.69509315088937,0.766418824623061));
#89779=CARTESIAN_POINT('Ctrl Pts',(-6.1039509645988,0.821548317644948,2.6788025810951));
#89780=CARTESIAN_POINT('Ctrl Pts',(-5.94540776060894,-1.80201649294392,
2.14561447279441));
#89781=CARTESIAN_POINT('Ctrl Pts',(-5.78686455661911,-2.78045789425295,
-0.346379567808426));
#89782=CARTESIAN_POINT('Ctrl Pts',(-5.62832135262924,-1.2205227666753,-2.52215167718616));
#89783=CARTESIAN_POINT('Ctrl Pts',(-5.4697781486394,1.45366996224847,-2.39536396974682));
#89784=CARTESIAN_POINT('Ctrl Pts',(-5.31123494464955,2.8007569218186,-0.0817653447559351));
#89785=CARTESIAN_POINT('Ctrl Pts',(-5.15269174065969,1.59093566559739,2.30647970175859));
#89786=CARTESIAN_POINT('Ctrl Pts',(-4.99414853666984,-1.07130598541964,
2.58905936438303));
#89787=CARTESIAN_POINT('Ctrl Pts',(-4.83560533268,-2.75551521443999,0.507996859999107));
#89788=CARTESIAN_POINT('Ctrl Pts',(-4.67706212869014,-1.92411895275705,
-2.0368336118205));
#89789=CARTESIAN_POINT('Ctrl Pts',(-4.51851892470029,0.663872292187274,
-2.72216797540702));
#89790=CARTESIAN_POINT('Ctrl Pts',(-4.35997572071044,2.64579147695974,-0.922340700408471));
#89791=CARTESIAN_POINT('Ctrl Pts',(-4.20143251672059,2.21227577950313,1.71952341690803));
#89792=CARTESIAN_POINT('Ctrl Pts',(-4.04288931273074,-0.24090327052083,
2.79157491766907));
#89793=CARTESIAN_POINT('Ctrl Pts',(-3.88434610874089,-2.47415336367322,
1.31510077286328));
#89794=CARTESIAN_POINT('Ctrl Pts',(-3.72580290475104,-2.44866296428837,
-1.36197451800221));
#89795=CARTESIAN_POINT('Ctrl Pts',(-3.56725970076119,-0.187703149434983,
-2.79565599393456));
#89796=CARTESIAN_POINT('Ctrl Pts',(-3.40871649677134,2.24461739453909,-1.67708606749907));
#89797=CARTESIAN_POINT('Ctrl Pts',(-3.25017329278149,2.6277487863971,0.972553944787357));
#89798=CARTESIAN_POINT('Ctrl Pts',(-3.09163008879163,0.611917125250802,
2.73431570350978));
#89799=CARTESIAN_POINT('Ctrl Pts',(-2.93308688480178,-1.96255497888086,
1.99982573600243));
#89800=CARTESIAN_POINT('Ctrl Pts',(-2.77454368081194,-2.7453424062727,-0.560374555724473));
#89801=CARTESIAN_POINT('Ctrl Pts',(-2.61600047682208,-1.02181166468338,
-2.60898948164979));
#89802=CARTESIAN_POINT('Ctrl Pts',(-2.45745727283223,1.63456682052989,-2.27576730983566));
#89803=CARTESIAN_POINT('Ctrl Pts',(-2.29891406884238,2.79869174091825,0.135081770570203));
#89804=CARTESIAN_POINT('Ctrl Pts',(-2.14037086485253,1.40779530021379,2.42261014084723));
#89805=CARTESIAN_POINT('Ctrl Pts',(-1.98182766086268,-1.26832916552041,
2.49845337495562));
#89806=CARTESIAN_POINT('Ctrl Pts',(-1.82328445687283,-2.78654650632543,
0.293372259804046));
#89807=CARTESIAN_POINT('Ctrl Pts',(-1.66474125288298,-1.76083913735052,
-2.17953946334347));
#89808=CARTESIAN_POINT('Ctrl Pts',(-1.50619804889313,0.872419133718849,
-2.66267225518167));
#89809=CARTESIAN_POINT('Ctrl Pts',(-1.34765484490327,2.70917798905082,-0.714962360659344));
#89810=CARTESIAN_POINT('Ctrl Pts',(-1.18911164091343,2.07270626924971,1.88546769043105));
#89811=CARTESIAN_POINT('Ctrl Pts',(-1.03056843692357,-0.456148649799437,
2.76457699047157));
#89812=CARTESIAN_POINT('Ctrl Pts',(-0.872025232933722,-2.56830648615081,
1.11983062863355));
#89813=CARTESIAN_POINT('Ctrl Pts',(-0.713482028943871,-2.33627110408012,
-1.54729124337272));
#89814=CARTESIAN_POINT('Ctrl Pts',(-0.55493882495402,0.029588806200308,
-2.80175461640703));
#89815=CARTESIAN_POINT('Ctrl Pts',(-0.396395620964169,2.36659463660617,
-1.49855635136634));
#89816=CARTESIAN_POINT('Ctrl Pts',(-0.237852416974319,2.54660786489694,
1.17302270490791));
#89817=CARTESIAN_POINT('Ctrl Pts',(-0.0793092129844672,0.394634923242509,
2.77317754196636));
#89818=CARTESIAN_POINT('Ctrl Pts',(0.0263862563420988,-1.26942383546611,
2.15266989399166));
#89819=CARTESIAN_POINT('Ctrl Pts',(0.079233991005383,-1.78717139335243,
1.55923586197943));
#89820=CARTESIAN_POINT('Origin',(-0.25,0.,0.));
#89821=CARTESIAN_POINT('Origin',(-0.25,0.,0.));
#89822=CARTESIAN_POINT('',(0.,-3.90907258287835E-16,3.192));
#89823=CARTESIAN_POINT('Origin',(-0.25,-3.90907258287835E-16,3.192));
#89824=CARTESIAN_POINT('Origin',(0.,0.,0.));
#89825=CARTESIAN_POINT('Origin',(-7.7,0.,0.));
#89826=CARTESIAN_POINT('Origin',(0.,5.,0.));
#89827=CARTESIAN_POINT('',(0.,-5.,-6.12323399573677E-16));
#89828=CARTESIAN_POINT('Origin',(0.,0.,0.));
#89829=CARTESIAN_POINT('Origin',(0.3,4.70738105939836,-0.830038289247927));
#89830=CARTESIAN_POINT('',(0.3,4.90726077320404,-0.958536229765423));
#89831=CARTESIAN_POINT('',(5.4,4.90726077320404,-0.958536229765423));
#89832=CARTESIAN_POINT('',(2.7,4.90726077320404,-0.958536229765423));
#89833=CARTESIAN_POINT('',(0.3,4.70738105939836,-0.830038289247927));
#89834=CARTESIAN_POINT('',(0.3,5.0904382363941,-1.07629668839819));
#89835=CARTESIAN_POINT('',(5.4,4.70738105939836,-0.830038289247927));
#89836=CARTESIAN_POINT('',(0.3,4.70738105939836,-0.830038289247927));
#89837=CARTESIAN_POINT('',(5.4,5.0904382363941,-1.07629668839819));
#89838=CARTESIAN_POINT('Origin',(5.4,4.91419068753092,-0.866504406557983));
#89839=CARTESIAN_POINT('',(5.4,4.9391554355392,-0.777652611121163));
#89840=CARTESIAN_POINT('Origin',(5.4,0.,0.));
#89841=CARTESIAN_POINT('',(5.4,4.70738105939836,-0.830038289247927));
#89842=CARTESIAN_POINT('Origin',(0.3,5.15156239493286,-0.72964435933789));
#89843=CARTESIAN_POINT('',(0.3,4.9391554355392,-0.777652611121163));
#89844=CARTESIAN_POINT('',(2.7,4.9391554355392,-0.777652611121163));
#89845=CARTESIAN_POINT('',(0.3,4.70738105939836,-0.830038289247927));
#89846=CARTESIAN_POINT('Origin',(0.3,4.91419068753092,-0.866504406557983));
#89847=CARTESIAN_POINT('Origin',(0.3,0.,0.));
#89848=CARTESIAN_POINT('Origin',(0.3,4.49173072735664,-1.6348562850967));
#89849=CARTESIAN_POINT('',(0.3,4.66626038597752,-1.79611080121938));
#89850=CARTESIAN_POINT('',(5.4,4.66626038597752,-1.79611080121938));
#89851=CARTESIAN_POINT('',(2.7,4.66626038597752,-1.79611080121938));
#89852=CARTESIAN_POINT('',(0.3,4.49173072735664,-1.6348562850967));
#89853=CARTESIAN_POINT('',(0.3,4.8262060828614,-1.9438906465518));
#89854=CARTESIAN_POINT('',(5.4,4.49173072735664,-1.6348562850967));
#89855=CARTESIAN_POINT('',(0.3,4.49173072735664,-1.6348562850967));
#89856=CARTESIAN_POINT('',(5.4,4.8262060828614,-1.9438906465518));
#89857=CARTESIAN_POINT('Origin',(5.4,4.68906617772168,-1.70668051519509));
#89858=CARTESIAN_POINT('',(5.4,4.72908060747227,-1.62351366117741));
#89859=CARTESIAN_POINT('Origin',(5.4,0.,0.));
#89860=CARTESIAN_POINT('',(5.4,4.49173072735664,-1.6348562850967));
#89861=CARTESIAN_POINT('Origin',(0.3,4.94659717331204,-1.61311884403516));
#89862=CARTESIAN_POINT('',(0.3,4.72908060747227,-1.62351366117741));
#89863=CARTESIAN_POINT('',(2.7,4.72908060747227,-1.62351366117741));
#89864=CARTESIAN_POINT('',(0.3,4.49173072735664,-1.6348562850967));
#89865=CARTESIAN_POINT('Origin',(0.3,4.68906617772168,-1.70668051519509));
#89866=CARTESIAN_POINT('Origin',(0.3,0.,0.));
#89867=CARTESIAN_POINT('Origin',(0.3,4.13960143008962,-2.39));
#89868=CARTESIAN_POINT('',(0.3,4.28347803816477,-2.57911145485419));
#89869=CARTESIAN_POINT('',(5.4,4.28347803816477,-2.57911145485419));
#89870=CARTESIAN_POINT('',(2.7,4.28347803816477,-2.57911145485419));
#89871=CARTESIAN_POINT('',(0.3,4.13960143008962,-2.39));
#89872=CARTESIAN_POINT('',(0.3,4.41533209967908,-2.75242047106606));
#89873=CARTESIAN_POINT('',(5.4,4.13960143008962,-2.39));
#89874=CARTESIAN_POINT('',(0.3,4.13960143008962,-2.39));
#89875=CARTESIAN_POINT('',(5.4,4.41533209967908,-2.75242047106606));
#89876=CARTESIAN_POINT('Origin',(5.4,4.32146676488435,-2.495));
#89877=CARTESIAN_POINT('',(5.4,4.37531505817755,-2.42004507017633));
#89878=CARTESIAN_POINT('Origin',(5.4,0.,0.));
#89879=CARTESIAN_POINT('',(5.4,4.13960143008962,-2.39));
#89880=CARTESIAN_POINT('Origin',(0.3,4.59133209967908,-2.44757952893394));
#89881=CARTESIAN_POINT('',(0.3,4.37531505817755,-2.42004507017633));
#89882=CARTESIAN_POINT('',(2.7,4.37531505817755,-2.42004507017633));
#89883=CARTESIAN_POINT('',(0.3,4.13960143008962,-2.39));
#89884=CARTESIAN_POINT('Origin',(0.3,4.32146676488435,-2.495));
#89885=CARTESIAN_POINT('Origin',(0.3,0.,0.));
#89886=CARTESIAN_POINT('Origin',(0.3,3.66169243810871,-3.07252477430166));
#89887=CARTESIAN_POINT('',(0.3,3.77054437770685,-3.28374711202663));
#89888=CARTESIAN_POINT('',(5.4,3.77054437770685,-3.28374711202663));
#89889=CARTESIAN_POINT('',(2.7,3.77054437770685,-3.28374711202663));
#89890=CARTESIAN_POINT('',(0.3,3.66169243810871,-3.07252477430166));
#89891=CARTESIAN_POINT('',(0.3,3.87030048491385,-3.47731939235895));
#89892=CARTESIAN_POINT('',(5.4,3.66169243810871,-3.07252477430166));
#89893=CARTESIAN_POINT('',(0.3,3.66169243810871,-3.07252477430166));
#89894=CARTESIAN_POINT('',(5.4,3.87030048491385,-3.47731939235895));
#89895=CARTESIAN_POINT('Origin',(5.4,3.8225617711637,-3.20751017233583));
#89896=CARTESIAN_POINT('',(5.4,3.88860777485636,-3.14304463431983));
#89897=CARTESIAN_POINT('Origin',(5.4,0.,0.));
#89898=CARTESIAN_POINT('',(5.4,3.66169243810871,-3.07252477430166));
#89899=CARTESIAN_POINT('Origin',(0.3,4.09656172352352,-3.20767174838107));
#89900=CARTESIAN_POINT('',(0.3,3.88860777485636,-3.14304463431983));
#89901=CARTESIAN_POINT('',(2.7,3.88860777485636,-3.14304463431983));
#89902=CARTESIAN_POINT('',(0.3,3.66169243810871,-3.07252477430166));
#89903=CARTESIAN_POINT('Origin',(0.3,3.8225617711637,-3.20751017233583));
#89904=CARTESIAN_POINT('Origin',(0.3,0.,0.));
#89905=CARTESIAN_POINT('Origin',(0.3,3.07252477430166,-3.66169243810872));
#89906=CARTESIAN_POINT('',(0.3,3.14304463431983,-3.88860777485636));
#89907=CARTESIAN_POINT('',(5.4,3.14304463431983,-3.88860777485636));
#89908=CARTESIAN_POINT('',(2.7,3.14304463431983,-3.88860777485636));
#89909=CARTESIAN_POINT('',(0.3,3.07252477430166,-3.66169243810872));
#89910=CARTESIAN_POINT('',(0.3,3.20767174838106,-4.09656172352352));
#89911=CARTESIAN_POINT('',(5.4,3.07252477430166,-3.66169243810872));
#89912=CARTESIAN_POINT('',(0.3,3.07252477430166,-3.66169243810872));
#89913=CARTESIAN_POINT('',(5.4,3.20767174838106,-4.09656172352352));
#89914=CARTESIAN_POINT('Origin',(5.4,3.20751017233583,-3.8225617711637));
#89915=CARTESIAN_POINT('',(5.4,3.28374711202663,-3.77054437770685));
#89916=CARTESIAN_POINT('Origin',(5.4,0.,0.));
#89917=CARTESIAN_POINT('',(5.4,3.07252477430166,-3.66169243810872));
#89918=CARTESIAN_POINT('Origin',(0.3,3.47731939235894,-3.87030048491386));
#89919=CARTESIAN_POINT('',(0.3,3.28374711202663,-3.77054437770685));
#89920=CARTESIAN_POINT('',(2.7,3.28374711202663,-3.77054437770685));
#89921=CARTESIAN_POINT('',(0.3,3.07252477430166,-3.66169243810872));
#89922=CARTESIAN_POINT('Origin',(0.3,3.20751017233583,-3.8225617711637));
#89923=CARTESIAN_POINT('Origin',(0.3,0.,0.));
#89924=CARTESIAN_POINT('Origin',(0.3,2.39,-4.13960143008962));
#89925=CARTESIAN_POINT('',(0.3,2.42004507017632,-4.37531505817756));
#89926=CARTESIAN_POINT('',(5.4,2.42004507017632,-4.37531505817756));
#89927=CARTESIAN_POINT('',(2.7,2.42004507017632,-4.37531505817756));
#89928=CARTESIAN_POINT('',(0.3,2.39,-4.13960143008962));
#89929=CARTESIAN_POINT('',(0.3,2.44757952893394,-4.59133209967908));
#89930=CARTESIAN_POINT('',(5.4,2.39,-4.13960143008962));
#89931=CARTESIAN_POINT('',(0.3,2.39,-4.13960143008962));
#89932=CARTESIAN_POINT('',(5.4,2.44757952893394,-4.59133209967908));
#89933=CARTESIAN_POINT('Origin',(5.4,2.495,-4.32146676488435));
#89934=CARTESIAN_POINT('',(5.4,2.57911145485419,-4.28347803816477));
#89935=CARTESIAN_POINT('Origin',(5.4,0.,0.));
#89936=CARTESIAN_POINT('',(5.4,2.39,-4.13960143008962));
#89937=CARTESIAN_POINT('Origin',(0.3,2.75242047106606,-4.41533209967908));
#89938=CARTESIAN_POINT('',(0.3,2.57911145485419,-4.28347803816477));
#89939=CARTESIAN_POINT('',(2.7,2.57911145485419,-4.28347803816477));
#89940=CARTESIAN_POINT('',(0.3,2.39,-4.13960143008962));
#89941=CARTESIAN_POINT('Origin',(0.3,2.495,-4.32146676488435));
#89942=CARTESIAN_POINT('Origin',(0.3,0.,0.));
#89943=CARTESIAN_POINT('Origin',(0.3,1.63485628509669,-4.49173072735664));
#89944=CARTESIAN_POINT('',(0.3,1.6235136611774,-4.72908060747227));
#89945=CARTESIAN_POINT('',(5.4,1.6235136611774,-4.72908060747227));
#89946=CARTESIAN_POINT('',(2.7,1.6235136611774,-4.72908060747228));
#89947=CARTESIAN_POINT('',(0.3,1.63485628509669,-4.49173072735664));
#89948=CARTESIAN_POINT('',(0.3,1.61311884403515,-4.94659717331204));
#89949=CARTESIAN_POINT('',(5.4,1.63485628509669,-4.49173072735664));
#89950=CARTESIAN_POINT('',(0.3,1.63485628509669,-4.49173072735664));
#89951=CARTESIAN_POINT('',(5.4,1.61311884403515,-4.94659717331204));
#89952=CARTESIAN_POINT('Origin',(5.4,1.70668051519508,-4.68906617772168));
#89953=CARTESIAN_POINT('',(5.4,1.79611080121937,-4.66626038597752));
#89954=CARTESIAN_POINT('Origin',(5.4,0.,0.));
#89955=CARTESIAN_POINT('',(5.4,1.63485628509669,-4.49173072735664));
#89956=CARTESIAN_POINT('Origin',(0.3,1.94389064655179,-4.82620608286141));
#89957=CARTESIAN_POINT('',(0.3,1.79611080121937,-4.66626038597752));
#89958=CARTESIAN_POINT('',(2.7,1.79611080121937,-4.66626038597752));
#89959=CARTESIAN_POINT('',(0.3,1.63485628509669,-4.49173072735664));
#89960=CARTESIAN_POINT('Origin',(0.3,1.70668051519508,-4.68906617772168));
#89961=CARTESIAN_POINT('Origin',(0.3,0.,0.));
#89962=CARTESIAN_POINT('Origin',(0.3,0.830038289247925,-4.70738105939836));
#89963=CARTESIAN_POINT('',(0.3,0.777652611121161,-4.9391554355392));
#89964=CARTESIAN_POINT('',(5.4,0.777652611121161,-4.9391554355392));
#89965=CARTESIAN_POINT('',(2.7,0.777652611121161,-4.9391554355392));
#89966=CARTESIAN_POINT('',(0.3,0.830038289247925,-4.70738105939836));
#89967=CARTESIAN_POINT('',(0.3,0.729644359337887,-5.15156239493286));
#89968=CARTESIAN_POINT('',(5.4,0.830038289247925,-4.70738105939836));
#89969=CARTESIAN_POINT('',(0.3,0.830038289247925,-4.70738105939836));
#89970=CARTESIAN_POINT('',(5.4,0.729644359337887,-5.15156239493286));
#89971=CARTESIAN_POINT('Origin',(5.4,0.866504406557981,-4.91419068753092));
#89972=CARTESIAN_POINT('',(5.4,0.958536229765421,-4.90726077320404));
#89973=CARTESIAN_POINT('Origin',(5.4,0.,0.));
#89974=CARTESIAN_POINT('',(5.4,0.830038289247925,-4.70738105939836));
#89975=CARTESIAN_POINT('Origin',(0.3,1.07629668839818,-5.0904382363941));
#89976=CARTESIAN_POINT('',(0.3,0.958536229765421,-4.90726077320404));
#89977=CARTESIAN_POINT('',(2.7,0.958536229765421,-4.90726077320404));
#89978=CARTESIAN_POINT('',(0.3,0.830038289247925,-4.70738105939836));
#89979=CARTESIAN_POINT('Origin',(0.3,0.866504406557981,-4.91419068753092));
#89980=CARTESIAN_POINT('Origin',(0.3,0.,0.));
#89981=CARTESIAN_POINT('Origin',(0.3,-8.78071754988652E-16,-4.78));
#89982=CARTESIAN_POINT('',(0.3,-0.0918370200127877,-4.99915652503051));
#89983=CARTESIAN_POINT('',(5.4,-0.0918370200127877,-4.99915652503051));
#89984=CARTESIAN_POINT('',(2.7,-0.0918370200127877,-4.99915652503051));
#89985=CARTESIAN_POINT('',(0.3,-8.78071754988652E-16,-4.78));
#89986=CARTESIAN_POINT('',(0.3,-0.176000000000001,-5.2));
#89987=CARTESIAN_POINT('',(5.4,-8.78071754988652E-16,-4.78));
#89988=CARTESIAN_POINT('',(0.3,-8.78071754988652E-16,-4.78));
#89989=CARTESIAN_POINT('',(5.4,-0.176000000000001,-5.2));
#89990=CARTESIAN_POINT('Origin',(5.4,-9.16648129161794E-16,-4.99));
#89991=CARTESIAN_POINT('',(5.4,0.091837020012786,-4.99915652503051));
#89992=CARTESIAN_POINT('Origin',(5.4,0.,0.));
#89993=CARTESIAN_POINT('',(5.4,-8.78071754988652E-16,-4.78));
#89994=CARTESIAN_POINT('Origin',(0.3,0.175999999999999,-5.2));
#89995=CARTESIAN_POINT('',(0.3,0.091837020012786,-4.99915652503051));
#89996=CARTESIAN_POINT('',(2.7,0.0918370200127863,-4.99915652503051));
#89997=CARTESIAN_POINT('',(0.3,-8.78071754988652E-16,-4.78));
#89998=CARTESIAN_POINT('Origin',(0.3,-9.16648129161794E-16,-4.99));
#89999=CARTESIAN_POINT('Origin',(0.3,0.,0.));
#90000=CARTESIAN_POINT('Origin',(0.3,-0.830038289247927,-4.70738105939836));
#90001=CARTESIAN_POINT('',(0.3,-0.958536229765423,-4.90726077320404));
#90002=CARTESIAN_POINT('',(5.4,-0.958536229765423,-4.90726077320404));
#90003=CARTESIAN_POINT('',(2.7,-0.958536229765423,-4.90726077320404));
#90004=CARTESIAN_POINT('',(0.3,-0.830038289247927,-4.70738105939836));
#90005=CARTESIAN_POINT('',(0.3,-1.07629668839819,-5.0904382363941));
#90006=CARTESIAN_POINT('',(5.4,-0.830038289247927,-4.70738105939836));
#90007=CARTESIAN_POINT('',(0.3,-0.830038289247927,-4.70738105939836));
#90008=CARTESIAN_POINT('',(5.4,-1.07629668839819,-5.0904382363941));
#90009=CARTESIAN_POINT('Origin',(5.4,-0.866504406557982,-4.91419068753092));
#90010=CARTESIAN_POINT('',(5.4,-0.777652611121163,-4.9391554355392));
#90011=CARTESIAN_POINT('Origin',(5.4,0.,0.));
#90012=CARTESIAN_POINT('',(5.4,-0.830038289247927,-4.70738105939836));
#90013=CARTESIAN_POINT('Origin',(0.3,-0.729644359337889,-5.15156239493286));
#90014=CARTESIAN_POINT('',(0.3,-0.777652611121163,-4.9391554355392));
#90015=CARTESIAN_POINT('',(2.7,-0.777652611121163,-4.9391554355392));
#90016=CARTESIAN_POINT('',(0.3,-0.830038289247927,-4.70738105939836));
#90017=CARTESIAN_POINT('Origin',(0.3,-0.866504406557982,-4.91419068753092));
#90018=CARTESIAN_POINT('Origin',(0.3,0.,0.));
#90019=CARTESIAN_POINT('Origin',(0.3,-1.6348562850967,-4.49173072735664));
#90020=CARTESIAN_POINT('',(0.3,-1.79611080121938,-4.66626038597752));
#90021=CARTESIAN_POINT('',(5.4,-1.79611080121938,-4.66626038597752));
#90022=CARTESIAN_POINT('',(2.7,-1.79611080121938,-4.66626038597752));
#90023=CARTESIAN_POINT('',(0.3,-1.6348562850967,-4.49173072735664));
#90024=CARTESIAN_POINT('',(0.3,-1.9438906465518,-4.8262060828614));
#90025=CARTESIAN_POINT('',(5.4,-1.6348562850967,-4.49173072735664));
#90026=CARTESIAN_POINT('',(0.3,-1.6348562850967,-4.49173072735664));
#90027=CARTESIAN_POINT('',(5.4,-1.9438906465518,-4.8262060828614));
#90028=CARTESIAN_POINT('Origin',(5.4,-1.70668051519509,-4.68906617772168));
#90029=CARTESIAN_POINT('',(5.4,-1.62351366117741,-4.72908060747227));
#90030=CARTESIAN_POINT('Origin',(5.4,0.,0.));
#90031=CARTESIAN_POINT('',(5.4,-1.6348562850967,-4.49173072735664));
#90032=CARTESIAN_POINT('Origin',(0.3,-1.61311884403516,-4.94659717331204));
#90033=CARTESIAN_POINT('',(0.3,-1.62351366117741,-4.72908060747227));
#90034=CARTESIAN_POINT('',(2.7,-1.62351366117741,-4.72908060747227));
#90035=CARTESIAN_POINT('',(0.3,-1.6348562850967,-4.49173072735664));
#90036=CARTESIAN_POINT('Origin',(0.3,-1.70668051519509,-4.68906617772168));
#90037=CARTESIAN_POINT('Origin',(0.3,0.,0.));
#90038=CARTESIAN_POINT('Origin',(0.3,-2.39,-4.13960143008962));
#90039=CARTESIAN_POINT('',(0.3,-2.57911145485419,-4.28347803816477));
#90040=CARTESIAN_POINT('',(5.4,-2.57911145485419,-4.28347803816477));
#90041=CARTESIAN_POINT('',(2.7,-2.57911145485419,-4.28347803816477));
#90042=CARTESIAN_POINT('',(0.3,-2.39,-4.13960143008962));
#90043=CARTESIAN_POINT('',(0.3,-2.75242047106606,-4.41533209967908));
#90044=CARTESIAN_POINT('',(5.4,-2.39,-4.13960143008962));
#90045=CARTESIAN_POINT('',(0.3,-2.39,-4.13960143008962));
#90046=CARTESIAN_POINT('',(5.4,-2.75242047106606,-4.41533209967908));
#90047=CARTESIAN_POINT('Origin',(5.4,-2.495,-4.32146676488435));
#90048=CARTESIAN_POINT('',(5.4,-2.42004507017633,-4.37531505817755));
#90049=CARTESIAN_POINT('Origin',(5.4,0.,0.));
#90050=CARTESIAN_POINT('',(5.4,-2.39,-4.13960143008962));
#90051=CARTESIAN_POINT('Origin',(0.3,-2.44757952893394,-4.59133209967908));
#90052=CARTESIAN_POINT('',(0.3,-2.42004507017633,-4.37531505817755));
#90053=CARTESIAN_POINT('',(2.7,-2.42004507017633,-4.37531505817755));
#90054=CARTESIAN_POINT('',(0.3,-2.39,-4.13960143008962));
#90055=CARTESIAN_POINT('Origin',(0.3,-2.495,-4.32146676488435));
#90056=CARTESIAN_POINT('Origin',(0.3,0.,0.));
#90057=CARTESIAN_POINT('Origin',(0.3,-3.07252477430166,-3.66169243810871));
#90058=CARTESIAN_POINT('',(0.3,-3.28374711202663,-3.77054437770685));
#90059=CARTESIAN_POINT('',(5.4,-3.28374711202663,-3.77054437770685));
#90060=CARTESIAN_POINT('',(2.7,-3.28374711202663,-3.77054437770685));
#90061=CARTESIAN_POINT('',(0.3,-3.07252477430166,-3.66169243810871));
#90062=CARTESIAN_POINT('',(0.3,-3.47731939235895,-3.87030048491385));
#90063=CARTESIAN_POINT('',(5.4,-3.07252477430166,-3.66169243810871));
#90064=CARTESIAN_POINT('',(0.3,-3.07252477430166,-3.66169243810871));
#90065=CARTESIAN_POINT('',(5.4,-3.47731939235895,-3.87030048491385));
#90066=CARTESIAN_POINT('Origin',(5.4,-3.20751017233583,-3.8225617711637));
#90067=CARTESIAN_POINT('',(5.4,-3.14304463431983,-3.88860777485636));
#90068=CARTESIAN_POINT('Origin',(5.4,0.,0.));
#90069=CARTESIAN_POINT('',(5.4,-3.07252477430166,-3.66169243810871));
#90070=CARTESIAN_POINT('Origin',(0.3,-3.20767174838107,-4.09656172352352));
#90071=CARTESIAN_POINT('',(0.3,-3.14304463431983,-3.88860777485636));
#90072=CARTESIAN_POINT('',(2.7,-3.14304463431983,-3.88860777485636));
#90073=CARTESIAN_POINT('',(0.3,-3.07252477430166,-3.66169243810871));
#90074=CARTESIAN_POINT('Origin',(0.3,-3.20751017233583,-3.8225617711637));
#90075=CARTESIAN_POINT('Origin',(0.3,0.,0.));
#90076=CARTESIAN_POINT('Origin',(0.3,-3.66169243810872,-3.07252477430166));
#90077=CARTESIAN_POINT('',(0.3,-3.88860777485636,-3.14304463431983));
#90078=CARTESIAN_POINT('',(5.4,-3.88860777485636,-3.14304463431983));
#90079=CARTESIAN_POINT('',(2.7,-3.88860777485636,-3.14304463431983));
#90080=CARTESIAN_POINT('',(0.3,-3.66169243810872,-3.07252477430166));
#90081=CARTESIAN_POINT('',(0.3,-4.09656172352352,-3.20767174838106));
#90082=CARTESIAN_POINT('',(5.4,-3.66169243810872,-3.07252477430166));
#90083=CARTESIAN_POINT('',(0.3,-3.66169243810872,-3.07252477430166));
#90084=CARTESIAN_POINT('',(5.4,-4.09656172352352,-3.20767174838106));
#90085=CARTESIAN_POINT('Origin',(5.4,-3.8225617711637,-3.20751017233583));
#90086=CARTESIAN_POINT('',(5.4,-3.77054437770685,-3.28374711202663));
#90087=CARTESIAN_POINT('Origin',(5.4,0.,0.));
#90088=CARTESIAN_POINT('',(5.4,-3.66169243810872,-3.07252477430166));
#90089=CARTESIAN_POINT('Origin',(0.3,-3.87030048491386,-3.47731939235894));
#90090=CARTESIAN_POINT('',(0.3,-3.77054437770685,-3.28374711202663));
#90091=CARTESIAN_POINT('',(2.7,-3.77054437770685,-3.28374711202663));
#90092=CARTESIAN_POINT('',(0.3,-3.66169243810872,-3.07252477430166));
#90093=CARTESIAN_POINT('Origin',(0.3,-3.8225617711637,-3.20751017233583));
#90094=CARTESIAN_POINT('Origin',(0.3,0.,0.));
#90095=CARTESIAN_POINT('Origin',(0.3,-4.13960143008962,-2.39));
#90096=CARTESIAN_POINT('',(0.3,-4.37531505817756,-2.42004507017632));
#90097=CARTESIAN_POINT('',(5.4,-4.37531505817756,-2.42004507017632));
#90098=CARTESIAN_POINT('',(2.7,-4.37531505817756,-2.42004507017632));
#90099=CARTESIAN_POINT('',(0.3,-4.13960143008962,-2.39));
#90100=CARTESIAN_POINT('',(0.3,-4.59133209967908,-2.44757952893394));
#90101=CARTESIAN_POINT('',(5.4,-4.13960143008962,-2.39));
#90102=CARTESIAN_POINT('',(0.3,-4.13960143008962,-2.39));
#90103=CARTESIAN_POINT('',(5.4,-4.59133209967908,-2.44757952893394));
#90104=CARTESIAN_POINT('Origin',(5.4,-4.32146676488435,-2.495));
#90105=CARTESIAN_POINT('',(5.4,-4.28347803816477,-2.57911145485419));
#90106=CARTESIAN_POINT('Origin',(5.4,0.,0.));
#90107=CARTESIAN_POINT('',(5.4,-4.13960143008962,-2.39));
#90108=CARTESIAN_POINT('Origin',(0.3,-4.41533209967908,-2.75242047106606));
#90109=CARTESIAN_POINT('',(0.3,-4.28347803816477,-2.57911145485419));
#90110=CARTESIAN_POINT('',(2.7,-4.28347803816477,-2.57911145485419));
#90111=CARTESIAN_POINT('',(0.3,-4.13960143008962,-2.39));
#90112=CARTESIAN_POINT('Origin',(0.3,-4.32146676488435,-2.495));
#90113=CARTESIAN_POINT('Origin',(0.3,0.,0.));
#90114=CARTESIAN_POINT('Origin',(0.3,-4.49173072735664,-1.6348562850967));
#90115=CARTESIAN_POINT('',(0.3,-4.72908060747227,-1.6235136611774));
#90116=CARTESIAN_POINT('',(5.4,-4.72908060747227,-1.6235136611774));
#90117=CARTESIAN_POINT('',(2.7,-4.72908060747227,-1.6235136611774));
#90118=CARTESIAN_POINT('',(0.3,-4.49173072735664,-1.6348562850967));
#90119=CARTESIAN_POINT('',(0.3,-4.94659717331204,-1.61311884403516));
#90120=CARTESIAN_POINT('',(5.4,-4.49173072735664,-1.6348562850967));
#90121=CARTESIAN_POINT('',(0.3,-4.49173072735664,-1.6348562850967));
#90122=CARTESIAN_POINT('',(5.4,-4.94659717331204,-1.61311884403516));
#90123=CARTESIAN_POINT('Origin',(5.4,-4.68906617772168,-1.70668051519509));
#90124=CARTESIAN_POINT('',(5.4,-4.66626038597752,-1.79611080121937));
#90125=CARTESIAN_POINT('Origin',(5.4,0.,0.));
#90126=CARTESIAN_POINT('',(5.4,-4.49173072735664,-1.6348562850967));
#90127=CARTESIAN_POINT('Origin',(0.3,-4.82620608286141,-1.9438906465518));
#90128=CARTESIAN_POINT('',(0.3,-4.66626038597752,-1.79611080121937));
#90129=CARTESIAN_POINT('',(2.7,-4.66626038597752,-1.79611080121937));
#90130=CARTESIAN_POINT('',(0.3,-4.49173072735664,-1.6348562850967));
#90131=CARTESIAN_POINT('Origin',(0.3,-4.68906617772168,-1.70668051519509));
#90132=CARTESIAN_POINT('Origin',(0.3,0.,0.));
#90133=CARTESIAN_POINT('Origin',(0.3,-4.70738105939836,-0.830038289247926));
#90134=CARTESIAN_POINT('',(0.3,-4.9391554355392,-0.777652611121161));
#90135=CARTESIAN_POINT('',(5.4,-4.9391554355392,-0.777652611121161));
#90136=CARTESIAN_POINT('',(2.7,-4.9391554355392,-0.777652611121161));
#90137=CARTESIAN_POINT('',(0.3,-4.70738105939836,-0.830038289247926));
#90138=CARTESIAN_POINT('',(0.3,-5.15156239493286,-0.729644359337888));
#90139=CARTESIAN_POINT('',(5.4,-4.70738105939836,-0.830038289247926));
#90140=CARTESIAN_POINT('',(0.3,-4.70738105939836,-0.830038289247926));
#90141=CARTESIAN_POINT('',(5.4,-5.15156239493286,-0.729644359337888));
#90142=CARTESIAN_POINT('Origin',(5.4,-4.91419068753092,-0.866504406557981));
#90143=CARTESIAN_POINT('',(5.4,-4.90726077320404,-0.958536229765421));
#90144=CARTESIAN_POINT('Origin',(5.4,0.,0.));
#90145=CARTESIAN_POINT('',(5.4,-4.70738105939836,-0.830038289247926));
#90146=CARTESIAN_POINT('Origin',(0.3,-5.0904382363941,-1.07629668839818));
#90147=CARTESIAN_POINT('',(0.3,-4.90726077320404,-0.958536229765421));
#90148=CARTESIAN_POINT('',(2.7,-4.90726077320404,-0.958536229765421));
#90149=CARTESIAN_POINT('',(0.3,-4.70738105939836,-0.830038289247926));
#90150=CARTESIAN_POINT('Origin',(0.3,-4.91419068753092,-0.866504406557981));
#90151=CARTESIAN_POINT('Origin',(0.3,0.,0.));
#90152=CARTESIAN_POINT('Origin',(0.3,-4.78,5.85381169992435E-16));
#90153=CARTESIAN_POINT('',(0.3,-4.99915652503051,0.0918370200127872));
#90154=CARTESIAN_POINT('',(5.4,-4.99915652503051,0.0918370200127872));
#90155=CARTESIAN_POINT('',(2.7,-4.99915652503051,0.0918370200127877));
#90156=CARTESIAN_POINT('',(0.3,-4.78,5.85381169992435E-16));
#90157=CARTESIAN_POINT('',(0.3,-5.2,0.176000000000001));
#90158=CARTESIAN_POINT('',(5.4,-4.78,5.85381169992435E-16));
#90159=CARTESIAN_POINT('',(0.3,-4.78,5.85381169992435E-16));
#90160=CARTESIAN_POINT('',(5.4,-5.2,0.176000000000001));
#90161=CARTESIAN_POINT('Origin',(5.4,-4.99,6.11098752774529E-16));
#90162=CARTESIAN_POINT('',(5.4,-5.,-6.12323399573677E-16));
#90163=CARTESIAN_POINT('Origin',(5.4,0.,0.));
#90164=CARTESIAN_POINT('',(5.4,-4.99915652503051,-0.0918370200127866));
#90165=CARTESIAN_POINT('',(5.4,-4.78,5.85381169992435E-16));
#90166=CARTESIAN_POINT('Origin',(5.4,0.,0.));
#90167=CARTESIAN_POINT('Origin',(0.3,-5.2,-0.175999999999999));
#90168=CARTESIAN_POINT('',(0.3,-4.99915652503051,-0.0918370200127866));
#90169=CARTESIAN_POINT('',(2.7,-4.99915652503051,-0.091837020012786));
#90170=CARTESIAN_POINT('',(0.3,-4.78,5.85381169992435E-16));
#90171=CARTESIAN_POINT('Origin',(0.3,-4.99,6.11098752774529E-16));
#90172=CARTESIAN_POINT('',(0.3,-5.,-6.12323399573677E-16));
#90173=CARTESIAN_POINT('Origin',(0.3,0.,0.));
#90174=CARTESIAN_POINT('Origin',(0.3,0.,0.));
#90175=CARTESIAN_POINT('Origin',(0.3,-4.70738105939835,0.830038289247929));
#90176=CARTESIAN_POINT('',(0.3,-4.90726077320404,0.958536229765424));
#90177=CARTESIAN_POINT('',(5.4,-4.90726077320404,0.958536229765424));
#90178=CARTESIAN_POINT('',(2.7,-4.90726077320404,0.958536229765425));
#90179=CARTESIAN_POINT('',(0.3,-4.70738105939835,0.830038289247929));
#90180=CARTESIAN_POINT('',(0.3,-5.0904382363941,1.07629668839819));
#90181=CARTESIAN_POINT('',(5.4,-4.70738105939835,0.830038289247929));
#90182=CARTESIAN_POINT('',(0.3,-4.70738105939835,0.830038289247929));
#90183=CARTESIAN_POINT('',(5.4,-5.0904382363941,1.07629668839819));
#90184=CARTESIAN_POINT('Origin',(5.4,-4.91419068753092,0.866504406557984));
#90185=CARTESIAN_POINT('',(5.4,-4.9391554355392,0.777652611121165));
#90186=CARTESIAN_POINT('Origin',(5.4,0.,0.));
#90187=CARTESIAN_POINT('',(5.4,-4.70738105939835,0.830038289247929));
#90188=CARTESIAN_POINT('Origin',(0.3,-5.15156239493286,0.729644359337891));
#90189=CARTESIAN_POINT('',(0.3,-4.9391554355392,0.777652611121165));
#90190=CARTESIAN_POINT('',(2.7,-4.9391554355392,0.777652611121165));
#90191=CARTESIAN_POINT('',(0.3,-4.70738105939835,0.830038289247929));
#90192=CARTESIAN_POINT('Origin',(0.3,-4.91419068753092,0.866504406557984));
#90193=CARTESIAN_POINT('Origin',(0.3,0.,0.));
#90194=CARTESIAN_POINT('Origin',(0.3,-4.49173072735664,1.6348562850967));
#90195=CARTESIAN_POINT('',(0.3,-4.66626038597752,1.79611080121937));
#90196=CARTESIAN_POINT('',(5.4,-4.66626038597752,1.79611080121937));
#90197=CARTESIAN_POINT('',(2.7,-4.66626038597752,1.79611080121937));
#90198=CARTESIAN_POINT('',(0.3,-4.49173072735664,1.6348562850967));
#90199=CARTESIAN_POINT('',(0.3,-4.82620608286141,1.9438906465518));
#90200=CARTESIAN_POINT('',(5.4,-4.49173072735664,1.6348562850967));
#90201=CARTESIAN_POINT('',(0.3,-4.49173072735664,1.6348562850967));
#90202=CARTESIAN_POINT('',(5.4,-4.82620608286141,1.9438906465518));
#90203=CARTESIAN_POINT('Origin',(5.4,-4.68906617772168,1.70668051519509));
#90204=CARTESIAN_POINT('',(5.4,-4.72908060747227,1.62351366117741));
#90205=CARTESIAN_POINT('Origin',(5.4,0.,0.));
#90206=CARTESIAN_POINT('',(5.4,-4.49173072735664,1.6348562850967));
#90207=CARTESIAN_POINT('Origin',(0.3,-4.94659717331204,1.61311884403516));
#90208=CARTESIAN_POINT('',(0.3,-4.72908060747227,1.62351366117741));
#90209=CARTESIAN_POINT('',(2.7,-4.72908060747227,1.62351366117741));
#90210=CARTESIAN_POINT('',(0.3,-4.49173072735664,1.6348562850967));
#90211=CARTESIAN_POINT('Origin',(0.3,-4.68906617772168,1.70668051519509));
#90212=CARTESIAN_POINT('Origin',(0.3,0.,0.));
#90213=CARTESIAN_POINT('Origin',(0.3,-4.13960143008962,2.39));
#90214=CARTESIAN_POINT('',(0.3,-4.28347803816477,2.57911145485419));
#90215=CARTESIAN_POINT('',(5.4,-4.28347803816477,2.57911145485419));
#90216=CARTESIAN_POINT('',(2.7,-4.28347803816477,2.57911145485419));
#90217=CARTESIAN_POINT('',(0.3,-4.13960143008962,2.39));
#90218=CARTESIAN_POINT('',(0.3,-4.41533209967908,2.75242047106606));
#90219=CARTESIAN_POINT('',(5.4,-4.13960143008962,2.39));
#90220=CARTESIAN_POINT('',(0.3,-4.13960143008962,2.39));
#90221=CARTESIAN_POINT('',(5.4,-4.41533209967908,2.75242047106606));
#90222=CARTESIAN_POINT('Origin',(5.4,-4.32146676488435,2.495));
#90223=CARTESIAN_POINT('',(5.4,-4.37531505817756,2.42004507017632));
#90224=CARTESIAN_POINT('Origin',(5.4,0.,0.));
#90225=CARTESIAN_POINT('',(5.4,-4.13960143008962,2.39));
#90226=CARTESIAN_POINT('Origin',(0.3,-4.59133209967908,2.44757952893394));
#90227=CARTESIAN_POINT('',(0.3,-4.37531505817756,2.42004507017632));
#90228=CARTESIAN_POINT('',(2.7,-4.37531505817756,2.42004507017632));
#90229=CARTESIAN_POINT('',(0.3,-4.13960143008962,2.39));
#90230=CARTESIAN_POINT('Origin',(0.3,-4.32146676488435,2.495));
#90231=CARTESIAN_POINT('Origin',(0.3,0.,0.));
#90232=CARTESIAN_POINT('Origin',(0.3,-3.66169243810871,3.07252477430166));
#90233=CARTESIAN_POINT('',(0.3,-3.77054437770685,3.28374711202663));
#90234=CARTESIAN_POINT('',(5.4,-3.77054437770685,3.28374711202663));
#90235=CARTESIAN_POINT('',(2.7,-3.77054437770685,3.28374711202663));
#90236=CARTESIAN_POINT('',(0.3,-3.66169243810871,3.07252477430166));
#90237=CARTESIAN_POINT('',(0.3,-3.87030048491385,3.47731939235895));
#90238=CARTESIAN_POINT('',(5.4,-3.66169243810871,3.07252477430166));
#90239=CARTESIAN_POINT('',(0.3,-3.66169243810871,3.07252477430166));
#90240=CARTESIAN_POINT('',(5.4,-3.87030048491385,3.47731939235895));
#90241=CARTESIAN_POINT('Origin',(5.4,-3.8225617711637,3.20751017233583));
#90242=CARTESIAN_POINT('',(5.4,-3.88860777485636,3.14304463431983));
#90243=CARTESIAN_POINT('Origin',(5.4,0.,0.));
#90244=CARTESIAN_POINT('',(5.4,-3.66169243810871,3.07252477430166));
#90245=CARTESIAN_POINT('Origin',(0.3,-4.09656172352352,3.20767174838107));
#90246=CARTESIAN_POINT('',(0.3,-3.88860777485636,3.14304463431983));
#90247=CARTESIAN_POINT('',(2.7,-3.88860777485636,3.14304463431983));
#90248=CARTESIAN_POINT('',(0.3,-3.66169243810871,3.07252477430166));
#90249=CARTESIAN_POINT('Origin',(0.3,-3.8225617711637,3.20751017233583));
#90250=CARTESIAN_POINT('Origin',(0.3,0.,0.));
#90251=CARTESIAN_POINT('Origin',(0.3,-3.07252477430166,3.66169243810872));
#90252=CARTESIAN_POINT('',(0.3,-3.14304463431983,3.88860777485636));
#90253=CARTESIAN_POINT('',(5.4,-3.14304463431983,3.88860777485636));
#90254=CARTESIAN_POINT('',(2.7,-3.14304463431983,3.88860777485636));
#90255=CARTESIAN_POINT('',(0.3,-3.07252477430166,3.66169243810872));
#90256=CARTESIAN_POINT('',(0.3,-3.20767174838106,4.09656172352352));
#90257=CARTESIAN_POINT('',(5.4,-3.07252477430166,3.66169243810872));
#90258=CARTESIAN_POINT('',(0.3,-3.07252477430166,3.66169243810872));
#90259=CARTESIAN_POINT('',(5.4,-3.20767174838106,4.09656172352352));
#90260=CARTESIAN_POINT('Origin',(5.4,-3.20751017233583,3.8225617711637));
#90261=CARTESIAN_POINT('',(5.4,-3.28374711202663,3.77054437770685));
#90262=CARTESIAN_POINT('Origin',(5.4,0.,0.));
#90263=CARTESIAN_POINT('',(5.4,-3.07252477430166,3.66169243810872));
#90264=CARTESIAN_POINT('Origin',(0.3,-3.47731939235894,3.87030048491386));
#90265=CARTESIAN_POINT('',(0.3,-3.28374711202663,3.77054437770685));
#90266=CARTESIAN_POINT('',(2.7,-3.28374711202663,3.77054437770685));
#90267=CARTESIAN_POINT('',(0.3,-3.07252477430166,3.66169243810872));
#90268=CARTESIAN_POINT('Origin',(0.3,-3.20751017233583,3.8225617711637));
#90269=CARTESIAN_POINT('Origin',(0.3,0.,0.));
#90270=CARTESIAN_POINT('Origin',(0.3,-2.39,4.13960143008962));
#90271=CARTESIAN_POINT('',(0.3,-2.42004507017632,4.37531505817756));
#90272=CARTESIAN_POINT('',(5.4,-2.42004507017632,4.37531505817756));
#90273=CARTESIAN_POINT('',(2.7,-2.42004507017632,4.37531505817756));
#90274=CARTESIAN_POINT('',(0.3,-2.39,4.13960143008962));
#90275=CARTESIAN_POINT('',(0.3,-2.44757952893394,4.59133209967908));
#90276=CARTESIAN_POINT('',(5.4,-2.39,4.13960143008962));
#90277=CARTESIAN_POINT('',(0.3,-2.39,4.13960143008962));
#90278=CARTESIAN_POINT('',(5.4,-2.44757952893394,4.59133209967908));
#90279=CARTESIAN_POINT('Origin',(5.4,-2.495,4.32146676488435));
#90280=CARTESIAN_POINT('',(5.4,-2.57911145485419,4.28347803816477));
#90281=CARTESIAN_POINT('Origin',(5.4,0.,0.));
#90282=CARTESIAN_POINT('',(5.4,-2.39,4.13960143008962));
#90283=CARTESIAN_POINT('Origin',(0.3,-2.75242047106606,4.41533209967908));
#90284=CARTESIAN_POINT('',(0.3,-2.57911145485419,4.28347803816477));
#90285=CARTESIAN_POINT('',(2.7,-2.57911145485419,4.28347803816477));
#90286=CARTESIAN_POINT('',(0.3,-2.39,4.13960143008962));
#90287=CARTESIAN_POINT('Origin',(0.3,-2.495,4.32146676488435));
#90288=CARTESIAN_POINT('Origin',(0.3,0.,0.));
#90289=CARTESIAN_POINT('Origin',(0.3,-1.6348562850967,4.49173072735664));
#90290=CARTESIAN_POINT('',(0.3,-1.6235136611774,4.72908060747227));
#90291=CARTESIAN_POINT('',(5.4,-1.6235136611774,4.72908060747227));
#90292=CARTESIAN_POINT('',(2.7,-1.6235136611774,4.72908060747227));
#90293=CARTESIAN_POINT('',(0.3,-1.6348562850967,4.49173072735664));
#90294=CARTESIAN_POINT('',(0.3,-1.61311884403516,4.94659717331204));
#90295=CARTESIAN_POINT('',(5.4,-1.6348562850967,4.49173072735664));
#90296=CARTESIAN_POINT('',(0.3,-1.6348562850967,4.49173072735664));
#90297=CARTESIAN_POINT('',(5.4,-1.61311884403516,4.94659717331204));
#90298=CARTESIAN_POINT('Origin',(5.4,-1.70668051519509,4.68906617772168));
#90299=CARTESIAN_POINT('',(5.4,-1.79611080121937,4.66626038597752));
#90300=CARTESIAN_POINT('Origin',(5.4,0.,0.));
#90301=CARTESIAN_POINT('',(5.4,-1.6348562850967,4.49173072735664));
#90302=CARTESIAN_POINT('Origin',(0.3,-1.9438906465518,4.82620608286141));
#90303=CARTESIAN_POINT('',(0.3,-1.79611080121937,4.66626038597752));
#90304=CARTESIAN_POINT('',(2.7,-1.79611080121937,4.66626038597752));
#90305=CARTESIAN_POINT('',(0.3,-1.6348562850967,4.49173072735664));
#90306=CARTESIAN_POINT('Origin',(0.3,-1.70668051519509,4.68906617772168));
#90307=CARTESIAN_POINT('Origin',(0.3,0.,0.));
#90308=CARTESIAN_POINT('Origin',(0.3,-0.830038289247927,4.70738105939836));
#90309=CARTESIAN_POINT('',(0.3,-0.777652611121163,4.9391554355392));
#90310=CARTESIAN_POINT('',(5.4,-0.777652611121163,4.9391554355392));
#90311=CARTESIAN_POINT('',(2.7,-0.777652611121163,4.9391554355392));
#90312=CARTESIAN_POINT('',(0.3,-0.830038289247927,4.70738105939836));
#90313=CARTESIAN_POINT('',(0.3,-0.729644359337889,5.15156239493286));
#90314=CARTESIAN_POINT('',(5.4,-0.830038289247927,4.70738105939836));
#90315=CARTESIAN_POINT('',(0.3,-0.830038289247927,4.70738105939836));
#90316=CARTESIAN_POINT('',(5.4,-0.729644359337889,5.15156239493286));
#90317=CARTESIAN_POINT('Origin',(5.4,-0.866504406557982,4.91419068753092));
#90318=CARTESIAN_POINT('',(5.4,-0.958536229765423,4.90726077320404));
#90319=CARTESIAN_POINT('Origin',(5.4,0.,0.));
#90320=CARTESIAN_POINT('',(5.4,-0.830038289247927,4.70738105939836));
#90321=CARTESIAN_POINT('Origin',(0.3,-1.07629668839819,5.0904382363941));
#90322=CARTESIAN_POINT('',(0.3,-0.958536229765423,4.90726077320404));
#90323=CARTESIAN_POINT('',(2.7,-0.958536229765423,4.90726077320404));
#90324=CARTESIAN_POINT('',(0.3,-0.830038289247927,4.70738105939836));
#90325=CARTESIAN_POINT('Origin',(0.3,-0.866504406557982,4.91419068753092));
#90326=CARTESIAN_POINT('Origin',(0.3,0.,0.));
#90327=CARTESIAN_POINT('Origin',(0.3,2.92690584996217E-16,4.78));
#90328=CARTESIAN_POINT('',(0.3,0.0918370200127869,4.99915652503051));
#90329=CARTESIAN_POINT('',(5.4,0.0918370200127869,4.99915652503051));
#90330=CARTESIAN_POINT('',(2.7,0.0918370200127874,4.99915652503051));
#90331=CARTESIAN_POINT('',(0.3,2.92690584996217E-16,4.78));
#90332=CARTESIAN_POINT('',(0.3,0.176,5.2));
#90333=CARTESIAN_POINT('',(5.4,2.92690584996217E-16,4.78));
#90334=CARTESIAN_POINT('',(0.3,2.92690584996217E-16,4.78));
#90335=CARTESIAN_POINT('',(5.4,0.176,5.2));
#90336=CARTESIAN_POINT('Origin',(5.4,3.05549376387265E-16,4.99));
#90337=CARTESIAN_POINT('',(5.4,-0.0918370200127869,4.99915652503051));
#90338=CARTESIAN_POINT('Origin',(5.4,0.,0.));
#90339=CARTESIAN_POINT('',(5.4,2.92690584996217E-16,4.78));
#90340=CARTESIAN_POINT('Origin',(0.3,-0.176,5.2));
#90341=CARTESIAN_POINT('',(0.3,-0.0918370200127869,4.99915652503051));
#90342=CARTESIAN_POINT('',(2.7,-0.0918370200127863,4.99915652503051));
#90343=CARTESIAN_POINT('',(0.3,2.92690584996217E-16,4.78));
#90344=CARTESIAN_POINT('Origin',(0.3,3.05549376387265E-16,4.99));
#90345=CARTESIAN_POINT('Origin',(0.3,0.,0.));
#90346=CARTESIAN_POINT('Origin',(0.3,0.830038289247928,4.70738105939836));
#90347=CARTESIAN_POINT('',(0.3,0.958536229765423,4.90726077320404));
#90348=CARTESIAN_POINT('',(5.4,0.958536229765423,4.90726077320404));
#90349=CARTESIAN_POINT('',(2.7,0.958536229765423,4.90726077320404));
#90350=CARTESIAN_POINT('',(0.3,0.830038289247928,4.70738105939836));
#90351=CARTESIAN_POINT('',(0.3,1.07629668839819,5.0904382363941));
#90352=CARTESIAN_POINT('',(5.4,0.830038289247928,4.70738105939836));
#90353=CARTESIAN_POINT('',(0.3,0.830038289247928,4.70738105939836));
#90354=CARTESIAN_POINT('',(5.4,1.07629668839819,5.0904382363941));
#90355=CARTESIAN_POINT('Origin',(5.4,0.866504406557983,4.91419068753092));
#90356=CARTESIAN_POINT('',(5.4,0.777652611121164,4.9391554355392));
#90357=CARTESIAN_POINT('Origin',(5.4,0.,0.));
#90358=CARTESIAN_POINT('',(5.4,0.830038289247928,4.70738105939836));
#90359=CARTESIAN_POINT('Origin',(0.3,0.72964435933789,5.15156239493286));
#90360=CARTESIAN_POINT('',(0.3,0.777652611121164,4.9391554355392));
#90361=CARTESIAN_POINT('',(2.7,0.777652611121163,4.9391554355392));
#90362=CARTESIAN_POINT('',(0.3,0.830038289247928,4.70738105939836));
#90363=CARTESIAN_POINT('Origin',(0.3,0.866504406557983,4.91419068753092));
#90364=CARTESIAN_POINT('Origin',(0.3,0.,0.));
#90365=CARTESIAN_POINT('Origin',(0.3,1.6348562850967,4.49173072735664));
#90366=CARTESIAN_POINT('',(0.3,1.79611080121937,4.66626038597752));
#90367=CARTESIAN_POINT('',(5.4,1.79611080121937,4.66626038597752));
#90368=CARTESIAN_POINT('',(2.7,1.79611080121937,4.66626038597752));
#90369=CARTESIAN_POINT('',(0.3,1.6348562850967,4.49173072735664));
#90370=CARTESIAN_POINT('',(0.3,1.9438906465518,4.82620608286141));
#90371=CARTESIAN_POINT('',(5.4,1.6348562850967,4.49173072735664));
#90372=CARTESIAN_POINT('',(0.3,1.6348562850967,4.49173072735664));
#90373=CARTESIAN_POINT('',(5.4,1.9438906465518,4.82620608286141));
#90374=CARTESIAN_POINT('Origin',(5.4,1.70668051519509,4.68906617772168));
#90375=CARTESIAN_POINT('',(5.4,1.62351366117741,4.72908060747227));
#90376=CARTESIAN_POINT('Origin',(5.4,0.,0.));
#90377=CARTESIAN_POINT('',(5.4,1.6348562850967,4.49173072735664));
#90378=CARTESIAN_POINT('Origin',(0.3,1.61311884403516,4.94659717331204));
#90379=CARTESIAN_POINT('',(0.3,1.62351366117741,4.72908060747227));
#90380=CARTESIAN_POINT('',(2.7,1.62351366117741,4.72908060747227));
#90381=CARTESIAN_POINT('',(0.3,1.6348562850967,4.49173072735664));
#90382=CARTESIAN_POINT('Origin',(0.3,1.70668051519509,4.68906617772168));
#90383=CARTESIAN_POINT('Origin',(0.3,0.,0.));
#90384=CARTESIAN_POINT('Origin',(0.3,2.39,4.13960143008962));
#90385=CARTESIAN_POINT('',(0.3,2.57911145485419,4.28347803816477));
#90386=CARTESIAN_POINT('',(5.4,2.57911145485419,4.28347803816477));
#90387=CARTESIAN_POINT('',(2.7,2.57911145485419,4.28347803816477));
#90388=CARTESIAN_POINT('',(0.3,2.39,4.13960143008962));
#90389=CARTESIAN_POINT('',(0.3,2.75242047106606,4.41533209967908));
#90390=CARTESIAN_POINT('',(5.4,2.39,4.13960143008962));
#90391=CARTESIAN_POINT('',(0.3,2.39,4.13960143008962));
#90392=CARTESIAN_POINT('',(5.4,2.75242047106606,4.41533209967908));
#90393=CARTESIAN_POINT('Origin',(5.4,2.495,4.32146676488435));
#90394=CARTESIAN_POINT('',(5.4,2.42004507017632,4.37531505817756));
#90395=CARTESIAN_POINT('Origin',(5.4,0.,0.));
#90396=CARTESIAN_POINT('',(5.4,2.39,4.13960143008962));
#90397=CARTESIAN_POINT('Origin',(0.3,2.44757952893394,4.59133209967908));
#90398=CARTESIAN_POINT('',(0.3,2.42004507017632,4.37531505817756));
#90399=CARTESIAN_POINT('',(2.7,2.42004507017632,4.37531505817756));
#90400=CARTESIAN_POINT('',(0.3,2.39,4.13960143008962));
#90401=CARTESIAN_POINT('Origin',(0.3,2.495,4.32146676488435));
#90402=CARTESIAN_POINT('Origin',(0.3,0.,0.));
#90403=CARTESIAN_POINT('Origin',(0.3,3.07252477430166,3.66169243810872));
#90404=CARTESIAN_POINT('',(0.3,3.28374711202663,3.77054437770685));
#90405=CARTESIAN_POINT('',(5.4,3.28374711202663,3.77054437770685));
#90406=CARTESIAN_POINT('',(2.7,3.28374711202663,3.77054437770685));
#90407=CARTESIAN_POINT('',(0.3,3.07252477430166,3.66169243810872));
#90408=CARTESIAN_POINT('',(0.3,3.47731939235894,3.87030048491386));
#90409=CARTESIAN_POINT('',(5.4,3.07252477430166,3.66169243810872));
#90410=CARTESIAN_POINT('',(0.3,3.07252477430166,3.66169243810872));
#90411=CARTESIAN_POINT('',(5.4,3.47731939235894,3.87030048491386));
#90412=CARTESIAN_POINT('Origin',(5.4,3.20751017233583,3.8225617711637));
#90413=CARTESIAN_POINT('',(5.4,3.14304463431983,3.88860777485636));
#90414=CARTESIAN_POINT('Origin',(5.4,0.,0.));
#90415=CARTESIAN_POINT('',(5.4,3.07252477430166,3.66169243810872));
#90416=CARTESIAN_POINT('Origin',(0.3,3.20767174838106,4.09656172352352));
#90417=CARTESIAN_POINT('',(0.3,3.14304463431983,3.88860777485636));
#90418=CARTESIAN_POINT('',(2.7,3.14304463431983,3.88860777485636));
#90419=CARTESIAN_POINT('',(0.3,3.07252477430166,3.66169243810872));
#90420=CARTESIAN_POINT('Origin',(0.3,3.20751017233583,3.8225617711637));
#90421=CARTESIAN_POINT('Origin',(0.3,0.,0.));
#90422=CARTESIAN_POINT('Origin',(0.3,3.66169243810872,3.07252477430166));
#90423=CARTESIAN_POINT('',(0.3,3.88860777485636,3.14304463431983));
#90424=CARTESIAN_POINT('',(5.4,3.88860777485636,3.14304463431983));
#90425=CARTESIAN_POINT('',(2.7,3.88860777485636,3.14304463431983));
#90426=CARTESIAN_POINT('',(0.3,3.66169243810872,3.07252477430166));
#90427=CARTESIAN_POINT('',(0.3,4.09656172352352,3.20767174838106));
#90428=CARTESIAN_POINT('',(5.4,3.66169243810872,3.07252477430166));
#90429=CARTESIAN_POINT('',(0.3,3.66169243810872,3.07252477430166));
#90430=CARTESIAN_POINT('',(5.4,4.09656172352352,3.20767174838106));
#90431=CARTESIAN_POINT('Origin',(5.4,3.8225617711637,3.20751017233583));
#90432=CARTESIAN_POINT('',(5.4,3.77054437770685,3.28374711202663));
#90433=CARTESIAN_POINT('Origin',(5.4,0.,0.));
#90434=CARTESIAN_POINT('',(5.4,3.66169243810872,3.07252477430166));
#90435=CARTESIAN_POINT('Origin',(0.3,3.87030048491386,3.47731939235894));
#90436=CARTESIAN_POINT('',(0.3,3.77054437770685,3.28374711202663));
#90437=CARTESIAN_POINT('',(2.7,3.77054437770685,3.28374711202663));
#90438=CARTESIAN_POINT('',(0.3,3.66169243810872,3.07252477430166));
#90439=CARTESIAN_POINT('Origin',(0.3,3.8225617711637,3.20751017233583));
#90440=CARTESIAN_POINT('Origin',(0.3,0.,0.));
#90441=CARTESIAN_POINT('Origin',(0.3,4.13960143008962,2.39));
#90442=CARTESIAN_POINT('',(0.3,4.37531505817756,2.42004507017632));
#90443=CARTESIAN_POINT('',(5.4,4.37531505817756,2.42004507017632));
#90444=CARTESIAN_POINT('',(2.7,4.37531505817756,2.42004507017632));
#90445=CARTESIAN_POINT('',(0.3,4.13960143008962,2.39));
#90446=CARTESIAN_POINT('',(0.3,4.59133209967908,2.44757952893394));
#90447=CARTESIAN_POINT('',(5.4,4.13960143008962,2.39));
#90448=CARTESIAN_POINT('',(0.3,4.13960143008962,2.39));
#90449=CARTESIAN_POINT('',(5.4,4.59133209967908,2.44757952893394));
#90450=CARTESIAN_POINT('Origin',(5.4,4.32146676488435,2.495));
#90451=CARTESIAN_POINT('',(5.4,4.28347803816477,2.57911145485419));
#90452=CARTESIAN_POINT('Origin',(5.4,0.,0.));
#90453=CARTESIAN_POINT('',(5.4,4.13960143008962,2.39));
#90454=CARTESIAN_POINT('Origin',(0.3,4.41533209967908,2.75242047106606));
#90455=CARTESIAN_POINT('',(0.3,4.28347803816477,2.57911145485419));
#90456=CARTESIAN_POINT('',(2.7,4.28347803816477,2.57911145485419));
#90457=CARTESIAN_POINT('',(0.3,4.13960143008962,2.39));
#90458=CARTESIAN_POINT('Origin',(0.3,4.32146676488435,2.495));
#90459=CARTESIAN_POINT('Origin',(0.3,0.,0.));
#90460=CARTESIAN_POINT('Origin',(0.3,4.49173072735664,1.6348562850967));
#90461=CARTESIAN_POINT('',(0.3,4.72908060747227,1.6235136611774));
#90462=CARTESIAN_POINT('',(5.4,4.72908060747227,1.6235136611774));
#90463=CARTESIAN_POINT('',(2.7,4.72908060747227,1.6235136611774));
#90464=CARTESIAN_POINT('',(0.3,4.49173072735664,1.6348562850967));
#90465=CARTESIAN_POINT('',(0.3,4.94659717331204,1.61311884403516));
#90466=CARTESIAN_POINT('',(5.4,4.49173072735664,1.6348562850967));
#90467=CARTESIAN_POINT('',(0.3,4.49173072735664,1.6348562850967));
#90468=CARTESIAN_POINT('',(5.4,4.94659717331204,1.61311884403516));
#90469=CARTESIAN_POINT('Origin',(5.4,4.68906617772168,1.70668051519509));
#90470=CARTESIAN_POINT('',(5.4,4.66626038597752,1.79611080121937));
#90471=CARTESIAN_POINT('Origin',(5.4,0.,0.));
#90472=CARTESIAN_POINT('',(5.4,4.49173072735664,1.6348562850967));
#90473=CARTESIAN_POINT('Origin',(0.3,4.82620608286141,1.9438906465518));
#90474=CARTESIAN_POINT('',(0.3,4.66626038597752,1.79611080121937));
#90475=CARTESIAN_POINT('',(2.7,4.66626038597752,1.79611080121937));
#90476=CARTESIAN_POINT('',(0.3,4.49173072735664,1.6348562850967));
#90477=CARTESIAN_POINT('Origin',(0.3,4.68906617772168,1.70668051519509));
#90478=CARTESIAN_POINT('Origin',(0.3,0.,0.));
#90479=CARTESIAN_POINT('Origin',(0.3,4.70738105939836,0.830038289247927));
#90480=CARTESIAN_POINT('',(0.3,4.9391554355392,0.777652611121163));
#90481=CARTESIAN_POINT('',(5.4,4.9391554355392,0.777652611121163));
#90482=CARTESIAN_POINT('',(2.7,4.9391554355392,0.777652611121163));
#90483=CARTESIAN_POINT('',(0.3,4.70738105939836,0.830038289247927));
#90484=CARTESIAN_POINT('',(0.3,5.15156239493286,0.729644359337889));
#90485=CARTESIAN_POINT('',(5.4,4.70738105939836,0.830038289247927));
#90486=CARTESIAN_POINT('',(0.3,4.70738105939836,0.830038289247927));
#90487=CARTESIAN_POINT('',(5.4,5.15156239493286,0.729644359337889));
#90488=CARTESIAN_POINT('Origin',(5.4,4.91419068753092,0.866504406557982));
#90489=CARTESIAN_POINT('',(5.4,4.90726077320404,0.958536229765423));
#90490=CARTESIAN_POINT('Origin',(5.4,0.,0.));
#90491=CARTESIAN_POINT('',(5.4,4.70738105939836,0.830038289247927));
#90492=CARTESIAN_POINT('Origin',(0.3,5.0904382363941,1.07629668839819));
#90493=CARTESIAN_POINT('',(0.3,4.90726077320404,0.958536229765423));
#90494=CARTESIAN_POINT('',(2.7,4.90726077320404,0.958536229765423));
#90495=CARTESIAN_POINT('',(0.3,4.70738105939836,0.830038289247927));
#90496=CARTESIAN_POINT('Origin',(0.3,4.91419068753092,0.866504406557982));
#90497=CARTESIAN_POINT('Origin',(0.3,0.,0.));
#90498=CARTESIAN_POINT('Origin',(5.4,4.99,0.));
#90499=CARTESIAN_POINT('',(5.4,4.99915652503051,-0.0918370200127866));
#90500=CARTESIAN_POINT('',(5.4,4.99915652503051,0.0918370200127872));
#90501=CARTESIAN_POINT('Origin',(5.4,0.,0.));
#90502=CARTESIAN_POINT('',(5.4,4.78,0.));
#90503=CARTESIAN_POINT('',(5.4,5.2,-0.176));
#90504=CARTESIAN_POINT('',(5.4,4.78,0.));
#90505=CARTESIAN_POINT('Origin',(0.3,4.78,0.));
#90506=CARTESIAN_POINT('',(0.3,4.99915652503051,-0.0918370200127866));
#90507=CARTESIAN_POINT('',(2.7,4.99915652503051,-0.0918370200127872));
#90508=CARTESIAN_POINT('',(0.3,4.78,0.));
#90509=CARTESIAN_POINT('',(0.3,5.2,-0.176));
#90510=CARTESIAN_POINT('',(0.3,4.78,0.));
#90511=CARTESIAN_POINT('Origin',(0.3,5.2,0.176));
#90512=CARTESIAN_POINT('',(0.3,4.99915652503051,0.0918370200127872));
#90513=CARTESIAN_POINT('',(2.7,4.99915652503051,0.0918370200127866));
#90514=CARTESIAN_POINT('',(0.3,4.78,0.));
#90515=CARTESIAN_POINT('Origin',(0.3,4.99,0.));
#90516=CARTESIAN_POINT('Origin',(0.3,0.,0.));
#90517=CARTESIAN_POINT('Origin',(2.25392422621555,0.,0.));
#90518=CARTESIAN_POINT('',(1.4978484524311,0.,0.));
#90519=CARTESIAN_POINT('',(3.,-2.48346726553949,3.04137023753017E-16));
#90520=CARTESIAN_POINT('',(2.25392422621555,-1.25,-1.53080849893419E-16));
#90521=CARTESIAN_POINT('Origin',(3.,0.,0.));
#90522=CARTESIAN_POINT('Origin',(3.,1.76762539787484E-16,2.88675134594813));
#90523=CARTESIAN_POINT('',(6.,-2.5,1.44337567297406));
#90524=CARTESIAN_POINT('',(6.,1.76762539787484E-16,2.88675134594813));
#90525=CARTESIAN_POINT('',(6.,-0.625,2.52590742770461));
#90526=CARTESIAN_POINT('',(3.,-2.5,1.44337567297406));
#90527=CARTESIAN_POINT('',(3.,-2.5,1.44337567297406));
#90528=CARTESIAN_POINT('',(3.,1.76762539787484E-16,2.88675134594813));
#90529=CARTESIAN_POINT('',(3.,1.76762539787484E-16,2.88675134594813));
#90530=CARTESIAN_POINT('',(3.,1.76762539787484E-16,2.88675134594813));
#90531=CARTESIAN_POINT('Origin',(3.,2.5,1.44337567297406));
#90532=CARTESIAN_POINT('',(6.,2.5,1.44337567297406));
#90533=CARTESIAN_POINT('',(6.,1.875,1.80421959121758));
#90534=CARTESIAN_POINT('',(3.,2.5,1.44337567297406));
#90535=CARTESIAN_POINT('',(3.,2.5,1.44337567297406));
#90536=CARTESIAN_POINT('',(3.,2.5,1.44337567297406));
#90537=CARTESIAN_POINT('Origin',(3.,2.5,-1.44337567297407));
#90538=CARTESIAN_POINT('',(6.,2.5,-1.44337567297407));
#90539=CARTESIAN_POINT('',(6.,2.5,-0.721687836487033));
#90540=CARTESIAN_POINT('',(3.,2.5,-1.44337567297407));
#90541=CARTESIAN_POINT('',(3.,2.5,-1.44337567297407));
#90542=CARTESIAN_POINT('',(3.,2.5,-1.44337567297407));
#90543=CARTESIAN_POINT('Origin',(3.,-5.30287619362453E-16,-2.88675134594813));
#90544=CARTESIAN_POINT('',(6.,-5.30287619362453E-16,-2.88675134594813));
#90545=CARTESIAN_POINT('',(6.,0.625,-2.52590742770461));
#90546=CARTESIAN_POINT('',(3.,-5.30287619362453E-16,-2.88675134594813));
#90547=CARTESIAN_POINT('',(3.,-5.30287619362453E-16,-2.88675134594813));
#90548=CARTESIAN_POINT('',(3.,-5.30287619362453E-16,-2.88675134594813));
#90549=CARTESIAN_POINT('Origin',(3.,-2.5,-1.44337567297406));
#90550=CARTESIAN_POINT('',(6.,-2.5,-1.44337567297406));
#90551=CARTESIAN_POINT('',(6.,-1.875,-1.80421959121758));
#90552=CARTESIAN_POINT('',(3.,-2.5,-1.44337567297406));
#90553=CARTESIAN_POINT('',(3.,-2.5,-1.44337567297406));
#90554=CARTESIAN_POINT('',(3.,-2.5,-1.44337567297406));
#90555=CARTESIAN_POINT('Origin',(3.,-2.5,1.44337567297406));
#90556=CARTESIAN_POINT('',(6.,-2.5,0.721687836487032));
#90557=CARTESIAN_POINT('',(3.,-2.5,1.44337567297406));
#90558=CARTESIAN_POINT('Origin',(3.,0.,0.));
#90559=CARTESIAN_POINT('Origin',(-16.,2.4,0.));
#90560=CARTESIAN_POINT('',(-16.,-2.4,-2.93915231795365E-16));
#90561=CARTESIAN_POINT('Origin',(-16.,0.,0.));
#90562=CARTESIAN_POINT('Origin',(-15.7,0.,0.));
#90563=CARTESIAN_POINT('',(-15.7,-2.7,-3.30654635769785E-16));
#90564=CARTESIAN_POINT('Origin',(2.7,0.,0.));
#90565=CARTESIAN_POINT('Origin',(5.4,0.,0.));
#90566=CARTESIAN_POINT('Origin',(5.4,0.,0.));
#90567=CARTESIAN_POINT('Origin',(5.4,0.,0.));
#90568=CARTESIAN_POINT('Origin',(5.4,0.,0.));
#90569=CARTESIAN_POINT('Origin',(5.4,0.,0.));
#90570=CARTESIAN_POINT('Origin',(5.4,0.,0.));
#90571=CARTESIAN_POINT('Origin',(5.4,0.,0.));
#90572=CARTESIAN_POINT('Origin',(5.4,0.,0.));
#90573=CARTESIAN_POINT('Origin',(5.4,0.,0.));
#90574=CARTESIAN_POINT('Origin',(5.4,0.,0.));
#90575=CARTESIAN_POINT('Origin',(5.4,0.,0.));
#90576=CARTESIAN_POINT('Origin',(5.4,0.,0.));
#90577=CARTESIAN_POINT('Origin',(5.4,0.,0.));
#90578=CARTESIAN_POINT('Origin',(5.4,0.,0.));
#90579=CARTESIAN_POINT('Origin',(5.4,0.,0.));
#90580=CARTESIAN_POINT('Origin',(5.4,0.,0.));
#90581=CARTESIAN_POINT('Origin',(5.4,0.,0.));
#90582=CARTESIAN_POINT('',(2.7,-5.,-6.12323399573677E-16));
#90583=CARTESIAN_POINT('Origin',(5.4,0.,0.));
#90584=CARTESIAN_POINT('Origin',(5.4,0.,0.));
#90585=CARTESIAN_POINT('Origin',(5.4,0.,0.));
#90586=CARTESIAN_POINT('Origin',(5.4,0.,0.));
#90587=CARTESIAN_POINT('Origin',(5.4,0.,0.));
#90588=CARTESIAN_POINT('Origin',(5.4,0.,0.));
#90589=CARTESIAN_POINT('Origin',(5.4,0.,0.));
#90590=CARTESIAN_POINT('Origin',(5.4,0.,0.));
#90591=CARTESIAN_POINT('Origin',(5.4,0.,0.));
#90592=CARTESIAN_POINT('Origin',(5.4,0.,0.));
#90593=CARTESIAN_POINT('Origin',(5.4,0.,0.));
#90594=CARTESIAN_POINT('Origin',(5.4,0.,0.));
#90595=CARTESIAN_POINT('Origin',(5.4,0.,0.));
#90596=CARTESIAN_POINT('Origin',(5.4,0.,0.));
#90597=CARTESIAN_POINT('Origin',(5.4,0.,0.));
#90598=CARTESIAN_POINT('Origin',(5.4,0.,0.));
#90599=CARTESIAN_POINT('Origin',(5.4,0.,0.));
#90600=CARTESIAN_POINT('Origin',(5.4,0.,0.));
#90601=CARTESIAN_POINT('Origin',(5.4,0.,0.));
#90602=CARTESIAN_POINT('Origin',(5.7,0.,0.));
#90603=CARTESIAN_POINT('',(6.,-4.4,-5.38844591624836E-16));
#90604=CARTESIAN_POINT('Origin',(6.,0.,0.));
#90605=CARTESIAN_POINT('',(5.7,-4.7,-5.75583995599256E-16));
#90606=CARTESIAN_POINT('Origin',(6.,0.,0.));
#94279=UNCERTAINTY_MEASURE_WITH_UNIT(LENGTH_MEASURE(0.01),#94302,
'DISTANCE_ACCURACY_VALUE',
'Maximum model space distance between geometric entities at asserted c
onnectivities');
#94285=UNCERTAINTY_MEASURE_WITH_UNIT(LENGTH_MEASURE(0.01),#94302,
'DISTANCE_ACCURACY_VALUE',
'Maximum model space distance between geometric entities at asserted c
onnectivities');
#94295=(
GEOMETRIC_REPRESENTATION_CONTEXT(3)
GLOBAL_UNCERTAINTY_ASSIGNED_CONTEXT((#94279))
GLOBAL_UNIT_ASSIGNED_CONTEXT((#94302,#94304,#94305))
REPRESENTATION_CONTEXT('','3D')
);
#94301=(
GEOMETRIC_REPRESENTATION_CONTEXT(3)
GLOBAL_UNCERTAINTY_ASSIGNED_CONTEXT((#94285))
GLOBAL_UNIT_ASSIGNED_CONTEXT((#94302,#94304,#94305))
REPRESENTATION_CONTEXT('','3D')
);
#94302=(
LENGTH_UNIT()
NAMED_UNIT(*)
SI_UNIT(.MILLI.,.METRE.)
);
#94304=(
NAMED_UNIT(*)
PLANE_ANGLE_UNIT()
SI_UNIT($,.RADIAN.)
);
#94305=(
NAMED_UNIT(*)
SI_UNIT($,.STERADIAN.)
SOLID_ANGLE_UNIT()
);
#94315=SHAPE_DEFINITION_REPRESENTATION(#94330,#94379);
#94330=PRODUCT_DEFINITION_SHAPE('',$,#94395);
#94379=SHAPE_REPRESENTATION('',(#54858),#94295);
#94385=PRODUCT_DEFINITION_CONTEXT('part definition',#94432,'design');
#94395=PRODUCT_DEFINITION('2026-10-11-08-26-41-539',
'09_ISO_4762_M6x16_SHCS',#94410,#94385);
#94410=PRODUCT_DEFINITION_FORMATION('',$,#94443);
#94432=APPLICATION_CONTEXT(
'Core Data for Automotive Mechanical Design Process');
#94433=PRODUCT_CONTEXT('part definition',#94432,'mechanical');
#94443=PRODUCT('2026-10-11-08-26-41-539','09_ISO_4762_M6x16_SHCS',$,(#94433));
#94582=COLOUR_RGB('Black',0.12,0.14,0.17);
#94583=FILL_AREA_STYLE_COLOUR('',#94582);
#94584=FILL_AREA_STYLE('',(#94583));
#94585=SURFACE_STYLE_FILL_AREA(#94584);
#94586=SURFACE_SIDE_STYLE('',(#94585));
#94587=SURFACE_STYLE_USAGE(.BOTH.,#94586);
#94588=PRESENTATION_STYLE_ASSIGNMENT((#94587));
ENDSEC;
END-ISO-10303-21;
